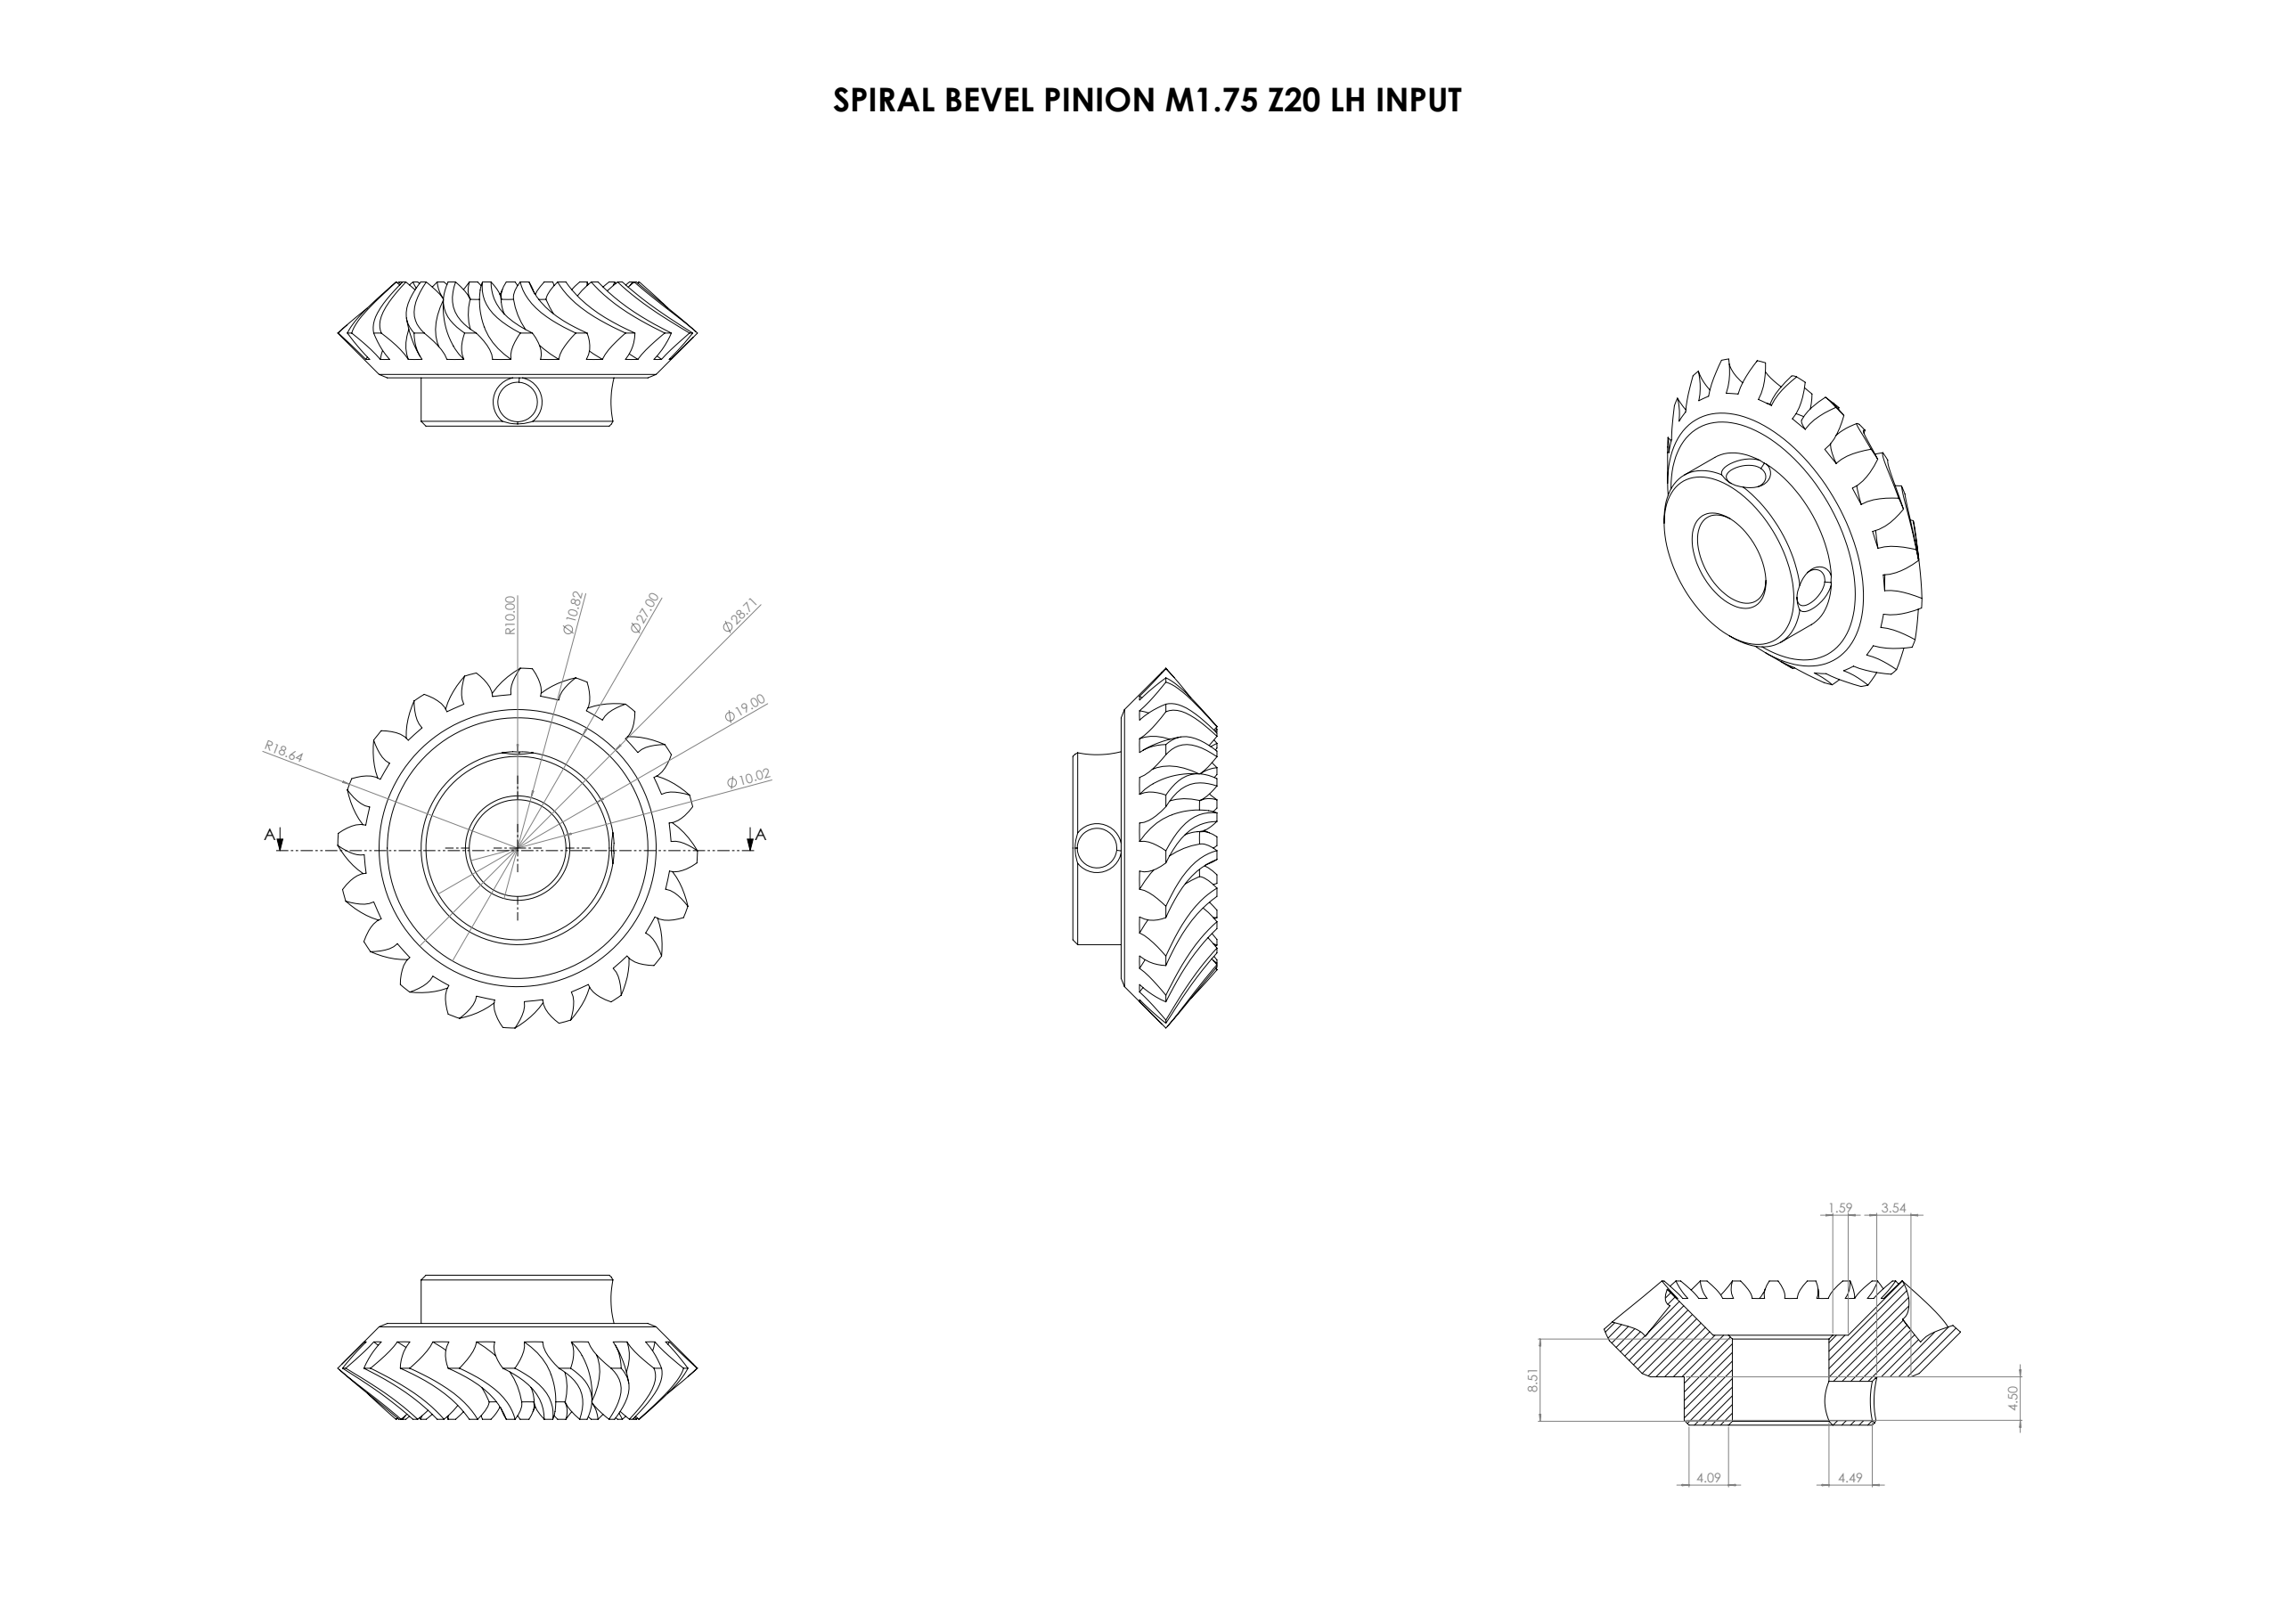
ISO-10303-21;
HEADER;
/* Generated by software containing ST-Developer
 * from STEP Tools, Inc. (www.steptools.com) 
 */

FILE_DESCRIPTION(
/* description */ (''),
/* implementation_level */ '2;1');

FILE_NAME(
/* name */ 
'03_Spiral_Bevel_Pinion_m1.75_z20_LH_Input.step',
/* time_stamp */ '2026-10-22T00:21:42-07:00',
/* author */ (''),
/* organization */ (''),
/* preprocessor_version */ 'ST-DEVELOPER v20.2',
/* originating_system */ 'Autodesk Translation Framework v15.15.0.0',
/* authorisation */ '');

FILE_SCHEMA (('AUTOMOTIVE_DESIGN { 1 0 10303 214 3 1 1 }'));
ENDSEC;

DATA;
#10=MECHANICAL_DESIGN_GEOMETRIC_PRESENTATION_REPRESENTATION('',(#206),#31638);
#184=SHAPE_REPRESENTATION_RELATIONSHIP('SRR','None',#31706,#195);
#195=ADVANCED_BREP_SHAPE_REPRESENTATION('',(#217),#31628);
#206=STYLED_ITEM('',(#31823),#217);
#217=MANIFOLD_SOLID_BREP('Spiral bevel gear',#12481);
#263=CYLINDRICAL_SURFACE('',#12805,1.);
#264=CYLINDRICAL_SURFACE('',#12808,1.);
#265=CYLINDRICAL_SURFACE('',#12810,0.205);
#266=CYLINDRICAL_SURFACE('',#12811,0.205);
#267=CYLINDRICAL_SURFACE('',#12860,0.501);
#376=CONICAL_SURFACE('',#12777,1.39267766952966,1.17809724509617);
#377=CONICAL_SURFACE('',#12781,1.63192209588552,0.785398163397448);
#378=CONICAL_SURFACE('',#12812,0.975,0.785398163397446);
#379=CONICAL_SURFACE('',#12814,1.56260147929642,0.850360450324169);
#380=CONICAL_SURFACE('',#12816,1.56260147929642,0.850360450324169);
#381=CONICAL_SURFACE('',#12818,1.56260147929642,0.850360450324169);
#382=CONICAL_SURFACE('',#12820,1.56260147929642,0.850360450324169);
#383=CONICAL_SURFACE('',#12822,1.56260147929642,0.850360450324169);
#384=CONICAL_SURFACE('',#12824,1.56260147929642,0.850360450324169);
#385=CONICAL_SURFACE('',#12826,1.56260147929642,0.850360450324169);
#386=CONICAL_SURFACE('',#12828,1.56260147929642,0.850360450324169);
#387=CONICAL_SURFACE('',#12830,1.56260147929642,0.850360450324169);
#388=CONICAL_SURFACE('',#12832,1.56260147929642,0.850360450324169);
#389=CONICAL_SURFACE('',#12834,1.56260147929642,0.850360450324169);
#390=CONICAL_SURFACE('',#12836,1.56260147929642,0.850360450324169);
#391=CONICAL_SURFACE('',#12838,1.56260147929642,0.850360450324169);
#392=CONICAL_SURFACE('',#12840,1.56260147929642,0.850360450324169);
#393=CONICAL_SURFACE('',#12842,1.56260147929642,0.850360450324169);
#394=CONICAL_SURFACE('',#12844,1.56260147929642,0.850360450324169);
#395=CONICAL_SURFACE('',#12846,1.56260147929642,0.850360450324169);
#396=CONICAL_SURFACE('',#12848,1.56260147929642,0.850360450324169);
#397=CONICAL_SURFACE('',#12850,1.56260147929642,0.850360450324169);
#398=CONICAL_SURFACE('',#12852,0.980679383410898,0.785398163397448);
#399=CONICAL_SURFACE('',#12855,1.56260147929642,0.850360450324169);
#400=CONICAL_SURFACE('',#12858,0.521,0.785398163397448);
#401=CONICAL_SURFACE('',#12862,0.521,0.785398163397451);
#501=B_SPLINE_CURVE_WITH_KNOTS('',3,(#17566,#17567,#17568,#17569,#17570,
#17571,#17572,#17573),.UNSPECIFIED.,.F.,.F.,(4,2,2,4),(0.149692773523897,
0.272438948836772,0.38754999579811,0.470116529869204),.UNSPECIFIED.);
#502=B_SPLINE_CURVE_WITH_KNOTS('',3,(#17575,#17576,#17577,#17578,#17579,
#17580,#17581),.UNSPECIFIED.,.F.,.F.,(4,3,4),(0.,0.0936389480740432,0.191756090575866),
 .UNSPECIFIED.);
#503=B_SPLINE_CURVE_WITH_KNOTS('',3,(#17583,#17584,#17585,#17586,#17587,
#17588),.UNSPECIFIED.,.F.,.F.,(4,2,4),(0.,0.200149552465016,0.391670798584888),
 .UNSPECIFIED.);
#504=B_SPLINE_CURVE_WITH_KNOTS('',3,(#17592,#17593,#17594,#17595,#17596,
#17597,#17598,#17599),.UNSPECIFIED.,.F.,.F.,(4,2,2,4),(0.0766926694683487,
0.272438948824957,0.387549995788498,0.470116529871579),.UNSPECIFIED.);
#505=B_SPLINE_CURVE_WITH_KNOTS('',3,(#17601,#17602,#17603,#17604,#17605,
#17606,#17607),.UNSPECIFIED.,.F.,.F.,(4,3,4),(0.,0.0936389480740869,0.191756090576058),
 .UNSPECIFIED.);
#506=B_SPLINE_CURVE_WITH_KNOTS('',3,(#17609,#17610,#17611,#17612,#17613,
#17614),.UNSPECIFIED.,.F.,.F.,(4,2,4),(0.,0.200149552461942,0.391670798543005),
 .UNSPECIFIED.);
#507=B_SPLINE_CURVE_WITH_KNOTS('',3,(#17618,#17619,#17620,#17621,#17622,
#17623,#17624,#17625),.UNSPECIFIED.,.F.,.F.,(4,2,2,4),(0.07669266946791,
0.272438948814009,0.387549995787584,0.470116529878316),.UNSPECIFIED.);
#508=B_SPLINE_CURVE_WITH_KNOTS('',3,(#17627,#17628,#17629,#17630,#17631,
#17632,#17633),.UNSPECIFIED.,.F.,.F.,(4,3,4),(0.,0.093638948074052,0.191756090575907),
 .UNSPECIFIED.);
#509=B_SPLINE_CURVE_WITH_KNOTS('',3,(#17635,#17636,#17637,#17638,#17639,
#17640),.UNSPECIFIED.,.F.,.F.,(4,2,4),(0.,0.200149552452443,0.391670798540186),
 .UNSPECIFIED.);
#510=B_SPLINE_CURVE_WITH_KNOTS('',3,(#17644,#17645,#17646,#17647,#17648,
#17649,#17650,#17651),.UNSPECIFIED.,.F.,.F.,(4,2,2,4),(0.0766926694699025,
0.27243894883796,0.387549995810096,0.470116529899442),.UNSPECIFIED.);
#511=B_SPLINE_CURVE_WITH_KNOTS('',3,(#17653,#17654,#17655,#17656,#17657,
#17658,#17659),.UNSPECIFIED.,.F.,.F.,(4,3,4),(0.,0.0936389480740974,0.191756090576102),
 .UNSPECIFIED.);
#512=B_SPLINE_CURVE_WITH_KNOTS('',3,(#17661,#17662,#17663,#17664,#17665,
#17666),.UNSPECIFIED.,.F.,.F.,(4,2,4),(0.,0.200149552471508,0.391670798610117),
 .UNSPECIFIED.);
#513=B_SPLINE_CURVE_WITH_KNOTS('',3,(#17670,#17671,#17672,#17673,#17674,
#17675,#17676,#17677),.UNSPECIFIED.,.F.,.F.,(4,2,2,4),(0.0766926694689824,
0.272438948828123,0.387549995794212,0.47011652987127),.UNSPECIFIED.);
#514=B_SPLINE_CURVE_WITH_KNOTS('',3,(#17679,#17680,#17681,#17682,#17683,
#17684,#17685),.UNSPECIFIED.,.F.,.F.,(4,3,4),(0.,0.0936389480740665,0.191756090575991),
 .UNSPECIFIED.);
#515=B_SPLINE_CURVE_WITH_KNOTS('',3,(#17687,#17688,#17689,#17690,#17691,
#17692),.UNSPECIFIED.,.F.,.F.,(4,2,4),(0.,0.200149552469487,0.327652992715533),
 .UNSPECIFIED.);
#516=B_SPLINE_CURVE_WITH_KNOTS('',3,(#17696,#17697,#17698,#17699,#17700,
#17701,#17702,#17703),.UNSPECIFIED.,.F.,.F.,(4,2,2,4),(0.0766926694695153,
0.272438948836664,0.387549995798075,0.47011652986564),.UNSPECIFIED.);
#517=B_SPLINE_CURVE_WITH_KNOTS('',3,(#17705,#17706,#17707,#17708,#17709,
#17710,#17711),.UNSPECIFIED.,.F.,.F.,(4,3,4),(0.,0.0936389480740678,0.191756090575965),
 .UNSPECIFIED.);
#518=B_SPLINE_CURVE_WITH_KNOTS('',3,(#17713,#17714,#17715,#17716,#17717,
#17718),.UNSPECIFIED.,.F.,.F.,(4,2,4),(0.,0.200149552470465,0.391670798620175),
 .UNSPECIFIED.);
#519=B_SPLINE_CURVE_WITH_KNOTS('',3,(#17722,#17723,#17724,#17725,#17726,
#17727,#17728,#17729),.UNSPECIFIED.,.F.,.F.,(4,2,2,4),(0.0766926694689144,
0.272438948826603,0.387549995797168,0.47011652988698),.UNSPECIFIED.);
#520=B_SPLINE_CURVE_WITH_KNOTS('',3,(#17731,#17732,#17733,#17734,#17735,
#17736,#17737),.UNSPECIFIED.,.F.,.F.,(4,3,4),(0.,0.0936389480740579,0.191756090575915),
 .UNSPECIFIED.);
#521=B_SPLINE_CURVE_WITH_KNOTS('',3,(#17739,#17740,#17741,#17742,#17743,
#17744),.UNSPECIFIED.,.F.,.F.,(4,2,4),(0.,0.200149552468106,0.391670798588367),
 .UNSPECIFIED.);
#522=B_SPLINE_CURVE_WITH_KNOTS('',3,(#17748,#17749,#17750,#17751,#17752,
#17753,#17754,#17755),.UNSPECIFIED.,.F.,.F.,(4,2,2,4),(0.0766926694722585,
0.272438948867033,0.387549995827054,0.470116529890559),.UNSPECIFIED.);
#523=B_SPLINE_CURVE_WITH_KNOTS('',3,(#17757,#17758,#17759,#17760,#17761,
#17762,#17763),.UNSPECIFIED.,.F.,.F.,(4,3,4),(0.,0.0936389480740453,0.191756090575874),
 .UNSPECIFIED.);
#524=B_SPLINE_CURVE_WITH_KNOTS('',3,(#17765,#17766,#17767,#17768,#17769,
#17770),.UNSPECIFIED.,.F.,.F.,(4,2,4),(0.,0.200149552459509,0.391670798578034),
 .UNSPECIFIED.);
#525=B_SPLINE_CURVE_WITH_KNOTS('',3,(#17774,#17775,#17776,#17777,#17778,
#17779,#17780,#17781),.UNSPECIFIED.,.F.,.F.,(4,2,2,4),(0.0766926694700454,
0.272438948841727,0.387549995804977,0.470116529879896),.UNSPECIFIED.);
#526=B_SPLINE_CURVE_WITH_KNOTS('',3,(#17783,#17784,#17785,#17786,#17787,
#17788,#17789),.UNSPECIFIED.,.F.,.F.,(4,3,4),(0.,0.0936389480740846,0.191756090576072),
 .UNSPECIFIED.);
#527=B_SPLINE_CURVE_WITH_KNOTS('',3,(#17791,#17792,#17793,#17794,#17795,
#17796),.UNSPECIFIED.,.F.,.F.,(4,2,4),(0.,0.200149552458071,0.391670798531918),
 .UNSPECIFIED.);
#528=B_SPLINE_CURVE_WITH_KNOTS('',3,(#17800,#17801,#17802,#17803,#17804,
#17805,#17806,#17807),.UNSPECIFIED.,.F.,.F.,(4,2,2,4),(0.0766926694689764,
0.272438948828007,0.387549995794164,0.470116529870617),.UNSPECIFIED.);
#529=B_SPLINE_CURVE_WITH_KNOTS('',3,(#17809,#17810,#17811,#17812,#17813,
#17814,#17815),.UNSPECIFIED.,.F.,.F.,(4,3,4),(0.,0.0936389480741051,0.191756090576146),
 .UNSPECIFIED.);
#530=B_SPLINE_CURVE_WITH_KNOTS('',3,(#17817,#17818,#17819,#17820,#17821,
#17822),.UNSPECIFIED.,.F.,.F.,(4,2,4),(0.,0.200149552457873,0.327652992693914),
 .UNSPECIFIED.);
#531=B_SPLINE_CURVE_WITH_KNOTS('',3,(#17826,#17827,#17828,#17829,#17830,
#17831,#17832,#17833),.UNSPECIFIED.,.F.,.F.,(4,2,2,4),(0.0766926694699692,
0.272438948839556,0.387549995809595,0.470116529895468),.UNSPECIFIED.);
#532=B_SPLINE_CURVE_WITH_KNOTS('',3,(#17835,#17836,#17837,#17838,#17839,
#17840,#17841),.UNSPECIFIED.,.F.,.F.,(4,3,4),(0.,0.0936389480740616,0.191756090575948),
 .UNSPECIFIED.);
#533=B_SPLINE_CURVE_WITH_KNOTS('',3,(#17843,#17844,#17845,#17846,#17847,
#17848),.UNSPECIFIED.,.F.,.F.,(4,2,4),(0.,0.200149552455358,0.391670798525636),
 .UNSPECIFIED.);
#534=B_SPLINE_CURVE_WITH_KNOTS('',3,(#17852,#17853,#17854,#17855,#17856,
#17857,#17858,#17859),.UNSPECIFIED.,.F.,.F.,(4,2,2,4),(0.0766926694698568,
0.272438948838172,0.387549995805395,0.470116529884337),.UNSPECIFIED.);
#535=B_SPLINE_CURVE_WITH_KNOTS('',3,(#17861,#17862,#17863,#17864,#17865,
#17866,#17867),.UNSPECIFIED.,.F.,.F.,(4,3,4),(0.,0.0936389480740228,0.191756090575811),
 .UNSPECIFIED.);
#536=B_SPLINE_CURVE_WITH_KNOTS('',3,(#17869,#17870,#17871,#17872,#17873,
#17874),.UNSPECIFIED.,.F.,.F.,(4,2,4),(0.,0.200149552470612,0.391670798618823),
 .UNSPECIFIED.);
#537=B_SPLINE_CURVE_WITH_KNOTS('',3,(#17878,#17879,#17880,#17881,#17882,
#17883,#17884,#17885),.UNSPECIFIED.,.F.,.F.,(4,2,2,4),(0.0766926694692372,
0.272438948831663,0.387549995799224,0.470116529873121),.UNSPECIFIED.);
#538=B_SPLINE_CURVE_WITH_KNOTS('',3,(#17887,#17888,#17889,#17890,#17891,
#17892,#17893),.UNSPECIFIED.,.F.,.F.,(4,3,4),(0.,0.0936389480740782,0.19175609057602),
 .UNSPECIFIED.);
#539=B_SPLINE_CURVE_WITH_KNOTS('',3,(#17895,#17896,#17897,#17898,#17899,
#17900),.UNSPECIFIED.,.F.,.F.,(4,2,4),(0.,0.200149552459575,0.391670798562508),
 .UNSPECIFIED.);
#540=B_SPLINE_CURVE_WITH_KNOTS('',3,(#17904,#17905,#17906,#17907,#17908,
#17909,#17910,#17911),.UNSPECIFIED.,.F.,.F.,(4,2,2,4),(0.0766926694691861,
0.272438948833637,0.387549995804666,0.470116529896578),.UNSPECIFIED.);
#541=B_SPLINE_CURVE_WITH_KNOTS('',3,(#17913,#17914,#17915,#17916,#17917,
#17918,#17919),.UNSPECIFIED.,.F.,.F.,(4,3,4),(0.,0.093638948074071,0.191756090576001),
 .UNSPECIFIED.);
#542=B_SPLINE_CURVE_WITH_KNOTS('',3,(#17921,#17922,#17923,#17924,#17925,
#17926),.UNSPECIFIED.,.F.,.F.,(4,2,4),(0.,0.20014955246592,0.39167079859368),
 .UNSPECIFIED.);
#543=B_SPLINE_CURVE_WITH_KNOTS('',3,(#17930,#17931,#17932,#17933,#17934,
#17935,#17936,#17937),.UNSPECIFIED.,.F.,.F.,(4,2,2,4),(0.0766926694700761,
0.27243894884306,0.387549995806336,0.470116529880931),.UNSPECIFIED.);
#544=B_SPLINE_CURVE_WITH_KNOTS('',3,(#17939,#17940,#17941,#17942,#17943,
#17944,#17945),.UNSPECIFIED.,.F.,.F.,(4,3,4),(0.,0.0936389480740579,0.191756090575929),
 .UNSPECIFIED.);
#545=B_SPLINE_CURVE_WITH_KNOTS('',3,(#17947,#17948,#17949,#17950,#17951,
#17952),.UNSPECIFIED.,.F.,.F.,(4,2,4),(0.,0.200149552465185,0.327652992740583),
 .UNSPECIFIED.);
#546=B_SPLINE_CURVE_WITH_KNOTS('',3,(#17956,#17957,#17958,#17959,#17960,
#17961,#17962,#17963),.UNSPECIFIED.,.F.,.F.,(4,2,2,4),(0.0766926694694027,
0.272438948835416,0.38754999579658,0.470116529865663),.UNSPECIFIED.);
#547=B_SPLINE_CURVE_WITH_KNOTS('',3,(#17965,#17966,#17967,#17968,#17969,
#17970,#17971),.UNSPECIFIED.,.F.,.F.,(4,3,4),(0.,0.0936389480740775,0.191756090576017),
 .UNSPECIFIED.);
#548=B_SPLINE_CURVE_WITH_KNOTS('',3,(#17973,#17974,#17975,#17976,#17977,
#17978),.UNSPECIFIED.,.F.,.F.,(4,2,4),(0.,0.200149552466382,0.391670798591391),
 .UNSPECIFIED.);
#549=B_SPLINE_CURVE_WITH_KNOTS('',3,(#17982,#17983,#17984,#17985,#17986,
#17987,#17988,#17989),.UNSPECIFIED.,.F.,.F.,(4,2,2,4),(0.0766926694683472,
0.272438948824933,0.387549995788448,0.470116529871442),.UNSPECIFIED.);
#550=B_SPLINE_CURVE_WITH_KNOTS('',3,(#17991,#17992,#17993,#17994,#17995,
#17996,#17997),.UNSPECIFIED.,.F.,.F.,(4,3,4),(0.,0.0936389480740692,0.19175609057597),
 .UNSPECIFIED.);
#551=B_SPLINE_CURVE_WITH_KNOTS('',3,(#17999,#18000,#18001,#18002,#18003,
#18004),.UNSPECIFIED.,.F.,.F.,(4,2,4),(0.,0.200149552469509,0.391670798593535),
 .UNSPECIFIED.);
#552=B_SPLINE_CURVE_WITH_KNOTS('',3,(#18008,#18009,#18010,#18011,#18012,
#18013,#18014,#18015),.UNSPECIFIED.,.F.,.F.,(4,2,2,4),(0.0766926694679092,
0.272438948814003,0.387549995787569,0.470116529878258),.UNSPECIFIED.);
#553=B_SPLINE_CURVE_WITH_KNOTS('',3,(#18017,#18018,#18019,#18020,#18021,
#18022,#18023),.UNSPECIFIED.,.F.,.F.,(4,3,4),(0.,0.093638948074058,0.191756090575958),
 .UNSPECIFIED.);
#554=B_SPLINE_CURVE_WITH_KNOTS('',3,(#18025,#18026,#18027,#18028,#18029,
#18030),.UNSPECIFIED.,.F.,.F.,(4,2,4),(0.,0.200149552458024,0.391670798575916),
 .UNSPECIFIED.);
#555=B_SPLINE_CURVE_WITH_KNOTS('',3,(#18034,#18035,#18036,#18037,#18038,
#18039,#18040,#18041),.UNSPECIFIED.,.F.,.F.,(4,2,2,4),(0.076692669469278,
0.272438948829378,0.387549995792969,0.47011652986107),.UNSPECIFIED.);
#556=B_SPLINE_CURVE_WITH_KNOTS('',3,(#18043,#18044,#18045,#18046,#18047,
#18048,#18049),.UNSPECIFIED.,.F.,.F.,(4,3,4),(0.,0.093638948074072,0.191756090575973),
 .UNSPECIFIED.);
#557=B_SPLINE_CURVE_WITH_KNOTS('',3,(#18051,#18052,#18053,#18054,#18055,
#18056),.UNSPECIFIED.,.F.,.F.,(4,2,4),(0.,0.200149552458622,0.391670798526984),
 .UNSPECIFIED.);
#558=B_SPLINE_CURVE_WITH_KNOTS('',3,(#18060,#18061,#18062,#18063,#18064,
#18065,#18066,#18067),.UNSPECIFIED.,.F.,.F.,(4,2,2,4),(0.0766926694689178,
0.272438948827195,0.387549995791794,0.470116529864375),.UNSPECIFIED.);
#559=B_SPLINE_CURVE_WITH_KNOTS('',3,(#18069,#18070,#18071,#18072,#18073,
#18074,#18075),.UNSPECIFIED.,.F.,.F.,(4,3,4),(0.,0.0936389480740925,0.191756090576061),
 .UNSPECIFIED.);
#560=B_SPLINE_CURVE_WITH_KNOTS('',3,(#18077,#18078,#18079,#18080,#18081,
#18082),.UNSPECIFIED.,.F.,.F.,(4,2,4),(0.,0.200149552462937,0.327652992716261),
 .UNSPECIFIED.);
#561=B_SPLINE_CURVE_WITH_KNOTS('',3,(#18085,#18086,#18087,#18088),
 .UNSPECIFIED.,.F.,.F.,(4,4),(0.076692669469509,0.149692773523897),
 .UNSPECIFIED.);
#562=B_SPLINE_CURVE_WITH_KNOTS('',3,(#18094,#18095,#18096,#18097,#18098,
#18099,#18100,#18101,#18102,#18103,#18104,#18105,#18106,#18107,#18108,#18109,
#18110,#18111,#18112,#18113,#18114,#18115,#18116,#18117,#18118,#18119,#18120,
#18121,#18122,#18123,#18124,#18125,#18126,#18127,#18128,#18129,#18130),
 .UNSPECIFIED.,.F.,.F.,(4,3,3,3,3,3,3,3,3,3,3,3,4),(0.,0.0140126898858465,
0.0198365927950119,0.0393688637311589,0.0455583406050571,0.0493231568139791,
0.0527005792494364,0.0569161964938546,0.0651768568751002,0.0683276956644967,
0.0828398890011837,0.0964479725722503,0.100882854087323),.UNSPECIFIED.);
#563=B_SPLINE_CURVE_WITH_KNOTS('',3,(#18133,#18134,#18135,#18136,#18137,
#18138,#18139,#18140,#18141,#18142,#18143,#18144,#18145,#18146,#18147,#18148,
#18149,#18150,#18151,#18152,#18153,#18154,#18155,#18156,#18157,#18158,#18159,
#18160,#18161,#18162,#18163,#18164,#18165,#18166),.UNSPECIFIED.,.F.,.F.,
(4,3,3,3,3,3,3,3,3,3,3,4),(0.,0.0110116267986798,0.0198365927950272,0.0393688637311641,
0.0455583406049715,0.0493231568143408,0.0527005792502689,0.056916196494854,
0.0651768568763584,0.0788461297337949,0.0828398890027903,0.100882854089343),
 .UNSPECIFIED.);
#564=B_SPLINE_CURVE_WITH_KNOTS('',3,(#18284,#18285,#18286,#18287,#18288,
#18289,#18290,#18291,#18292,#18293,#18294,#18295,#18296,#18297),
 .UNSPECIFIED.,.F.,.F.,(4,1,1,1,1,1,1,1,1,2,4),(-0.889886066635509,-0.843971490026765,
-0.78979558357151,-0.749163653730069,-0.681443770661001,-0.654355817433373,
-0.627267864205746,-0.600179910978118,-0.573091957750491,-0.464740144839981,
-0.44137654239973),.UNSPECIFIED.);
#565=B_SPLINE_CURVE_WITH_KNOTS('',3,(#18299,#18300,#18301,#18302,#18303,
#18304,#18305,#18306,#18307,#18308,#18309,#18310),.UNSPECIFIED.,.F.,.F.,
(4,2,2,2,2,4),(0.,0.0358257028990328,0.131952299625094,0.148884451735932,
0.157379698574708,0.16223106694039),.UNSPECIFIED.);
#566=B_SPLINE_CURVE_WITH_KNOTS('',3,(#18312,#18313,#18314,#18315),
 .UNSPECIFIED.,.F.,.F.,(4,4),(0.549999999941368,1.),.UNSPECIFIED.);
#567=B_SPLINE_CURVE_WITH_KNOTS('',3,(#18317,#18318,#18319,#18320,#18321,
#18322,#18323,#18324,#18325,#18326,#18327,#18328,#18329,#18330,#18331,#18332),
 .UNSPECIFIED.,.F.,.F.,(4,1,2,1,1,1,1,1,1,1,1,1,4),(0.310721506882948,0.387730825861464,
0.464740144839981,0.573091957750491,0.600179910978118,0.627267864205746,
0.654355817433373,0.681443770661001,0.749163653730069,0.78979558357151,
0.843971490026765,0.89814739648202,0.929489890414014),.UNSPECIFIED.);
#568=B_SPLINE_CURVE_WITH_KNOTS('',3,(#18333,#18334,#18335,#18336,#18337,
#18338,#18339,#18340,#18341,#18342,#18343,#18344,#18345,#18346,#18347,#18348,
#18349),.UNSPECIFIED.,.F.,.F.,(4,1,1,1,1,1,1,1,1,1,1,1,1,1,4),(0.929489890414014,
0.952323302937276,1.00649920939253,1.06067511584779,1.11485102230304,1.1690269287583,
1.22320283521355,1.26383476505499,1.33155464812406,1.35864260135169,1.38573055457932,
1.41281850780694,1.43990646103457,1.49408236748983,1.54825827394508),
 .UNSPECIFIED.);
#569=B_SPLINE_CURVE_WITH_KNOTS('',3,(#18351,#18352,#18353,#18354,#18355,
#18356,#18357,#18358,#18359,#18360,#18361,#18362,#18363,#18364),
 .UNSPECIFIED.,.F.,.F.,(4,2,2,2,2,2,4),(0.16223106694039,0.163967550885131,
0.171180716857468,0.182777598096348,0.205784524866042,0.262730804446443,
0.324280670363194),.UNSPECIFIED.);
#570=B_SPLINE_CURVE_WITH_KNOTS('',3,(#18365,#18366,#18367,#18368,#18369,
#18370,#18371,#18372,#18373,#18374,#18375,#18376,#18377,#18378),
 .UNSPECIFIED.,.F.,.F.,(4,1,1,1,1,1,1,1,1,1,1,4),(-1.4176032384283,-1.41281850780694,
-1.38573055457932,-1.35864260135169,-1.33155464812406,-1.26383476505499,
-1.22320283521355,-1.1690269287583,-1.11485102230304,-1.06067511584779,
-1.00649920939253,-0.969093714192518),.UNSPECIFIED.);
#571=B_SPLINE_CURVE_WITH_KNOTS('',3,(#18384,#18385,#18386,#18387,#18388,
#18389,#18390,#18391,#18392,#18393,#18394,#18395),.UNSPECIFIED.,.F.,.F.,
(4,1,1,1,1,1,1,2,4),(-1.50954599357819,-1.43295998077967,-1.38938999215504,
-1.34582000353042,-1.25868002628116,-1.21511003765654,-1.17154004903191,
-1.08440007178266,-1.06103646934241),.UNSPECIFIED.);
#572=B_SPLINE_CURVE_WITH_KNOTS('',3,(#18398,#18399,#18400,#18401,#18402,
#18403,#18404,#18405,#18406,#18407,#18408,#18409,#18410,#18411),
 .UNSPECIFIED.,.F.,.F.,(4,1,1,1,2,2,1,1,1,4),(-2.03726316537097,-2.03275764211163,
-2.01344899085789,-1.93621438584296,-1.85897978082803,-1.78151988977668,
-1.71616490683974,-1.69437991252743,-1.60723993527817,-1.58875364113519),
 .UNSPECIFIED.);
#573=B_SPLINE_CURVE_WITH_KNOTS('',3,(#18417,#18418,#18419,#18420,#18421,
#18422,#18423,#18424,#18425,#18426),.UNSPECIFIED.,.F.,.F.,(4,2,2,2,4),(0.,
0.0782721603764034,0.156544320752807,0.234729089704077,0.312913858655347),
 .UNSPECIFIED.);
#574=B_SPLINE_CURVE_WITH_KNOTS('',3,(#18427,#18428,#18429,#18430,#18431,
#18432,#18433,#18434,#18435,#18436,#18437,#18438,#18439,#18440,#18441,#18442,
#18443,#18444,#18445,#18446,#18447,#18448,#18449,#18450,#18451,#18452),
 .UNSPECIFIED.,.F.,.F.,(4,2,2,2,2,2,2,2,2,2,2,2,4),(0.312913858655347,0.391098627606618,
0.469283396557888,0.547555556934292,0.625827717310695,0.704099877687098,
0.782372038063502,0.860556807014772,0.938741575966043,1.01692634491731,
1.09511111386858,1.17338327424499,1.25165543462139),.UNSPECIFIED.);
#575=B_SPLINE_CURVE_WITH_KNOTS('',3,(#18566,#18567,#18568,#18569,#18570,
#18571,#18572,#18573,#18574,#18575,#18576,#18577),.UNSPECIFIED.,.F.,.F.,
(4,2,2,2,2,4),(0.,0.0358257028990433,0.131952299625135,0.148884451735976,
0.157379698574799,0.162231066940522),.UNSPECIFIED.);
#576=B_SPLINE_CURVE_WITH_KNOTS('',3,(#18579,#18580,#18581,#18582),
 .UNSPECIFIED.,.F.,.F.,(4,4),(0.549999999941368,1.),.UNSPECIFIED.);
#577=B_SPLINE_CURVE_WITH_KNOTS('',3,(#18584,#18585,#18586,#18587,#18588,
#18589,#18590,#18591,#18592,#18593,#18594,#18595,#18596,#18597),
 .UNSPECIFIED.,.F.,.F.,(4,1,2,1,1,1,1,1,1,1,4),(0.930381433825624,1.00739075280414,
1.08440007178266,1.17154004903191,1.21511003765654,1.25868002628116,1.34582000353042,
1.38938999215504,1.43295998077967,1.52009995802892,1.54914981735669),
 .UNSPECIFIED.);
#578=B_SPLINE_CURVE_WITH_KNOTS('',3,(#18598,#18599,#18600,#18601,#18602,
#18603,#18604,#18605,#18606,#18607,#18608,#18609,#18610,#18611,#18612,#18613,
#18614,#18615),.UNSPECIFIED.,.F.,.F.,(4,1,1,1,1,1,2,2,1,1,1,1,1,4),(1.54914981735669,
1.56366994665355,1.58545494096586,1.60723993527817,1.69437991252743,1.71616490683974,
1.78151988977668,1.85897978082803,1.93621438584296,2.01344899085789,2.03275764211163,
2.05206629336536,2.09068359587282,2.16791820088776),.UNSPECIFIED.);
#579=B_SPLINE_CURVE_WITH_KNOTS('',3,(#18616,#18617,#18618,#18619,#18620,
#18621,#18622,#18623,#18624,#18625,#18626,#18627,#18628,#18629),
 .UNSPECIFIED.,.F.,.F.,(4,2,2,2,2,2,4),(0.162231066940522,0.163967550885278,
0.171180716857662,0.182777598096494,0.205784524865831,0.262730804445425,
0.324280670361326),.UNSPECIFIED.);
#580=B_SPLINE_CURVE_WITH_KNOTS('',3,(#18633,#18634,#18635,#18636,#18637,
#18638,#18639,#18640,#18641,#18642,#18643,#18644,#18645,#18646,#18647,#18648,
#18649,#18650,#18651,#18652,#18653,#18654,#18655,#18656,#18657,#18658),
 .UNSPECIFIED.,.F.,.F.,(4,2,2,2,2,2,2,2,2,2,2,2,4),(0.,0.0782721603764034,
0.156544320752807,0.234729089704077,0.312913858655348,0.391098627606618,
0.469283396557888,0.547555556934292,0.625827717310695,0.704099877687099,
0.782372038063502,0.860556807014772,0.938741575966043),.UNSPECIFIED.);
#581=B_SPLINE_CURVE_WITH_KNOTS('',3,(#18659,#18660,#18661,#18662,#18663,
#18664,#18665,#18666,#18667,#18668),.UNSPECIFIED.,.F.,.F.,(4,2,2,2,4),(0.938741575966043,
1.01692634491731,1.09511111386858,1.17338327424499,1.25165543462139),
 .UNSPECIFIED.);
#582=B_SPLINE_CURVE_WITH_KNOTS('',3,(#18700,#18701,#18702,#18703,#18704,
#18705),.UNSPECIFIED.,.F.,.F.,(4,2,4),(0.,0.138460176945389,0.254919406868435),
 .UNSPECIFIED.);
#583=B_SPLINE_CURVE_WITH_KNOTS('',3,(#18706,#18707,#18708,#18709,#18710,
#18711),.UNSPECIFIED.,.F.,.F.,(4,2,4),(0.0638119305867456,0.434740434623819,
0.895232561311265),.UNSPECIFIED.);
#584=B_SPLINE_CURVE_WITH_KNOTS('',3,(#18712,#18713,#18714,#18715,#18716,
#18717,#18718,#18719),.UNSPECIFIED.,.F.,.F.,(4,2,2,4),(0.0746811865707125,
0.397508022614213,0.744535688298142,1.03619555646955),.UNSPECIFIED.);
#585=B_SPLINE_CURVE_WITH_KNOTS('',3,(#18746,#18747,#18748,#18749,#18750,
#18751,#18752,#18753),.UNSPECIFIED.,.F.,.F.,(4,2,2,4),(0.0544345524991837,
0.140376841744982,0.193303927754724,0.23329596220082),.UNSPECIFIED.);
#586=B_SPLINE_CURVE_WITH_KNOTS('',3,(#18754,#18755,#18756,#18757,#18758,
#18759,#18760,#18761),.UNSPECIFIED.,.F.,.F.,(4,2,2,4),(0.15440517711793,
0.43827181462838,0.790258491635714,1.12994605591353),.UNSPECIFIED.);
#587=B_SPLINE_CURVE_WITH_KNOTS('',3,(#18762,#18763,#18764,#18765,#18766,
#18767),.UNSPECIFIED.,.F.,.F.,(4,2,4),(0.0638119305867456,0.434740434623819,
0.895232561311264),.UNSPECIFIED.);
#588=B_SPLINE_CURVE_WITH_KNOTS('',3,(#18784,#18785,#18786,#18787,#18788,
#18789,#18790),.UNSPECIFIED.,.F.,.F.,(4,3,4),(0.,0.0653793053833038,0.130355487793338),
 .UNSPECIFIED.);
#589=B_SPLINE_CURVE_WITH_KNOTS('',3,(#18794,#18795,#18796,#18797,#18798,
#18799,#18800,#18801),.UNSPECIFIED.,.F.,.F.,(4,2,2,4),(0.0746811865707133,
0.397508022614224,0.744535688298146,1.0361955564692),.UNSPECIFIED.);
#590=B_SPLINE_CURVE_WITH_KNOTS('',3,(#18804,#18805,#18806,#18807,#18808,
#18809,#18810,#18811),.UNSPECIFIED.,.F.,.F.,(4,2,2,4),(0.15440517711793,
0.438271814628377,0.790258491635718,1.12994605591353),.UNSPECIFIED.);
#591=B_SPLINE_CURVE_WITH_KNOTS('',3,(#18839,#18840,#18841,#18842,#18843,
#18844),.UNSPECIFIED.,.F.,.F.,(4,2,4),(0.,0.138460176942891,0.254919406877601),
 .UNSPECIFIED.);
#592=B_SPLINE_CURVE_WITH_KNOTS('',3,(#18845,#18846,#18847,#18848,#18849,
#18850),.UNSPECIFIED.,.F.,.F.,(4,2,4),(0.0638119305867455,0.434740434623819,
0.895232561311264),.UNSPECIFIED.);
#593=B_SPLINE_CURVE_WITH_KNOTS('',3,(#18851,#18852,#18853,#18854,#18855,
#18856,#18857,#18858),.UNSPECIFIED.,.F.,.F.,(4,2,2,4),(0.0746811865707128,
0.397508022614225,0.744535688298148,1.03619555646854),.UNSPECIFIED.);
#594=B_SPLINE_CURVE_WITH_KNOTS('',3,(#18884,#18885,#18886,#18887,#18888,
#18889,#18890,#18891),.UNSPECIFIED.,.F.,.F.,(4,2,2,4),(0.0544345524999985,
0.140376841748909,0.193303927764524,0.233295962216222),.UNSPECIFIED.);
#595=B_SPLINE_CURVE_WITH_KNOTS('',3,(#18892,#18893,#18894,#18895,#18896,
#18897),.UNSPECIFIED.,.F.,.F.,(4,2,4),(0.0638119305867455,0.434740434623819,
0.895232561311264),.UNSPECIFIED.);
#596=B_SPLINE_CURVE_WITH_KNOTS('',3,(#18914,#18915,#18916,#18917,#18918,
#18919,#18920),.UNSPECIFIED.,.F.,.F.,(4,3,4),(0.,0.0653793053833002,0.130355487793372),
 .UNSPECIFIED.);
#597=B_SPLINE_CURVE_WITH_KNOTS('',3,(#18923,#18924,#18925,#18926,#18927,
#18928,#18929,#18930),.UNSPECIFIED.,.F.,.F.,(4,2,2,4),(0.154405177117932,
0.438271814628394,0.790258491635738,1.12994605591355),.UNSPECIFIED.);
#598=B_SPLINE_CURVE_WITH_KNOTS('',3,(#18958,#18959,#18960,#18961,#18962,
#18963),.UNSPECIFIED.,.F.,.F.,(4,2,4),(0.,0.138460176943918,0.254919406860805),
 .UNSPECIFIED.);
#599=B_SPLINE_CURVE_WITH_KNOTS('',3,(#18964,#18965,#18966,#18967,#18968,
#18969),.UNSPECIFIED.,.F.,.F.,(4,2,4),(0.0638119305867456,0.434740434623819,
0.895232561311265),.UNSPECIFIED.);
#600=B_SPLINE_CURVE_WITH_KNOTS('',3,(#18970,#18971,#18972,#18973,#18974,
#18975,#18976,#18977),.UNSPECIFIED.,.F.,.F.,(4,2,2,4),(0.0746811865707128,
0.397508022614222,0.744535688298131,1.03619555646937),.UNSPECIFIED.);
#601=B_SPLINE_CURVE_WITH_KNOTS('',3,(#19003,#19004,#19005,#19006,#19007,
#19008,#19009,#19010),.UNSPECIFIED.,.F.,.F.,(4,2,2,4),(0.0544345524991458,
0.140376841744735,0.193303927754458,0.233295962201587),.UNSPECIFIED.);
#602=B_SPLINE_CURVE_WITH_KNOTS('',3,(#19011,#19012,#19013,#19014,#19015,
#19016),.UNSPECIFIED.,.F.,.F.,(4,2,4),(0.0638119305867456,0.434740434623819,
0.895232561311265),.UNSPECIFIED.);
#603=B_SPLINE_CURVE_WITH_KNOTS('',3,(#19033,#19034,#19035,#19036,#19037,
#19038,#19039),.UNSPECIFIED.,.F.,.F.,(4,3,4),(0.,0.0653793053832705,0.130355487793285),
 .UNSPECIFIED.);
#604=B_SPLINE_CURVE_WITH_KNOTS('',3,(#19042,#19043,#19044,#19045,#19046,
#19047,#19048,#19049),.UNSPECIFIED.,.F.,.F.,(4,2,2,4),(0.15440517711793,
0.438271814628378,0.790258491635719,1.12994605591353),.UNSPECIFIED.);
#605=B_SPLINE_CURVE_WITH_KNOTS('',3,(#19077,#19078,#19079,#19080,#19081,
#19082),.UNSPECIFIED.,.F.,.F.,(4,2,4),(0.,0.138460176945285,0.254919406866285),
 .UNSPECIFIED.);
#606=B_SPLINE_CURVE_WITH_KNOTS('',3,(#19083,#19084,#19085,#19086,#19087,
#19088),.UNSPECIFIED.,.F.,.F.,(4,2,4),(0.0638119305867456,0.434740434623819,
0.895232561311265),.UNSPECIFIED.);
#607=B_SPLINE_CURVE_WITH_KNOTS('',3,(#19089,#19090,#19091,#19092,#19093,
#19094,#19095,#19096),.UNSPECIFIED.,.F.,.F.,(4,2,2,4),(0.0746811865707126,
0.397508022614211,0.744535688298121,1.05488349691751),.UNSPECIFIED.);
#608=B_SPLINE_CURVE_WITH_KNOTS('',3,(#19122,#19123,#19124,#19125,#19126,
#19127,#19128,#19129),.UNSPECIFIED.,.F.,.F.,(4,2,2,4),(0.0544345524985586,
0.140376841742248,0.193303927756487,0.233295962206935),.UNSPECIFIED.);
#609=B_SPLINE_CURVE_WITH_KNOTS('',3,(#19130,#19131,#19132,#19133,#19134,
#19135),.UNSPECIFIED.,.F.,.F.,(4,2,4),(0.0638119305867456,0.434740434623819,
0.895232561311265),.UNSPECIFIED.);
#610=B_SPLINE_CURVE_WITH_KNOTS('',3,(#19152,#19153,#19154,#19155,#19156,
#19157,#19158),.UNSPECIFIED.,.F.,.F.,(4,3,4),(0.,0.0653793053832869,0.130355487793285),
 .UNSPECIFIED.);
#611=B_SPLINE_CURVE_WITH_KNOTS('',3,(#19161,#19162,#19163,#19164,#19165,
#19166,#19167,#19168),.UNSPECIFIED.,.F.,.F.,(4,2,2,4),(0.0774162478443013,
0.414979417786432,0.760655521250469,1.05194916247838),.UNSPECIFIED.);
#612=B_SPLINE_CURVE_WITH_KNOTS('',3,(#19196,#19197,#19198,#19199,#19200,
#19201),.UNSPECIFIED.,.F.,.F.,(4,2,4),(0.,0.138460176945226,0.254919406867686),
 .UNSPECIFIED.);
#613=B_SPLINE_CURVE_WITH_KNOTS('',3,(#19202,#19203,#19204,#19205,#19206,
#19207),.UNSPECIFIED.,.F.,.F.,(4,2,4),(0.0638119305867456,0.434740434623819,
0.895232561311265),.UNSPECIFIED.);
#614=B_SPLINE_CURVE_WITH_KNOTS('',3,(#19208,#19209,#19210,#19211,#19212,
#19213,#19214,#19215),.UNSPECIFIED.,.F.,.F.,(4,2,2,4),(0.0746811865707126,
0.397508022614209,0.744535688298118,1.03619555646857),.UNSPECIFIED.);
#615=B_SPLINE_CURVE_WITH_KNOTS('',3,(#19241,#19242,#19243,#19244,#19245,
#19246,#19247,#19248),.UNSPECIFIED.,.F.,.F.,(4,2,2,4),(0.0544345524990915,
0.140376841744593,0.193303927757736,0.233295962205675),.UNSPECIFIED.);
#616=B_SPLINE_CURVE_WITH_KNOTS('',3,(#19249,#19250,#19251,#19252,#19253,
#19254),.UNSPECIFIED.,.F.,.F.,(4,2,4),(0.0638119305867457,0.434740434623819,
0.895232561311264),.UNSPECIFIED.);
#617=B_SPLINE_CURVE_WITH_KNOTS('',3,(#19271,#19272,#19273,#19274,#19275,
#19276,#19277),.UNSPECIFIED.,.F.,.F.,(4,3,4),(0.,0.0653793053833536,0.130355487793441),
 .UNSPECIFIED.);
#618=B_SPLINE_CURVE_WITH_KNOTS('',3,(#19280,#19281,#19282,#19283,#19284,
#19285,#19286,#19287),.UNSPECIFIED.,.F.,.F.,(4,2,2,4),(0.154405177117923,
0.438271814628353,0.790258491635649,1.1299460559134),.UNSPECIFIED.);
#619=B_SPLINE_CURVE_WITH_KNOTS('',3,(#19315,#19316,#19317,#19318,#19319,
#19320),.UNSPECIFIED.,.F.,.F.,(4,2,4),(0.,0.138460176945371,0.254919406866122),
 .UNSPECIFIED.);
#620=B_SPLINE_CURVE_WITH_KNOTS('',3,(#19321,#19322,#19323,#19324,#19325,
#19326),.UNSPECIFIED.,.F.,.F.,(4,2,4),(0.0638119305867456,0.434740434623819,
0.895232561311265),.UNSPECIFIED.);
#621=B_SPLINE_CURVE_WITH_KNOTS('',3,(#19327,#19328,#19329,#19330,#19331,
#19332,#19333,#19334),.UNSPECIFIED.,.F.,.F.,(4,2,2,4),(0.0746811865707114,
0.397508022614213,0.744535688298102,1.03619555646808),.UNSPECIFIED.);
#622=B_SPLINE_CURVE_WITH_KNOTS('',3,(#19360,#19361,#19362,#19363,#19364,
#19365,#19366,#19367),.UNSPECIFIED.,.F.,.F.,(4,2,2,4),(0.0544345524988946,
0.140376841743774,0.193303927754125,0.233295962200619),.UNSPECIFIED.);
#623=B_SPLINE_CURVE_WITH_KNOTS('',3,(#19368,#19369,#19370,#19371,#19372,
#19373),.UNSPECIFIED.,.F.,.F.,(4,2,4),(0.0638119305867456,0.434740434623819,
0.895232561311264),.UNSPECIFIED.);
#624=B_SPLINE_CURVE_WITH_KNOTS('',3,(#19390,#19391,#19392,#19393,#19394,
#19395,#19396),.UNSPECIFIED.,.F.,.F.,(4,3,4),(0.,0.0653793053832619,0.130355487793235),
 .UNSPECIFIED.);
#625=B_SPLINE_CURVE_WITH_KNOTS('',3,(#19399,#19400,#19401,#19402,#19403,
#19404,#19405,#19406),.UNSPECIFIED.,.F.,.F.,(4,2,2,4),(0.154405177117934,
0.4382718146284,0.790258491635752,1.12994605591358),.UNSPECIFIED.);
#626=B_SPLINE_CURVE_WITH_KNOTS('',3,(#19434,#19435,#19436,#19437,#19438,
#19439),.UNSPECIFIED.,.F.,.F.,(4,2,4),(0.,0.138460176943452,0.25491940687479),
 .UNSPECIFIED.);
#627=B_SPLINE_CURVE_WITH_KNOTS('',3,(#19440,#19441,#19442,#19443,#19444,
#19445),.UNSPECIFIED.,.F.,.F.,(4,2,4),(0.0638119305867456,0.434740434623819,
0.895232561311265),.UNSPECIFIED.);
#628=B_SPLINE_CURVE_WITH_KNOTS('',3,(#19446,#19447,#19448,#19449,#19450,
#19451,#19452,#19453),.UNSPECIFIED.,.F.,.F.,(4,2,2,4),(0.0746811865707127,
0.397508022614219,0.744535688298134,1.0361955564692),.UNSPECIFIED.);
#629=B_SPLINE_CURVE_WITH_KNOTS('',3,(#19479,#19480,#19481,#19482,#19483,
#19484,#19485,#19486),.UNSPECIFIED.,.F.,.F.,(4,2,2,4),(0.0544345524985935,
0.140376841742227,0.193303927751676,0.233295962196035),.UNSPECIFIED.);
#630=B_SPLINE_CURVE_WITH_KNOTS('',3,(#19487,#19488,#19489,#19490,#19491,
#19492),.UNSPECIFIED.,.F.,.F.,(4,2,4),(0.0638119305867456,0.434740434623819,
0.895232561311264),.UNSPECIFIED.);
#631=B_SPLINE_CURVE_WITH_KNOTS('',3,(#19509,#19510,#19511,#19512,#19513,
#19514,#19515),.UNSPECIFIED.,.F.,.F.,(4,3,4),(0.,0.0653793053833638,0.130355487793505),
 .UNSPECIFIED.);
#632=B_SPLINE_CURVE_WITH_KNOTS('',3,(#19518,#19519,#19520,#19521,#19522,
#19523,#19524,#19525),.UNSPECIFIED.,.F.,.F.,(4,2,2,4),(0.154405177117939,
0.438271814628415,0.790258491635773,1.12994605591359),.UNSPECIFIED.);
#633=B_SPLINE_CURVE_WITH_KNOTS('',3,(#19553,#19554,#19555,#19556,#19557,
#19558),.UNSPECIFIED.,.F.,.F.,(4,2,4),(0.,0.138460176943768,0.254919406861752),
 .UNSPECIFIED.);
#634=B_SPLINE_CURVE_WITH_KNOTS('',3,(#19559,#19560,#19561,#19562,#19563,
#19564),.UNSPECIFIED.,.F.,.F.,(4,2,4),(0.0638119305867455,0.434740434623819,
0.895232561311264),.UNSPECIFIED.);
#635=B_SPLINE_CURVE_WITH_KNOTS('',3,(#19565,#19566,#19567,#19568,#19569,
#19570,#19571,#19572),.UNSPECIFIED.,.F.,.F.,(4,2,2,4),(0.074681186570713,
0.397508022614234,0.744535688298142,1.03619555646862),.UNSPECIFIED.);
#636=B_SPLINE_CURVE_WITH_KNOTS('',3,(#19598,#19599,#19600,#19601,#19602,
#19603,#19604,#19605),.UNSPECIFIED.,.F.,.F.,(4,2,2,4),(0.0544345524996551,
0.140376841747112,0.193303927760047,0.233295962211347),.UNSPECIFIED.);
#637=B_SPLINE_CURVE_WITH_KNOTS('',3,(#19606,#19607,#19608,#19609,#19610,
#19611),.UNSPECIFIED.,.F.,.F.,(4,2,4),(0.0638119305867455,0.434740434623819,
0.895232561311264),.UNSPECIFIED.);
#638=B_SPLINE_CURVE_WITH_KNOTS('',3,(#19628,#19629,#19630,#19631,#19632,
#19633,#19634),.UNSPECIFIED.,.F.,.F.,(4,3,4),(0.,0.065379305383271,0.130355487793261),
 .UNSPECIFIED.);
#639=B_SPLINE_CURVE_WITH_KNOTS('',3,(#19637,#19638,#19639,#19640,#19641,
#19642,#19643,#19644),.UNSPECIFIED.,.F.,.F.,(4,2,2,4),(0.154405177117931,
0.43827181462838,0.790258491635724,1.12994605591354),.UNSPECIFIED.);
#640=B_SPLINE_CURVE_WITH_KNOTS('',3,(#19672,#19673,#19674,#19675,#19676,
#19677),.UNSPECIFIED.,.F.,.F.,(4,2,4),(0.,0.13846017694485,0.254919406873115),
 .UNSPECIFIED.);
#641=B_SPLINE_CURVE_WITH_KNOTS('',3,(#19678,#19679,#19680,#19681,#19682,
#19683),.UNSPECIFIED.,.F.,.F.,(4,2,4),(0.0638119305867456,0.434740434623819,
0.895232561311265),.UNSPECIFIED.);
#642=B_SPLINE_CURVE_WITH_KNOTS('',3,(#19684,#19685,#19686,#19687,#19688,
#19689,#19690,#19691),.UNSPECIFIED.,.F.,.F.,(4,2,2,4),(0.0746811865707127,
0.397508022614212,0.74453568829812,1.05488349691753),.UNSPECIFIED.);
#643=B_SPLINE_CURVE_WITH_KNOTS('',3,(#19717,#19718,#19719,#19720,#19721,
#19722,#19723,#19724),.UNSPECIFIED.,.F.,.F.,(4,2,2,4),(0.0544345524992758,
0.140376841745509,0.193303927759893,0.233295962209951),.UNSPECIFIED.);
#644=B_SPLINE_CURVE_WITH_KNOTS('',3,(#19725,#19726,#19727,#19728,#19729,
#19730),.UNSPECIFIED.,.F.,.F.,(4,2,4),(0.0638119305867456,0.434740434623819,
0.895232561311265),.UNSPECIFIED.);
#645=B_SPLINE_CURVE_WITH_KNOTS('',3,(#19747,#19748,#19749,#19750,#19751,
#19752,#19753),.UNSPECIFIED.,.F.,.F.,(4,3,4),(0.,0.0653793053833319,0.130355487793411),
 .UNSPECIFIED.);
#646=B_SPLINE_CURVE_WITH_KNOTS('',3,(#19756,#19757,#19758,#19759,#19760,
#19761,#19762,#19763),.UNSPECIFIED.,.F.,.F.,(4,2,2,4),(0.0774162478442982,
0.414979417786394,0.760655521250395,1.05194916247827),.UNSPECIFIED.);
#647=B_SPLINE_CURVE_WITH_KNOTS('',3,(#19791,#19792,#19793,#19794,#19795,
#19796),.UNSPECIFIED.,.F.,.F.,(4,2,4),(0.,0.13846017694524,0.209756131428923),
 .UNSPECIFIED.);
#648=B_SPLINE_CURVE_WITH_KNOTS('',3,(#19797,#19798,#19799,#19800,#19801,
#19802),.UNSPECIFIED.,.F.,.F.,(4,2,4),(0.0638119305867456,0.434740434623819,
0.895232561311265),.UNSPECIFIED.);
#649=B_SPLINE_CURVE_WITH_KNOTS('',3,(#19804,#19805,#19806,#19807,#19808,
#19809,#19810,#19811),.UNSPECIFIED.,.F.,.F.,(4,2,2,4),(0.0746811865707122,
0.397508022614215,0.744535688298118,1.03619555646847),.UNSPECIFIED.);
#650=B_SPLINE_CURVE_WITH_KNOTS('',3,(#19812,#19813,#19814,#19815),
 .UNSPECIFIED.,.F.,.F.,(4,4),(0.209756131428923,0.254919406867736),
 .UNSPECIFIED.);
#651=B_SPLINE_CURVE_WITH_KNOTS('',3,(#19841,#19842,#19843,#19844,#19845,
#19846,#19847,#19848),.UNSPECIFIED.,.F.,.F.,(4,2,2,4),(0.0544345524990686,
0.140376841744483,0.193303927757129,0.233295962204701),.UNSPECIFIED.);
#652=B_SPLINE_CURVE_WITH_KNOTS('',3,(#19849,#19850,#19851,#19852,#19853,
#19854),.UNSPECIFIED.,.F.,.F.,(4,2,4),(0.0638119305867457,0.434740434623819,
0.895232561311264),.UNSPECIFIED.);
#653=B_SPLINE_CURVE_WITH_KNOTS('',3,(#19871,#19872,#19873,#19874,#19875,
#19876,#19877),.UNSPECIFIED.,.F.,.F.,(4,3,4),(0.,0.0653793053833073,0.130355487793357),
 .UNSPECIFIED.);
#654=B_SPLINE_CURVE_WITH_KNOTS('',3,(#19880,#19881,#19882,#19883,#19884,
#19885,#19886,#19887),.UNSPECIFIED.,.F.,.F.,(4,2,2,4),(0.154405177117928,
0.438271814628368,0.790258491635699,1.12994605591349),.UNSPECIFIED.);
#655=B_SPLINE_CURVE_WITH_KNOTS('',3,(#19915,#19916,#19917,#19918,#19919,
#19920),.UNSPECIFIED.,.F.,.F.,(4,2,4),(0.,0.138460176945471,0.254919406864932),
 .UNSPECIFIED.);
#656=B_SPLINE_CURVE_WITH_KNOTS('',3,(#19921,#19922,#19923,#19924,#19925,
#19926),.UNSPECIFIED.,.F.,.F.,(4,2,4),(0.0638119305867457,0.434740434623819,
0.895232561311265),.UNSPECIFIED.);
#657=B_SPLINE_CURVE_WITH_KNOTS('',3,(#19927,#19928,#19929,#19930,#19931,
#19932,#19933,#19934),.UNSPECIFIED.,.F.,.F.,(4,2,2,4),(0.0746811865707118,
0.39750802261421,0.744535688298092,1.03619555646858),.UNSPECIFIED.);
#658=B_SPLINE_CURVE_WITH_KNOTS('',3,(#19960,#19961,#19962,#19963,#19964,
#19965,#19966,#19967),.UNSPECIFIED.,.F.,.F.,(4,2,2,4),(0.0544345524998506,
0.140376841748323,0.193303927766303,0.233295962218452),.UNSPECIFIED.);
#659=B_SPLINE_CURVE_WITH_KNOTS('',3,(#19968,#19969,#19970,#19971,#19972,
#19973),.UNSPECIFIED.,.F.,.F.,(4,2,4),(0.0638119305867456,0.434740434623819,
0.895232561311265),.UNSPECIFIED.);
#660=B_SPLINE_CURVE_WITH_KNOTS('',3,(#19990,#19991,#19992,#19993,#19994,
#19995,#19996),.UNSPECIFIED.,.F.,.F.,(4,3,4),(0.,0.0653793053833078,0.130355487793348),
 .UNSPECIFIED.);
#661=B_SPLINE_CURVE_WITH_KNOTS('',3,(#19999,#20000,#20001,#20002,#20003,
#20004,#20005,#20006),.UNSPECIFIED.,.F.,.F.,(4,2,2,4),(0.154405177117931,
0.438271814628383,0.790258491635722,1.12994605591352),.UNSPECIFIED.);
#662=B_SPLINE_CURVE_WITH_KNOTS('',3,(#20034,#20035,#20036,#20037,#20038,
#20039),.UNSPECIFIED.,.F.,.F.,(4,2,4),(0.,0.138460176943519,0.254919406873928),
 .UNSPECIFIED.);
#663=B_SPLINE_CURVE_WITH_KNOTS('',3,(#20040,#20041,#20042,#20043,#20044,
#20045),.UNSPECIFIED.,.F.,.F.,(4,2,4),(0.0638119305867456,0.434740434623819,
0.895232561311265),.UNSPECIFIED.);
#664=B_SPLINE_CURVE_WITH_KNOTS('',3,(#20046,#20047,#20048,#20049,#20050,
#20051,#20052,#20053),.UNSPECIFIED.,.F.,.F.,(4,2,2,4),(0.0746811865707111,
0.397508022614208,0.744535688298079,1.036195556468),.UNSPECIFIED.);
#665=B_SPLINE_CURVE_WITH_KNOTS('',3,(#20079,#20080,#20081,#20082,#20083,
#20084,#20085,#20086),.UNSPECIFIED.,.F.,.F.,(4,2,2,4),(0.0544345524985954,
0.140376841742234,0.193303927751678,0.233295962196024),.UNSPECIFIED.);
#666=B_SPLINE_CURVE_WITH_KNOTS('',3,(#20087,#20088,#20089,#20090,#20091,
#20092),.UNSPECIFIED.,.F.,.F.,(4,2,4),(0.0638119305867456,0.434740434623819,
0.895232561311264),.UNSPECIFIED.);
#667=B_SPLINE_CURVE_WITH_KNOTS('',3,(#20109,#20110,#20111,#20112,#20113,
#20114,#20115),.UNSPECIFIED.,.F.,.F.,(4,3,4),(0.,0.0653793053833565,0.130355487793492),
 .UNSPECIFIED.);
#668=B_SPLINE_CURVE_WITH_KNOTS('',3,(#20118,#20119,#20120,#20121,#20122,
#20123,#20124,#20125),.UNSPECIFIED.,.F.,.F.,(4,2,2,4),(0.15440517711794,
0.438271814628416,0.790258491635786,1.12994605591364),.UNSPECIFIED.);
#669=B_SPLINE_CURVE_WITH_KNOTS('',3,(#20153,#20154,#20155,#20156,#20157,
#20158),.UNSPECIFIED.,.F.,.F.,(4,2,4),(0.,0.138460176943852,0.254919406858792),
 .UNSPECIFIED.);
#670=B_SPLINE_CURVE_WITH_KNOTS('',3,(#20159,#20160,#20161,#20162,#20163,
#20164),.UNSPECIFIED.,.F.,.F.,(4,2,4),(0.0638119305867455,0.434740434623819,
0.895232561311264),.UNSPECIFIED.);
#671=B_SPLINE_CURVE_WITH_KNOTS('',3,(#20165,#20166,#20167,#20168,#20169,
#20170,#20171,#20172),.UNSPECIFIED.,.F.,.F.,(4,2,2,4),(0.074681186570714,
0.397508022614236,0.744535688298161,1.03619555646797),.UNSPECIFIED.);
#672=B_SPLINE_CURVE_WITH_KNOTS('',3,(#20198,#20199,#20200,#20201,#20202,
#20203,#20204,#20205),.UNSPECIFIED.,.F.,.F.,(4,2,2,4),(0.054434552499654,
0.140376841747107,0.193303927760024,0.233295962211313),.UNSPECIFIED.);
#673=B_SPLINE_CURVE_WITH_KNOTS('',3,(#20206,#20207,#20208,#20209,#20210,
#20211),.UNSPECIFIED.,.F.,.F.,(4,2,4),(0.0638119305867455,0.434740434623819,
0.895232561311264),.UNSPECIFIED.);
#674=B_SPLINE_CURVE_WITH_KNOTS('',3,(#20228,#20229,#20230,#20231,#20232,
#20233,#20234),.UNSPECIFIED.,.F.,.F.,(4,3,4),(0.,0.0653793053832257,0.130355487793195),
 .UNSPECIFIED.);
#675=B_SPLINE_CURVE_WITH_KNOTS('',3,(#20237,#20238,#20239,#20240,#20241,
#20242,#20243,#20244),.UNSPECIFIED.,.F.,.F.,(4,2,2,4),(0.154405177117938,
0.438271814628411,0.790258491635778,1.12994605591362),.UNSPECIFIED.);
#676=B_SPLINE_CURVE_WITH_KNOTS('',3,(#20272,#20273,#20274,#20275,#20276,
#20277),.UNSPECIFIED.,.F.,.F.,(4,2,4),(0.,0.138460176944659,0.254919406872703),
 .UNSPECIFIED.);
#677=B_SPLINE_CURVE_WITH_KNOTS('',3,(#20278,#20279,#20280,#20281,#20282,
#20283),.UNSPECIFIED.,.F.,.F.,(4,2,4),(0.0638119305867456,0.434740434623819,
0.895232561311265),.UNSPECIFIED.);
#678=B_SPLINE_CURVE_WITH_KNOTS('',3,(#20284,#20285,#20286,#20287,#20288,
#20289,#20290,#20291),.UNSPECIFIED.,.F.,.F.,(4,2,2,4),(0.0746811865707118,
0.397508022614199,0.7445356882981,1.05488349691747),.UNSPECIFIED.);
#679=B_SPLINE_CURVE_WITH_KNOTS('',3,(#20317,#20318,#20319,#20320,#20321,
#20322,#20323,#20324),.UNSPECIFIED.,.F.,.F.,(4,2,2,4),(0.0544345524994541,
0.140376841746265,0.193303927760631,0.2332959622117),.UNSPECIFIED.);
#680=B_SPLINE_CURVE_WITH_KNOTS('',3,(#20325,#20326,#20327,#20328,#20329,
#20330),.UNSPECIFIED.,.F.,.F.,(4,2,4),(0.0638119305867456,0.434740434623819,
0.895232561311265),.UNSPECIFIED.);
#681=B_SPLINE_CURVE_WITH_KNOTS('',3,(#20347,#20348,#20349,#20350,#20351,
#20352,#20353),.UNSPECIFIED.,.F.,.F.,(4,3,4),(0.,0.0653793053833301,0.130355487793397),
 .UNSPECIFIED.);
#682=B_SPLINE_CURVE_WITH_KNOTS('',3,(#20356,#20357,#20358,#20359,#20360,
#20361,#20362,#20363),.UNSPECIFIED.,.F.,.F.,(4,2,2,4),(0.0774162478442986,
0.414979417786383,0.760655521250363,1.05194916247819),.UNSPECIFIED.);
#683=B_SPLINE_CURVE_WITH_KNOTS('',3,(#20391,#20392,#20393,#20394,#20395,
#20396),.UNSPECIFIED.,.F.,.F.,(4,2,4),(0.,0.138460176945229,0.254919406868124),
 .UNSPECIFIED.);
#684=B_SPLINE_CURVE_WITH_KNOTS('',3,(#20397,#20398,#20399,#20400,#20401,
#20402),.UNSPECIFIED.,.F.,.F.,(4,2,4),(0.0638119305867456,0.434740434623819,
0.895232561311265),.UNSPECIFIED.);
#685=B_SPLINE_CURVE_WITH_KNOTS('',3,(#20403,#20404,#20405,#20406,#20407,
#20408,#20409,#20410),.UNSPECIFIED.,.F.,.F.,(4,2,2,4),(0.0746811865707123,
0.397508022614217,0.744535688298116,1.03619555646925),.UNSPECIFIED.);
#686=B_SPLINE_CURVE_WITH_KNOTS('',3,(#20436,#20437,#20438,#20439,#20440,
#20441,#20442,#20443),.UNSPECIFIED.,.F.,.F.,(4,2,2,4),(0.0544345524990402,
0.140376841744349,0.193303927756099,0.233295962203159),.UNSPECIFIED.);
#687=B_SPLINE_CURVE_WITH_KNOTS('',3,(#20444,#20445,#20446,#20447,#20448,
#20449),.UNSPECIFIED.,.F.,.F.,(4,2,4),(0.0638119305867457,0.434740434623819,
0.895232561311264),.UNSPECIFIED.);
#688=B_SPLINE_CURVE_WITH_KNOTS('',3,(#20466,#20467,#20468,#20469,#20470,
#20471,#20472),.UNSPECIFIED.,.F.,.F.,(4,3,4),(0.,0.0653793053833115,0.130355487793403),
 .UNSPECIFIED.);
#689=B_SPLINE_CURVE_WITH_KNOTS('',3,(#20475,#20476,#20477,#20478,#20479,
#20480,#20481,#20482),.UNSPECIFIED.,.F.,.F.,(4,2,2,4),(0.154405177117932,
0.438271814628382,0.79025849163572,1.12994605591353),.UNSPECIFIED.);
#690=B_SPLINE_CURVE_WITH_KNOTS('',3,(#20510,#20511,#20512,#20513,#20514,
#20515),.UNSPECIFIED.,.F.,.F.,(4,2,4),(0.,0.138460176945405,0.254919406862959),
 .UNSPECIFIED.);
#691=B_SPLINE_CURVE_WITH_KNOTS('',3,(#20516,#20517,#20518,#20519,#20520,
#20521),.UNSPECIFIED.,.F.,.F.,(4,2,4),(0.0638119305867455,0.434740434623819,
0.895232561311264),.UNSPECIFIED.);
#692=B_SPLINE_CURVE_WITH_KNOTS('',3,(#20522,#20523,#20524,#20525,#20526,
#20527,#20528,#20529),.UNSPECIFIED.,.F.,.F.,(4,2,2,4),(0.0746811865707101,
0.397508022614198,0.744535688298082,1.0361955564677),.UNSPECIFIED.);
#693=B_SPLINE_CURVE_WITH_KNOTS('',3,(#20555,#20556,#20557,#20558,#20559,
#20560,#20561,#20562),.UNSPECIFIED.,.F.,.F.,(4,2,2,4),(0.0544345524991343,
0.140376841744944,0.193303927755901,0.233295962204409),.UNSPECIFIED.);
#694=B_SPLINE_CURVE_WITH_KNOTS('',3,(#20563,#20564,#20565,#20566,#20567,
#20568),.UNSPECIFIED.,.F.,.F.,(4,2,4),(0.0638119305867454,0.434740434623819,
0.895232561311264),.UNSPECIFIED.);
#695=B_SPLINE_CURVE_WITH_KNOTS('',3,(#20585,#20586,#20587,#20588,#20589,
#20590,#20591),.UNSPECIFIED.,.F.,.F.,(4,3,4),(0.,0.065379305383312,0.130355487793393),
 .UNSPECIFIED.);
#696=B_SPLINE_CURVE_WITH_KNOTS('',3,(#20594,#20595,#20596,#20597,#20598,
#20599,#20600,#20601),.UNSPECIFIED.,.F.,.F.,(4,2,2,4),(0.15440517711793,
0.438271814628381,0.790258491635719,1.12994605591353),.UNSPECIFIED.);
#697=B_SPLINE_CURVE_WITH_KNOTS('',3,(#20629,#20630,#20631,#20632,#20633,
#20634),.UNSPECIFIED.,.F.,.F.,(4,2,4),(0.,0.138460176943226,0.254919406847183),
 .UNSPECIFIED.);
#698=B_SPLINE_CURVE_WITH_KNOTS('',3,(#20635,#20636,#20637,#20638,#20639,
#20640),.UNSPECIFIED.,.F.,.F.,(4,2,4),(0.0638119305867456,0.434740434623819,
0.895232561311265),.UNSPECIFIED.);
#699=B_SPLINE_CURVE_WITH_KNOTS('',3,(#20641,#20642,#20643,#20644,#20645,
#20646,#20647,#20648),.UNSPECIFIED.,.F.,.F.,(4,2,2,4),(0.0746811865707119,
0.397508022614209,0.744535688298112,1.03619555646863),.UNSPECIFIED.);
#700=B_SPLINE_CURVE_WITH_KNOTS('',3,(#20674,#20675,#20676,#20677,#20678,
#20679,#20680,#20681),.UNSPECIFIED.,.F.,.F.,(4,2,2,4),(0.0544345524993946,
0.140376841745933,0.193303927757098,0.233295962203211),.UNSPECIFIED.);
#701=B_SPLINE_CURVE_WITH_KNOTS('',3,(#20682,#20683,#20684,#20685,#20686,
#20687),.UNSPECIFIED.,.F.,.F.,(4,2,4),(0.0638119305867456,0.434740434623819,
0.895232561311264),.UNSPECIFIED.);
#702=B_SPLINE_CURVE_WITH_KNOTS('',3,(#20704,#20705,#20706,#20707,#20708,
#20709,#20710),.UNSPECIFIED.,.F.,.F.,(4,3,4),(0.,0.0653793053833217,0.130355487793375),
 .UNSPECIFIED.);
#703=B_SPLINE_CURVE_WITH_KNOTS('',3,(#20713,#20714,#20715,#20716,#20717,
#20718,#20719,#20720),.UNSPECIFIED.,.F.,.F.,(4,2,2,4),(0.154405177117935,
0.4382718146284,0.790258491635752,1.12994605591357),.UNSPECIFIED.);
#704=B_SPLINE_CURVE_WITH_KNOTS('',3,(#20748,#20749,#20750,#20751,#20752,
#20753),.UNSPECIFIED.,.F.,.F.,(4,2,4),(0.,0.138460176944331,0.254919406857816),
 .UNSPECIFIED.);
#705=B_SPLINE_CURVE_WITH_KNOTS('',3,(#20754,#20755,#20756,#20757,#20758,
#20759),.UNSPECIFIED.,.F.,.F.,(4,2,4),(0.0638119305867456,0.434740434623819,
0.895232561311265),.UNSPECIFIED.);
#706=B_SPLINE_CURVE_WITH_KNOTS('',3,(#20760,#20761,#20762,#20763,#20764,
#20765,#20766,#20767),.UNSPECIFIED.,.F.,.F.,(4,2,2,4),(0.0746811865707107,
0.397508022614195,0.744535688298062,1.03619555646822),.UNSPECIFIED.);
#707=B_SPLINE_CURVE_WITH_KNOTS('',3,(#20793,#20794,#20795,#20796,#20797,
#20798,#20799,#20800),.UNSPECIFIED.,.F.,.F.,(4,2,2,4),(0.0544345524991419,
0.140376841744898,0.193303927757274,0.233295962207447),.UNSPECIFIED.);
#708=B_SPLINE_CURVE_WITH_KNOTS('',3,(#20801,#20802,#20803,#20804,#20805,
#20806),.UNSPECIFIED.,.F.,.F.,(4,2,4),(0.0638119305867456,0.434740434623819,
0.895232561311265),.UNSPECIFIED.);
#709=B_SPLINE_CURVE_WITH_KNOTS('',3,(#20823,#20824,#20825,#20826,#20827,
#20828,#20829),.UNSPECIFIED.,.F.,.F.,(4,3,4),(0.,0.065379305383224,0.13035548779319),
 .UNSPECIFIED.);
#710=B_SPLINE_CURVE_WITH_KNOTS('',3,(#20832,#20833,#20834,#20835,#20836,
#20837,#20838,#20839),.UNSPECIFIED.,.F.,.F.,(4,2,2,4),(0.154405177117924,
0.43827181462835,0.79025849163566,1.12994605591344),.UNSPECIFIED.);
#711=B_SPLINE_CURVE_WITH_KNOTS('',3,(#20866,#20867,#20868,#20869,#20870,
#20871),.UNSPECIFIED.,.F.,.F.,(4,2,4),(0.0638119305867455,0.434740434623819,
0.895232561311264),.UNSPECIFIED.);
#712=B_SPLINE_CURVE_WITH_KNOTS('',3,(#20872,#20873,#20874,#20875,#20876,
#20877,#20878,#20879),.UNSPECIFIED.,.F.,.F.,(4,2,2,4),(0.054434552499212,
0.140376841745297,0.193303927759282,0.233295962210278),.UNSPECIFIED.);
#713=B_SPLINE_CURVE_WITH_KNOTS('',3,(#20897,#20898,#20899,#20900,#20901,
#20902),.UNSPECIFIED.,.F.,.F.,(4,2,4),(0.0638119305867455,0.434740434623819,
0.895232561311264),.UNSPECIFIED.);
#714=B_SPLINE_CURVE_WITH_KNOTS('',3,(#20903,#20904,#20905,#20906,#20907,
#20908,#20909),.UNSPECIFIED.,.F.,.F.,(4,3,4),(0.,0.0653793053832804,0.130355487793316),
 .UNSPECIFIED.);
#715=B_SPLINE_CURVE_WITH_KNOTS('',3,(#20935,#20936,#20937,#20938,#20939,
#20940,#20941,#20942),.UNSPECIFIED.,.F.,.F.,(4,2,2,4),(0.0746811865707135,
0.397508022614223,0.744535688298131,1.05488349691753),.UNSPECIFIED.);
#716=B_SPLINE_CURVE_WITH_KNOTS('',3,(#20943,#20944,#20945,#20946,#20947,
#20948),.UNSPECIFIED.,.F.,.F.,(4,2,4),(0.,0.138460176944853,0.254919406867187),
 .UNSPECIFIED.);
#717=B_SPLINE_CURVE_WITH_KNOTS('',3,(#20974,#20975,#20976,#20977,#20978,
#20979),.UNSPECIFIED.,.F.,.F.,(4,2,4),(0.0638119305867456,0.434740434623819,
0.895232561311265),.UNSPECIFIED.);
#718=B_SPLINE_CURVE_WITH_KNOTS('',3,(#20981,#20982,#20983,#20984,#20985,
#20986,#20987,#20988),.UNSPECIFIED.,.F.,.F.,(4,2,2,4),(0.0544345524992891,
0.140376841745541,0.193303927759119,0.23329596220775),.UNSPECIFIED.);
#719=B_SPLINE_CURVE_WITH_KNOTS('',3,(#20989,#20990,#20991,#20992,#20993,
#20994,#20995,#20996),.UNSPECIFIED.,.F.,.F.,(4,2,2,4),(0.0774162478442987,
0.414979417786396,0.760655521250396,1.05194916247824),.UNSPECIFIED.);
#720=B_SPLINE_CURVE_WITH_KNOTS('',3,(#21014,#21015,#21016,#21017,#21018,
#21019),.UNSPECIFIED.,.F.,.F.,(4,2,4),(0.0638119305867456,0.434740434623819,
0.895232561311265),.UNSPECIFIED.);
#721=B_SPLINE_CURVE_WITH_KNOTS('',3,(#21020,#21021,#21022,#21023,#21024,
#21025,#21026),.UNSPECIFIED.,.F.,.F.,(4,3,4),(0.,0.0653793053833094,0.13035548779333),
 .UNSPECIFIED.);
#722=B_SPLINE_CURVE_WITH_KNOTS('',3,(#21051,#21052,#21053,#21054,#21055,
#21056),.UNSPECIFIED.,.F.,.F.,(4,2,4),(0.,0.13846017694525,0.254919406867388),
 .UNSPECIFIED.);
#1206=B_SPLINE_SURFACE_WITH_KNOTS('',3,3,((#18167,#18168,#18169,#18170,
#18171,#18172,#18173,#18174,#18175,#18176,#18177,#18178,#18179,#18180,#18181,
#18182,#18183,#18184,#18185,#18186,#18187,#18188,#18189,#18190,#18191,#18192,
#18193,#18194,#18195),(#18196,#18197,#18198,#18199,#18200,#18201,#18202,
#18203,#18204,#18205,#18206,#18207,#18208,#18209,#18210,#18211,#18212,#18213,
#18214,#18215,#18216,#18217,#18218,#18219,#18220,#18221,#18222,#18223,#18224),
(#18225,#18226,#18227,#18228,#18229,#18230,#18231,#18232,#18233,#18234,
#18235,#18236,#18237,#18238,#18239,#18240,#18241,#18242,#18243,#18244,#18245,
#18246,#18247,#18248,#18249,#18250,#18251,#18252,#18253),(#18254,#18255,
#18256,#18257,#18258,#18259,#18260,#18261,#18262,#18263,#18264,#18265,#18266,
#18267,#18268,#18269,#18270,#18271,#18272,#18273,#18274,#18275,#18276,#18277,
#18278,#18279,#18280,#18281,#18282)),.UNSPECIFIED.,.F.,.T.,.F.,(4,4),(4,
1,2,1,1,1,1,1,1,1,1,1,1,1,1,1,1,1,1,1,1,1,1,1,1,4),(0.,1.),(0.310721506882948,
0.387730825861464,0.464740144839981,0.573091957750491,0.600179910978118,
0.627267864205746,0.654355817433373,0.681443770661001,0.749163653730069,
0.78979558357151,0.843971490026765,0.89814739648202,0.952323302937276,1.00649920939253,
1.06067511584779,1.11485102230304,1.1690269287583,1.22320283521355,1.26383476505499,
1.33155464812406,1.35864260135169,1.38573055457932,1.41281850780694,1.43990646103457,
1.49408236748983,1.54825827394508),.UNSPECIFIED.);
#1207=B_SPLINE_SURFACE_WITH_KNOTS('',3,3,((#18453,#18454,#18455,#18456,
#18457,#18458,#18459,#18460,#18461,#18462,#18463,#18464,#18465,#18466,#18467,
#18468,#18469,#18470,#18471,#18472,#18473,#18474,#18475,#18476,#18477,#18478,
#18479,#18480),(#18481,#18482,#18483,#18484,#18485,#18486,#18487,#18488,
#18489,#18490,#18491,#18492,#18493,#18494,#18495,#18496,#18497,#18498,#18499,
#18500,#18501,#18502,#18503,#18504,#18505,#18506,#18507,#18508),(#18509,
#18510,#18511,#18512,#18513,#18514,#18515,#18516,#18517,#18518,#18519,#18520,
#18521,#18522,#18523,#18524,#18525,#18526,#18527,#18528,#18529,#18530,#18531,
#18532,#18533,#18534,#18535,#18536),(#18537,#18538,#18539,#18540,#18541,
#18542,#18543,#18544,#18545,#18546,#18547,#18548,#18549,#18550,#18551,#18552,
#18553,#18554,#18555,#18556,#18557,#18558,#18559,#18560,#18561,#18562,#18563,
#18564)),.UNSPECIFIED.,.F.,.T.,.F.,(4,4),(4,1,2,1,1,1,1,1,1,1,1,1,1,1,1,
2,2,1,1,1,1,1,4),(0.,1.),(0.930381433825624,1.00739075280414,1.08440007178266,
1.17154004903191,1.21511003765654,1.25868002628116,1.34582000353042,1.38938999215504,
1.43295998077967,1.52009995802892,1.56366994665355,1.58545494096586,1.60723993527817,
1.69437991252743,1.71616490683974,1.78151988977668,1.85897978082803,1.93621438584296,
2.01344899085789,2.03275764211163,2.05206629336536,2.09068359587282,2.16791820088776),
 .UNSPECIFIED.);
#1208=B_SPLINE_SURFACE_WITH_KNOTS('',3,3,((#18674,#18675,#18676,#18677),
(#18678,#18679,#18680,#18681),(#18682,#18683,#18684,#18685),(#18686,#18687,
#18688,#18689),(#18690,#18691,#18692,#18693),(#18694,#18695,#18696,#18697)),
 .UNSPECIFIED.,.F.,.F.,.F.,(4,1,1,4),(4,4),(0.,0.183007073635842,0.366014147271685,
0.854033010300598),(0.0593282328972054,0.895517622296388),.UNSPECIFIED.);
#1209=B_SPLINE_SURFACE_WITH_KNOTS('',3,3,((#18720,#18721,#18722,#18723),
(#18724,#18725,#18726,#18727),(#18728,#18729,#18730,#18731),(#18732,#18733,
#18734,#18735),(#18736,#18737,#18738,#18739),(#18740,#18741,#18742,#18743)),
 .UNSPECIFIED.,.F.,.F.,.F.,(4,1,1,4),(4,4),(0.147257440457363,0.512718537404208,
0.756359268702104,1.),(0.0593287707275125,0.895619345916655),
 .UNSPECIFIED.);
#1210=B_SPLINE_SURFACE_WITH_KNOTS('',3,3,((#18768,#18769,#18770,#18771),
(#18772,#18773,#18774,#18775),(#18776,#18777,#18778,#18779),(#18780,#18781,
#18782,#18783)),.UNSPECIFIED.,.F.,.F.,.F.,(4,4),(4,4),(0.,1.),(0.0638119305867456,
0.897818181014928),.UNSPECIFIED.);
#1211=B_SPLINE_SURFACE_WITH_KNOTS('',3,3,((#18813,#18814,#18815,#18816),
(#18817,#18818,#18819,#18820),(#18821,#18822,#18823,#18824),(#18825,#18826,
#18827,#18828),(#18829,#18830,#18831,#18832),(#18833,#18834,#18835,#18836)),
 .UNSPECIFIED.,.F.,.F.,.F.,(4,1,1,4),(4,4),(0.,0.183007073635851,0.366014147271702,
0.854033010300638),(0.0593282328972055,0.895517622296396),.UNSPECIFIED.);
#1212=B_SPLINE_SURFACE_WITH_KNOTS('',3,3,((#18859,#18860,#18861,#18862),
(#18863,#18864,#18865,#18866),(#18867,#18868,#18869,#18870),(#18871,#18872,
#18873,#18874),(#18875,#18876,#18877,#18878),(#18879,#18880,#18881,#18882)),
 .UNSPECIFIED.,.F.,.F.,.F.,(4,1,1,4),(4,4),(0.147257440457364,0.512718537404208,
0.756359268702104,1.),(0.0593287707275126,0.895619345916652),
 .UNSPECIFIED.);
#1213=B_SPLINE_SURFACE_WITH_KNOTS('',3,3,((#18898,#18899,#18900,#18901),
(#18902,#18903,#18904,#18905),(#18906,#18907,#18908,#18909),(#18910,#18911,
#18912,#18913)),.UNSPECIFIED.,.F.,.F.,.F.,(4,4),(4,4),(0.,1.),(0.0638119305867453,
0.897818181014928),.UNSPECIFIED.);
#1214=B_SPLINE_SURFACE_WITH_KNOTS('',3,3,((#18932,#18933,#18934,#18935),
(#18936,#18937,#18938,#18939),(#18940,#18941,#18942,#18943),(#18944,#18945,
#18946,#18947),(#18948,#18949,#18950,#18951),(#18952,#18953,#18954,#18955)),
 .UNSPECIFIED.,.F.,.F.,.F.,(4,1,1,4),(4,4),(0.,0.183007073635844,0.366014147271687,
0.854033010300603),(0.0593282328972056,0.895517622296375),.UNSPECIFIED.);
#1215=B_SPLINE_SURFACE_WITH_KNOTS('',3,3,((#18978,#18979,#18980,#18981),
(#18982,#18983,#18984,#18985),(#18986,#18987,#18988,#18989),(#18990,#18991,
#18992,#18993),(#18994,#18995,#18996,#18997),(#18998,#18999,#19000,#19001)),
 .UNSPECIFIED.,.F.,.F.,.F.,(4,1,1,4),(4,4),(0.147257440457365,0.634538903053156,
0.817269451526578,1.),(0.0593287707275126,0.895619345916675),
 .UNSPECIFIED.);
#1216=B_SPLINE_SURFACE_WITH_KNOTS('',3,3,((#19017,#19018,#19019,#19020),
(#19021,#19022,#19023,#19024),(#19025,#19026,#19027,#19028),(#19029,#19030,
#19031,#19032)),.UNSPECIFIED.,.F.,.F.,.F.,(4,4),(4,4),(0.,1.),(0.0638119305867456,
0.897818181014929),.UNSPECIFIED.);
#1217=B_SPLINE_SURFACE_WITH_KNOTS('',3,3,((#19051,#19052,#19053,#19054),
(#19055,#19056,#19057,#19058),(#19059,#19060,#19061,#19062),(#19063,#19064,
#19065,#19066),(#19067,#19068,#19069,#19070),(#19071,#19072,#19073,#19074)),
 .UNSPECIFIED.,.F.,.F.,.F.,(4,1,1,4),(4,4),(0.,0.182864493320986,0.365728986641973,
0.853367635497937),(0.0593282328972057,0.895517622296394),.UNSPECIFIED.);
#1218=B_SPLINE_SURFACE_WITH_KNOTS('',3,3,((#19097,#19098,#19099,#19100),
(#19101,#19102,#19103,#19104),(#19105,#19106,#19107,#19108),(#19109,#19110,
#19111,#19112),(#19113,#19114,#19115,#19116),(#19117,#19118,#19119,#19120)),
 .UNSPECIFIED.,.F.,.F.,.F.,(4,1,1,4),(4,4),(0.147257440457363,0.512718537404207,
0.756359268702104,1.),(0.0593287707275127,0.895619345916678),
 .UNSPECIFIED.);
#1219=B_SPLINE_SURFACE_WITH_KNOTS('',3,3,((#19136,#19137,#19138,#19139),
(#19140,#19141,#19142,#19143),(#19144,#19145,#19146,#19147),(#19148,#19149,
#19150,#19151)),.UNSPECIFIED.,.F.,.F.,.F.,(4,4),(4,4),(0.,1.),(0.0638119305867454,
0.897818181014929),.UNSPECIFIED.);
#1220=B_SPLINE_SURFACE_WITH_KNOTS('',3,3,((#19170,#19171,#19172,#19173),
(#19174,#19175,#19176,#19177),(#19178,#19179,#19180,#19181),(#19182,#19183,
#19184,#19185),(#19186,#19187,#19188,#19189),(#19190,#19191,#19192,#19193)),
 .UNSPECIFIED.,.F.,.F.,.F.,(4,1,1,4),(4,4),(0.,0.18300707363585,0.366014147271701,
0.854033010300635),(0.0593282328972055,0.895517622296389),.UNSPECIFIED.);
#1221=B_SPLINE_SURFACE_WITH_KNOTS('',3,3,((#19216,#19217,#19218,#19219),
(#19220,#19221,#19222,#19223),(#19224,#19225,#19226,#19227),(#19228,#19229,
#19230,#19231),(#19232,#19233,#19234,#19235),(#19236,#19237,#19238,#19239)),
 .UNSPECIFIED.,.F.,.F.,.F.,(4,1,1,4),(4,4),(0.146295352012394,0.512168772578511,
0.756084386289255,1.),(0.0593287707275128,0.895619345916675),
 .UNSPECIFIED.);
#1222=B_SPLINE_SURFACE_WITH_KNOTS('',3,3,((#19255,#19256,#19257,#19258),
(#19259,#19260,#19261,#19262),(#19263,#19264,#19265,#19266),(#19267,#19268,
#19269,#19270)),.UNSPECIFIED.,.F.,.F.,.F.,(4,4),(4,4),(0.,1.),(0.0638119305867453,
0.897818181014928),.UNSPECIFIED.);
#1223=B_SPLINE_SURFACE_WITH_KNOTS('',3,3,((#19289,#19290,#19291,#19292),
(#19293,#19294,#19295,#19296),(#19297,#19298,#19299,#19300),(#19301,#19302,
#19303,#19304),(#19305,#19306,#19307,#19308),(#19309,#19310,#19311,#19312)),
 .UNSPECIFIED.,.F.,.F.,.F.,(4,1,1,4),(4,4),(0.,0.183007073635854,0.366014147271708,
0.854033010300653),(0.0593282328972056,0.895517622296374),.UNSPECIFIED.);
#1224=B_SPLINE_SURFACE_WITH_KNOTS('',3,3,((#19335,#19336,#19337,#19338),
(#19339,#19340,#19341,#19342),(#19343,#19344,#19345,#19346),(#19347,#19348,
#19349,#19350),(#19351,#19352,#19353,#19354),(#19355,#19356,#19357,#19358)),
 .UNSPECIFIED.,.F.,.F.,.F.,(4,1,1,4),(4,4),(0.147257440457363,0.512718537404207,
0.756359268702104,1.),(0.0593287707275127,0.895619345916681),
 .UNSPECIFIED.);
#1225=B_SPLINE_SURFACE_WITH_KNOTS('',3,3,((#19374,#19375,#19376,#19377),
(#19378,#19379,#19380,#19381),(#19382,#19383,#19384,#19385),(#19386,#19387,
#19388,#19389)),.UNSPECIFIED.,.F.,.F.,.F.,(4,4),(4,4),(0.,1.),(0.0638119305867453,
0.897818181014928),.UNSPECIFIED.);
#1226=B_SPLINE_SURFACE_WITH_KNOTS('',3,3,((#19408,#19409,#19410,#19411),
(#19412,#19413,#19414,#19415),(#19416,#19417,#19418,#19419),(#19420,#19421,
#19422,#19423),(#19424,#19425,#19426,#19427),(#19428,#19429,#19430,#19431)),
 .UNSPECIFIED.,.F.,.F.,.F.,(4,1,1,4),(4,4),(0.,0.183007073635845,0.36601414727169,
0.854033010300609),(0.0593282328972055,0.895517622296379),.UNSPECIFIED.);
#1227=B_SPLINE_SURFACE_WITH_KNOTS('',3,3,((#19454,#19455,#19456,#19457),
(#19458,#19459,#19460,#19461),(#19462,#19463,#19464,#19465),(#19466,#19467,
#19468,#19469),(#19470,#19471,#19472,#19473),(#19474,#19475,#19476,#19477)),
 .UNSPECIFIED.,.F.,.F.,.F.,(4,1,1,4),(4,4),(0.147257440457364,0.512718537404208,
0.756359268702104,1.),(0.0593287707275128,0.895619345916639),
 .UNSPECIFIED.);
#1228=B_SPLINE_SURFACE_WITH_KNOTS('',3,3,((#19493,#19494,#19495,#19496),
(#19497,#19498,#19499,#19500),(#19501,#19502,#19503,#19504),(#19505,#19506,
#19507,#19508)),.UNSPECIFIED.,.F.,.F.,.F.,(4,4),(4,4),(0.,1.),(0.0638119305867455,
0.897818181014928),.UNSPECIFIED.);
#1229=B_SPLINE_SURFACE_WITH_KNOTS('',3,3,((#19527,#19528,#19529,#19530),
(#19531,#19532,#19533,#19534),(#19535,#19536,#19537,#19538),(#19539,#19540,
#19541,#19542),(#19543,#19544,#19545,#19546),(#19547,#19548,#19549,#19550)),
 .UNSPECIFIED.,.F.,.F.,.F.,(4,1,1,4),(4,4),(0.,0.18300707363585,0.3660141472717,
0.854033010300634),(0.0593282328972057,0.895517622296377),.UNSPECIFIED.);
#1230=B_SPLINE_SURFACE_WITH_KNOTS('',3,3,((#19573,#19574,#19575,#19576),
(#19577,#19578,#19579,#19580),(#19581,#19582,#19583,#19584),(#19585,#19586,
#19587,#19588),(#19589,#19590,#19591,#19592),(#19593,#19594,#19595,#19596)),
 .UNSPECIFIED.,.F.,.F.,.F.,(4,1,1,4),(4,4),(0.147257440457363,0.634538903053156,
0.817269451526578,1.),(0.0593287707275124,0.895619345916661),
 .UNSPECIFIED.);
#1231=B_SPLINE_SURFACE_WITH_KNOTS('',3,3,((#19612,#19613,#19614,#19615),
(#19616,#19617,#19618,#19619),(#19620,#19621,#19622,#19623),(#19624,#19625,
#19626,#19627)),.UNSPECIFIED.,.F.,.F.,.F.,(4,4),(4,4),(0.,1.),(0.0638119305867453,
0.897818181014928),.UNSPECIFIED.);
#1232=B_SPLINE_SURFACE_WITH_KNOTS('',3,3,((#19646,#19647,#19648,#19649),
(#19650,#19651,#19652,#19653),(#19654,#19655,#19656,#19657),(#19658,#19659,
#19660,#19661),(#19662,#19663,#19664,#19665),(#19666,#19667,#19668,#19669)),
 .UNSPECIFIED.,.F.,.F.,.F.,(4,1,1,4),(4,4),(0.,0.182864493320987,0.365728986641974,
0.853367635497938),(0.0593282328972058,0.895517622296391),.UNSPECIFIED.);
#1233=B_SPLINE_SURFACE_WITH_KNOTS('',3,3,((#19692,#19693,#19694,#19695),
(#19696,#19697,#19698,#19699),(#19700,#19701,#19702,#19703),(#19704,#19705,
#19706,#19707),(#19708,#19709,#19710,#19711),(#19712,#19713,#19714,#19715)),
 .UNSPECIFIED.,.F.,.F.,.F.,(4,1,1,4),(4,4),(0.147257440457363,0.634538903053156,
0.817269451526578,1.),(0.059328770727513,0.895619345916667),
 .UNSPECIFIED.);
#1234=B_SPLINE_SURFACE_WITH_KNOTS('',3,3,((#19731,#19732,#19733,#19734),
(#19735,#19736,#19737,#19738),(#19739,#19740,#19741,#19742),(#19743,#19744,
#19745,#19746)),.UNSPECIFIED.,.F.,.F.,.F.,(4,4),(4,4),(0.,1.),(0.0638119305867456,
0.897818181014928),.UNSPECIFIED.);
#1235=B_SPLINE_SURFACE_WITH_KNOTS('',3,3,((#19765,#19766,#19767,#19768),
(#19769,#19770,#19771,#19772),(#19773,#19774,#19775,#19776),(#19777,#19778,
#19779,#19780),(#19781,#19782,#19783,#19784),(#19785,#19786,#19787,#19788)),
 .UNSPECIFIED.,.F.,.F.,.F.,(4,1,1,4),(4,4),(0.,0.183007073635851,0.366014147271702,
0.854033010300638),(0.0593282328972056,0.895517622296395),.UNSPECIFIED.);
#1236=B_SPLINE_SURFACE_WITH_KNOTS('',3,3,((#19816,#19817,#19818,#19819),
(#19820,#19821,#19822,#19823),(#19824,#19825,#19826,#19827),(#19828,#19829,
#19830,#19831),(#19832,#19833,#19834,#19835),(#19836,#19837,#19838,#19839)),
 .UNSPECIFIED.,.F.,.F.,.F.,(4,1,1,4),(4,4),(0.146295352012395,0.512168772578511,
0.756084386289256,1.),(0.0593287707275127,0.895619345916662),
 .UNSPECIFIED.);
#1237=B_SPLINE_SURFACE_WITH_KNOTS('',3,3,((#19855,#19856,#19857,#19858),
(#19859,#19860,#19861,#19862),(#19863,#19864,#19865,#19866),(#19867,#19868,
#19869,#19870)),.UNSPECIFIED.,.F.,.F.,.F.,(4,4),(4,4),(0.,1.),(0.0638119305867453,
0.897818181014928),.UNSPECIFIED.);
#1238=B_SPLINE_SURFACE_WITH_KNOTS('',3,3,((#19889,#19890,#19891,#19892),
(#19893,#19894,#19895,#19896),(#19897,#19898,#19899,#19900),(#19901,#19902,
#19903,#19904),(#19905,#19906,#19907,#19908),(#19909,#19910,#19911,#19912)),
 .UNSPECIFIED.,.F.,.F.,.F.,(4,1,1,4),(4,4),(0.,0.18300707363585,0.3660141472717,
0.854033010300633),(0.0593282328972056,0.895517622296402),.UNSPECIFIED.);
#1239=B_SPLINE_SURFACE_WITH_KNOTS('',3,3,((#19935,#19936,#19937,#19938),
(#19939,#19940,#19941,#19942),(#19943,#19944,#19945,#19946),(#19947,#19948,
#19949,#19950),(#19951,#19952,#19953,#19954),(#19955,#19956,#19957,#19958)),
 .UNSPECIFIED.,.F.,.F.,.F.,(4,1,1,4),(4,4),(0.147257440457363,0.512718537404207,
0.756359268702104,1.),(0.0593287707275125,0.895619345916659),
 .UNSPECIFIED.);
#1240=B_SPLINE_SURFACE_WITH_KNOTS('',3,3,((#19974,#19975,#19976,#19977),
(#19978,#19979,#19980,#19981),(#19982,#19983,#19984,#19985),(#19986,#19987,
#19988,#19989)),.UNSPECIFIED.,.F.,.F.,.F.,(4,4),(4,4),(0.,1.),(0.0638119305867455,
0.897818181014928),.UNSPECIFIED.);
#1241=B_SPLINE_SURFACE_WITH_KNOTS('',3,3,((#20008,#20009,#20010,#20011),
(#20012,#20013,#20014,#20015),(#20016,#20017,#20018,#20019),(#20020,#20021,
#20022,#20023),(#20024,#20025,#20026,#20027),(#20028,#20029,#20030,#20031)),
 .UNSPECIFIED.,.F.,.F.,.F.,(4,1,1,4),(4,4),(0.,0.183007073635855,0.366014147271709,
0.854033010300655),(0.0593282328972057,0.895517622296379),.UNSPECIFIED.);
#1242=B_SPLINE_SURFACE_WITH_KNOTS('',3,3,((#20054,#20055,#20056,#20057),
(#20058,#20059,#20060,#20061),(#20062,#20063,#20064,#20065),(#20066,#20067,
#20068,#20069),(#20070,#20071,#20072,#20073),(#20074,#20075,#20076,#20077)),
 .UNSPECIFIED.,.F.,.F.,.F.,(4,1,1,4),(4,4),(0.147257440457364,0.512718537404208,
0.756359268702104,1.),(0.0593287707275129,0.895619345916649),
 .UNSPECIFIED.);
#1243=B_SPLINE_SURFACE_WITH_KNOTS('',3,3,((#20093,#20094,#20095,#20096),
(#20097,#20098,#20099,#20100),(#20101,#20102,#20103,#20104),(#20105,#20106,
#20107,#20108)),.UNSPECIFIED.,.F.,.F.,.F.,(4,4),(4,4),(0.,1.),(0.0638119305867455,
0.897818181014929),.UNSPECIFIED.);
#1244=B_SPLINE_SURFACE_WITH_KNOTS('',3,3,((#20127,#20128,#20129,#20130),
(#20131,#20132,#20133,#20134),(#20135,#20136,#20137,#20138),(#20139,#20140,
#20141,#20142),(#20143,#20144,#20145,#20146),(#20147,#20148,#20149,#20150)),
 .UNSPECIFIED.,.F.,.F.,.F.,(4,1,1,4),(4,4),(0.,0.183007073635856,0.366014147271713,
0.854033010300663),(0.0593282328972055,0.895517622296378),.UNSPECIFIED.);
#1245=B_SPLINE_SURFACE_WITH_KNOTS('',3,3,((#20173,#20174,#20175,#20176),
(#20177,#20178,#20179,#20180),(#20181,#20182,#20183,#20184),(#20185,#20186,
#20187,#20188),(#20189,#20190,#20191,#20192),(#20193,#20194,#20195,#20196)),
 .UNSPECIFIED.,.F.,.F.,.F.,(4,1,1,4),(4,4),(0.147257440457363,0.512718537404207,
0.756359268702104,1.),(0.0593287707275125,0.895619345916676),
 .UNSPECIFIED.);
#1246=B_SPLINE_SURFACE_WITH_KNOTS('',3,3,((#20212,#20213,#20214,#20215),
(#20216,#20217,#20218,#20219),(#20220,#20221,#20222,#20223),(#20224,#20225,
#20226,#20227)),.UNSPECIFIED.,.F.,.F.,.F.,(4,4),(4,4),(0.,1.),(0.0638119305867453,
0.897818181014928),.UNSPECIFIED.);
#1247=B_SPLINE_SURFACE_WITH_KNOTS('',3,3,((#20246,#20247,#20248,#20249),
(#20250,#20251,#20252,#20253),(#20254,#20255,#20256,#20257),(#20258,#20259,
#20260,#20261),(#20262,#20263,#20264,#20265),(#20266,#20267,#20268,#20269)),
 .UNSPECIFIED.,.F.,.F.,.F.,(4,1,1,4),(4,4),(0.,0.243819324427982,0.487638648855963,
0.853367635497936),(0.0593282328972057,0.895517622296394),.UNSPECIFIED.);
#1248=B_SPLINE_SURFACE_WITH_KNOTS('',3,3,((#20292,#20293,#20294,#20295),
(#20296,#20297,#20298,#20299),(#20300,#20301,#20302,#20303),(#20304,#20305,
#20306,#20307),(#20308,#20309,#20310,#20311),(#20312,#20313,#20314,#20315)),
 .UNSPECIFIED.,.F.,.F.,.F.,(4,1,1,4),(4,4),(0.147257440457363,0.512718537404207,
0.756359268702104,1.),(0.0593287707275129,0.895619345916666),
 .UNSPECIFIED.);
#1249=B_SPLINE_SURFACE_WITH_KNOTS('',3,3,((#20331,#20332,#20333,#20334),
(#20335,#20336,#20337,#20338),(#20339,#20340,#20341,#20342),(#20343,#20344,
#20345,#20346)),.UNSPECIFIED.,.F.,.F.,.F.,(4,4),(4,4),(0.,1.),(0.0638119305867456,
0.897818181014929),.UNSPECIFIED.);
#1250=B_SPLINE_SURFACE_WITH_KNOTS('',3,3,((#20365,#20366,#20367,#20368),
(#20369,#20370,#20371,#20372),(#20373,#20374,#20375,#20376),(#20377,#20378,
#20379,#20380),(#20381,#20382,#20383,#20384),(#20385,#20386,#20387,#20388)),
 .UNSPECIFIED.,.F.,.F.,.F.,(4,1,1,4),(4,4),(0.,0.183007073635844,0.366014147271688,
0.854033010300606),(0.0593282328972055,0.895517622296384),.UNSPECIFIED.);
#1251=B_SPLINE_SURFACE_WITH_KNOTS('',3,3,((#20411,#20412,#20413,#20414),
(#20415,#20416,#20417,#20418),(#20419,#20420,#20421,#20422),(#20423,#20424,
#20425,#20426),(#20427,#20428,#20429,#20430),(#20431,#20432,#20433,#20434)),
 .UNSPECIFIED.,.F.,.F.,.F.,(4,1,1,4),(4,4),(0.146295352012395,0.634126579433884,
0.817063289716942,1.),(0.0593287707275129,0.895619345916667),
 .UNSPECIFIED.);
#1252=B_SPLINE_SURFACE_WITH_KNOTS('',3,3,((#20450,#20451,#20452,#20453),
(#20454,#20455,#20456,#20457),(#20458,#20459,#20460,#20461),(#20462,#20463,
#20464,#20465)),.UNSPECIFIED.,.F.,.F.,.F.,(4,4),(4,4),(0.,1.),(0.0638119305867452,
0.897818181014929),.UNSPECIFIED.);
#1253=B_SPLINE_SURFACE_WITH_KNOTS('',3,3,((#20484,#20485,#20486,#20487),
(#20488,#20489,#20490,#20491),(#20492,#20493,#20494,#20495),(#20496,#20497,
#20498,#20499),(#20500,#20501,#20502,#20503),(#20504,#20505,#20506,#20507)),
 .UNSPECIFIED.,.F.,.F.,.F.,(4,1,1,4),(4,4),(0.,0.183007073635857,0.366014147271714,
0.854033010300667),(0.0593282328972057,0.895517622296367),.UNSPECIFIED.);
#1254=B_SPLINE_SURFACE_WITH_KNOTS('',3,3,((#20530,#20531,#20532,#20533),
(#20534,#20535,#20536,#20537),(#20538,#20539,#20540,#20541),(#20542,#20543,
#20544,#20545),(#20546,#20547,#20548,#20549),(#20550,#20551,#20552,#20553)),
 .UNSPECIFIED.,.F.,.F.,.F.,(4,1,1,4),(4,4),(0.147257440457363,0.512718537404208,
0.756359268702104,1.),(0.0593287707275124,0.89561934591667),
 .UNSPECIFIED.);
#1255=B_SPLINE_SURFACE_WITH_KNOTS('',3,3,((#20569,#20570,#20571,#20572),
(#20573,#20574,#20575,#20576),(#20577,#20578,#20579,#20580),(#20581,#20582,
#20583,#20584)),.UNSPECIFIED.,.F.,.F.,.F.,(4,4),(4,4),(0.,1.),(0.063811930586745,
0.897818181014928),.UNSPECIFIED.);
#1256=B_SPLINE_SURFACE_WITH_KNOTS('',3,3,((#20603,#20604,#20605,#20606),
(#20607,#20608,#20609,#20610),(#20611,#20612,#20613,#20614),(#20615,#20616,
#20617,#20618),(#20619,#20620,#20621,#20622),(#20623,#20624,#20625,#20626)),
 .UNSPECIFIED.,.F.,.F.,.F.,(4,1,1,4),(4,4),(0.,0.18300707363585,0.3660141472717,
0.854033010300632),(0.0593282328972055,0.895517622296395),.UNSPECIFIED.);
#1257=B_SPLINE_SURFACE_WITH_KNOTS('',3,3,((#20649,#20650,#20651,#20652),
(#20653,#20654,#20655,#20656),(#20657,#20658,#20659,#20660),(#20661,#20662,
#20663,#20664),(#20665,#20666,#20667,#20668),(#20669,#20670,#20671,#20672)),
 .UNSPECIFIED.,.F.,.F.,.F.,(4,1,1,4),(4,4),(0.147257440457364,0.634538903053156,
0.817269451526578,1.),(0.0593287707275127,0.895619345916657),
 .UNSPECIFIED.);
#1258=B_SPLINE_SURFACE_WITH_KNOTS('',3,3,((#20688,#20689,#20690,#20691),
(#20692,#20693,#20694,#20695),(#20696,#20697,#20698,#20699),(#20700,#20701,
#20702,#20703)),.UNSPECIFIED.,.F.,.F.,.F.,(4,4),(4,4),(0.,1.),(0.0638119305867455,
0.897818181014928),.UNSPECIFIED.);
#1259=B_SPLINE_SURFACE_WITH_KNOTS('',3,3,((#20722,#20723,#20724,#20725),
(#20726,#20727,#20728,#20729),(#20730,#20731,#20732,#20733),(#20734,#20735,
#20736,#20737),(#20738,#20739,#20740,#20741),(#20742,#20743,#20744,#20745)),
 .UNSPECIFIED.,.F.,.F.,.F.,(4,1,1,4),(4,4),(0.,0.183007073635853,0.366014147271705,
0.854033010300645),(0.0593282328972057,0.895517622296384),.UNSPECIFIED.);
#1260=B_SPLINE_SURFACE_WITH_KNOTS('',3,3,((#20768,#20769,#20770,#20771),
(#20772,#20773,#20774,#20775),(#20776,#20777,#20778,#20779),(#20780,#20781,
#20782,#20783),(#20784,#20785,#20786,#20787),(#20788,#20789,#20790,#20791)),
 .UNSPECIFIED.,.F.,.F.,.F.,(4,1,1,4),(4,4),(0.147257440457364,0.512718537404208,
0.756359268702104,1.),(0.0593287707275128,0.895619345916678),
 .UNSPECIFIED.);
#1261=B_SPLINE_SURFACE_WITH_KNOTS('',3,3,((#20807,#20808,#20809,#20810),
(#20811,#20812,#20813,#20814),(#20815,#20816,#20817,#20818),(#20819,#20820,
#20821,#20822)),.UNSPECIFIED.,.F.,.F.,.F.,(4,4),(4,4),(0.,1.),(0.0638119305867456,
0.897818181014929),.UNSPECIFIED.);
#1262=B_SPLINE_SURFACE_WITH_KNOTS('',3,3,((#20841,#20842,#20843,#20844),
(#20845,#20846,#20847,#20848),(#20849,#20850,#20851,#20852),(#20853,#20854,
#20855,#20856),(#20857,#20858,#20859,#20860),(#20861,#20862,#20863,#20864)),
 .UNSPECIFIED.,.F.,.F.,.F.,(4,1,1,4),(4,4),(0.147257440457363,0.634538903053156,
0.817269451526578,1.),(0.0593287707275126,0.895619345916645),
 .UNSPECIFIED.);
#1263=B_SPLINE_SURFACE_WITH_KNOTS('',3,3,((#20880,#20881,#20882,#20883),
(#20884,#20885,#20886,#20887),(#20888,#20889,#20890,#20891),(#20892,#20893,
#20894,#20895)),.UNSPECIFIED.,.F.,.F.,.F.,(4,4),(4,4),(0.,1.),(0.0638119305867452,
0.897818181014928),.UNSPECIFIED.);
#1264=B_SPLINE_SURFACE_WITH_KNOTS('',3,3,((#20910,#20911,#20912,#20913),
(#20914,#20915,#20916,#20917),(#20918,#20919,#20920,#20921),(#20922,#20923,
#20924,#20925),(#20926,#20927,#20928,#20929),(#20930,#20931,#20932,#20933)),
 .UNSPECIFIED.,.F.,.F.,.F.,(4,1,1,4),(4,4),(0.,0.243819324427982,0.487638648855964,
0.853367635497937),(0.0593282328972056,0.895517622296376),.UNSPECIFIED.);
#1265=B_SPLINE_SURFACE_WITH_KNOTS('',3,3,((#20949,#20950,#20951,#20952),
(#20953,#20954,#20955,#20956),(#20957,#20958,#20959,#20960),(#20961,#20962,
#20963,#20964),(#20965,#20966,#20967,#20968),(#20969,#20970,#20971,#20972)),
 .UNSPECIFIED.,.F.,.F.,.F.,(4,1,1,4),(4,4),(0.146295352012396,0.634126579433884,
0.817063289716942,1.),(0.059328770727513,0.895619345916653),
 .UNSPECIFIED.);
#1266=B_SPLINE_SURFACE_WITH_KNOTS('',3,3,((#20997,#20998,#20999,#21000),
(#21001,#21002,#21003,#21004),(#21005,#21006,#21007,#21008),(#21009,#21010,
#21011,#21012)),.UNSPECIFIED.,.F.,.F.,.F.,(4,4),(4,4),(0.,1.),(0.0638119305867454,
0.897818181014928),.UNSPECIFIED.);
#1267=B_SPLINE_SURFACE_WITH_KNOTS('',3,3,((#21027,#21028,#21029,#21030),
(#21031,#21032,#21033,#21034),(#21035,#21036,#21037,#21038),(#21039,#21040,
#21041,#21042),(#21043,#21044,#21045,#21046),(#21047,#21048,#21049,#21050)),
 .UNSPECIFIED.,.F.,.F.,.F.,(4,1,1,4),(4,4),(0.,0.183007073635845,0.366014147271691,
0.854033010300612),(0.0593282328972056,0.89551762229639),.UNSPECIFIED.);
#1360=FACE_BOUND('',#2665,.T.);
#1361=FACE_BOUND('',#2755,.T.);
#1362=FACE_BOUND('',#2758,.T.);
#1363=FACE_BOUND('',#2759,.T.);
#1364=FACE_BOUND('',#2762,.T.);
#1457=CIRCLE('',#12778,1.35);
#1458=CIRCLE('',#12779,1.43535533905933);
#1459=CIRCLE('',#12780,1.43535533905933);
#1460=CIRCLE('',#12782,1.86384419177103);
#1461=CIRCLE('',#12783,1.86384419177103);
#1462=CIRCLE('',#12784,1.86384419177103);
#1463=CIRCLE('',#12785,1.86384419177103);
#1464=CIRCLE('',#12786,1.86384419177103);
#1465=CIRCLE('',#12787,1.86384419177103);
#1466=CIRCLE('',#12788,1.86384419177103);
#1467=CIRCLE('',#12789,1.86384419177103);
#1468=CIRCLE('',#12790,1.86384419177103);
#1469=CIRCLE('',#12791,1.86384419177103);
#1470=CIRCLE('',#12792,1.86384419177103);
#1471=CIRCLE('',#12793,1.86384419177103);
#1472=CIRCLE('',#12794,1.86384419177103);
#1473=CIRCLE('',#12795,1.86384419177103);
#1474=CIRCLE('',#12796,1.86384419177103);
#1475=CIRCLE('',#12797,1.86384419177103);
#1476=CIRCLE('',#12798,1.86384419177103);
#1477=CIRCLE('',#12799,1.86384419177103);
#1478=CIRCLE('',#12800,1.86384419177103);
#1479=CIRCLE('',#12801,1.86384419177103);
#1480=CIRCLE('',#12803,1.);
#1481=CIRCLE('',#12804,1.);
#1482=CIRCLE('',#12806,1.);
#1483=CIRCLE('',#12807,1.);
#1484=CIRCLE('',#12809,1.);
#1485=CIRCLE('',#12813,0.95);
#1486=CIRCLE('',#12815,1.2613587668218);
#1487=CIRCLE('',#12817,1.2613587668218);
#1488=CIRCLE('',#12819,1.2613587668218);
#1489=CIRCLE('',#12821,1.2613587668218);
#1490=CIRCLE('',#12823,1.2613587668218);
#1491=CIRCLE('',#12825,1.2613587668218);
#1492=CIRCLE('',#12827,1.2613587668218);
#1493=CIRCLE('',#12829,1.2613587668218);
#1494=CIRCLE('',#12831,1.2613587668218);
#1495=CIRCLE('',#12833,1.2613587668218);
#1496=CIRCLE('',#12835,1.2613587668218);
#1497=CIRCLE('',#12837,1.2613587668218);
#1498=CIRCLE('',#12839,1.2613587668218);
#1499=CIRCLE('',#12841,1.2613587668218);
#1500=CIRCLE('',#12843,1.2613587668218);
#1501=CIRCLE('',#12845,1.2613587668218);
#1502=CIRCLE('',#12847,1.2613587668218);
#1503=CIRCLE('',#12849,1.2613587668218);
#1504=CIRCLE('',#12851,1.2613587668218);
#1505=CIRCLE('',#12853,0.7);
#1506=CIRCLE('',#12854,1.2613587668218);
#1507=CIRCLE('',#12857,0.541);
#1508=CIRCLE('',#12859,0.501);
#1509=CIRCLE('',#12861,0.501);
#1510=CIRCLE('',#12863,0.541);
#1948=FACE_OUTER_BOUND('',#2662,.T.);
#1949=FACE_OUTER_BOUND('',#2663,.T.);
#1950=FACE_OUTER_BOUND('',#2664,.T.);
#1951=FACE_OUTER_BOUND('',#2666,.T.);
#1952=FACE_OUTER_BOUND('',#2667,.T.);
#1953=FACE_OUTER_BOUND('',#2668,.T.);
#1954=FACE_OUTER_BOUND('',#2669,.T.);
#1955=FACE_OUTER_BOUND('',#2670,.T.);
#1956=FACE_OUTER_BOUND('',#2671,.T.);
#1957=FACE_OUTER_BOUND('',#2672,.T.);
#1958=FACE_OUTER_BOUND('',#2673,.T.);
#1959=FACE_OUTER_BOUND('',#2674,.T.);
#1960=FACE_OUTER_BOUND('',#2675,.T.);
#1961=FACE_OUTER_BOUND('',#2676,.T.);
#1962=FACE_OUTER_BOUND('',#2677,.T.);
#1963=FACE_OUTER_BOUND('',#2678,.T.);
#1964=FACE_OUTER_BOUND('',#2679,.T.);
#1965=FACE_OUTER_BOUND('',#2680,.T.);
#1966=FACE_OUTER_BOUND('',#2681,.T.);
#1967=FACE_OUTER_BOUND('',#2682,.T.);
#1968=FACE_OUTER_BOUND('',#2683,.T.);
#1969=FACE_OUTER_BOUND('',#2684,.T.);
#1970=FACE_OUTER_BOUND('',#2685,.T.);
#1971=FACE_OUTER_BOUND('',#2686,.T.);
#1972=FACE_OUTER_BOUND('',#2687,.T.);
#1973=FACE_OUTER_BOUND('',#2688,.T.);
#1974=FACE_OUTER_BOUND('',#2689,.T.);
#1975=FACE_OUTER_BOUND('',#2690,.T.);
#1976=FACE_OUTER_BOUND('',#2691,.T.);
#1977=FACE_OUTER_BOUND('',#2692,.T.);
#1978=FACE_OUTER_BOUND('',#2693,.T.);
#1979=FACE_OUTER_BOUND('',#2694,.T.);
#1980=FACE_OUTER_BOUND('',#2695,.T.);
#1981=FACE_OUTER_BOUND('',#2696,.T.);
#1982=FACE_OUTER_BOUND('',#2697,.T.);
#1983=FACE_OUTER_BOUND('',#2698,.T.);
#1984=FACE_OUTER_BOUND('',#2699,.T.);
#1985=FACE_OUTER_BOUND('',#2700,.T.);
#1986=FACE_OUTER_BOUND('',#2701,.T.);
#1987=FACE_OUTER_BOUND('',#2702,.T.);
#1988=FACE_OUTER_BOUND('',#2703,.T.);
#1989=FACE_OUTER_BOUND('',#2704,.T.);
#1990=FACE_OUTER_BOUND('',#2705,.T.);
#1991=FACE_OUTER_BOUND('',#2706,.T.);
#1992=FACE_OUTER_BOUND('',#2707,.T.);
#1993=FACE_OUTER_BOUND('',#2708,.T.);
#1994=FACE_OUTER_BOUND('',#2709,.T.);
#1995=FACE_OUTER_BOUND('',#2710,.T.);
#1996=FACE_OUTER_BOUND('',#2711,.T.);
#1997=FACE_OUTER_BOUND('',#2712,.T.);
#1998=FACE_OUTER_BOUND('',#2713,.T.);
#1999=FACE_OUTER_BOUND('',#2714,.T.);
#2000=FACE_OUTER_BOUND('',#2715,.T.);
#2001=FACE_OUTER_BOUND('',#2716,.T.);
#2002=FACE_OUTER_BOUND('',#2717,.T.);
#2003=FACE_OUTER_BOUND('',#2718,.T.);
#2004=FACE_OUTER_BOUND('',#2719,.T.);
#2005=FACE_OUTER_BOUND('',#2720,.T.);
#2006=FACE_OUTER_BOUND('',#2721,.T.);
#2007=FACE_OUTER_BOUND('',#2722,.T.);
#2008=FACE_OUTER_BOUND('',#2723,.T.);
#2009=FACE_OUTER_BOUND('',#2724,.T.);
#2010=FACE_OUTER_BOUND('',#2725,.T.);
#2011=FACE_OUTER_BOUND('',#2726,.T.);
#2012=FACE_OUTER_BOUND('',#2727,.T.);
#2013=FACE_OUTER_BOUND('',#2728,.T.);
#2014=FACE_OUTER_BOUND('',#2729,.T.);
#2015=FACE_OUTER_BOUND('',#2730,.T.);
#2016=FACE_OUTER_BOUND('',#2731,.T.);
#2017=FACE_OUTER_BOUND('',#2732,.T.);
#2018=FACE_OUTER_BOUND('',#2733,.T.);
#2019=FACE_OUTER_BOUND('',#2734,.T.);
#2020=FACE_OUTER_BOUND('',#2735,.T.);
#2021=FACE_OUTER_BOUND('',#2736,.T.);
#2022=FACE_OUTER_BOUND('',#2737,.T.);
#2023=FACE_OUTER_BOUND('',#2738,.T.);
#2024=FACE_OUTER_BOUND('',#2739,.T.);
#2025=FACE_OUTER_BOUND('',#2740,.T.);
#2026=FACE_OUTER_BOUND('',#2741,.T.);
#2027=FACE_OUTER_BOUND('',#2742,.T.);
#2028=FACE_OUTER_BOUND('',#2743,.T.);
#2029=FACE_OUTER_BOUND('',#2744,.T.);
#2030=FACE_OUTER_BOUND('',#2745,.T.);
#2031=FACE_OUTER_BOUND('',#2746,.T.);
#2032=FACE_OUTER_BOUND('',#2747,.T.);
#2033=FACE_OUTER_BOUND('',#2748,.T.);
#2034=FACE_OUTER_BOUND('',#2749,.T.);
#2035=FACE_OUTER_BOUND('',#2750,.T.);
#2036=FACE_OUTER_BOUND('',#2751,.T.);
#2037=FACE_OUTER_BOUND('',#2752,.T.);
#2038=FACE_OUTER_BOUND('',#2753,.T.);
#2039=FACE_OUTER_BOUND('',#2754,.T.);
#2040=FACE_OUTER_BOUND('',#2756,.T.);
#2041=FACE_OUTER_BOUND('',#2757,.T.);
#2042=FACE_OUTER_BOUND('',#2760,.T.);
#2043=FACE_OUTER_BOUND('',#2761,.T.);
#2662=EDGE_LOOP('',(#8411,#8412,#8413,#8414,#8415));
#2663=EDGE_LOOP('',(#8416,#8417,#8418,#8419,#8420,#8421,#8422,#8423,#8424,
#8425,#8426,#8427,#8428,#8429,#8430,#8431,#8432,#8433,#8434,#8435,#8436,
#8437,#8438,#8439,#8440,#8441,#8442,#8443,#8444,#8445,#8446,#8447,#8448,
#8449,#8450,#8451,#8452,#8453,#8454,#8455,#8456,#8457,#8458,#8459,#8460,
#8461,#8462,#8463,#8464,#8465,#8466,#8467,#8468,#8469,#8470,#8471,#8472,
#8473,#8474,#8475,#8476,#8477,#8478,#8479,#8480,#8481,#8482,#8483,#8484,
#8485,#8486,#8487,#8488,#8489,#8490,#8491,#8492,#8493,#8494,#8495,#8496,
#8497,#8498,#8499,#8500));
#2664=EDGE_LOOP('',(#8501));
#2665=EDGE_LOOP('',(#8502,#8503,#8504,#8505));
#2666=EDGE_LOOP('',(#8506,#8507,#8508,#8509,#8510,#8511,#8512,#8513,#8514));
#2667=EDGE_LOOP('',(#8515,#8516,#8517,#8518,#8519));
#2668=EDGE_LOOP('',(#8520,#8521,#8522,#8523));
#2669=EDGE_LOOP('',(#8524,#8525,#8526,#8527,#8528,#8529));
#2670=EDGE_LOOP('',(#8530,#8531,#8532,#8533,#8534,#8535,#8536,#8537,#8538));
#2671=EDGE_LOOP('',(#8539,#8540,#8541,#8542,#8543,#8544));
#2672=EDGE_LOOP('',(#8545,#8546,#8547,#8548,#8549,#8550,#8551,#8552,#8553,
#8554));
#2673=EDGE_LOOP('',(#8555,#8556,#8557,#8558));
#2674=EDGE_LOOP('',(#8559,#8560,#8561,#8562));
#2675=EDGE_LOOP('',(#8563,#8564,#8565,#8566));
#2676=EDGE_LOOP('',(#8567,#8568,#8569,#8570));
#2677=EDGE_LOOP('',(#8571,#8572,#8573,#8574));
#2678=EDGE_LOOP('',(#8575,#8576,#8577,#8578));
#2679=EDGE_LOOP('',(#8579,#8580,#8581,#8582));
#2680=EDGE_LOOP('',(#8583,#8584,#8585,#8586));
#2681=EDGE_LOOP('',(#8587,#8588,#8589,#8590));
#2682=EDGE_LOOP('',(#8591,#8592,#8593,#8594));
#2683=EDGE_LOOP('',(#8595,#8596,#8597,#8598));
#2684=EDGE_LOOP('',(#8599,#8600,#8601,#8602));
#2685=EDGE_LOOP('',(#8603,#8604,#8605,#8606));
#2686=EDGE_LOOP('',(#8607,#8608,#8609,#8610));
#2687=EDGE_LOOP('',(#8611,#8612,#8613,#8614));
#2688=EDGE_LOOP('',(#8615,#8616,#8617,#8618));
#2689=EDGE_LOOP('',(#8619,#8620,#8621,#8622));
#2690=EDGE_LOOP('',(#8623,#8624,#8625,#8626));
#2691=EDGE_LOOP('',(#8627,#8628,#8629,#8630));
#2692=EDGE_LOOP('',(#8631,#8632,#8633,#8634));
#2693=EDGE_LOOP('',(#8635,#8636,#8637,#8638));
#2694=EDGE_LOOP('',(#8639,#8640,#8641,#8642));
#2695=EDGE_LOOP('',(#8643,#8644,#8645,#8646));
#2696=EDGE_LOOP('',(#8647,#8648,#8649,#8650));
#2697=EDGE_LOOP('',(#8651,#8652,#8653,#8654));
#2698=EDGE_LOOP('',(#8655,#8656,#8657,#8658));
#2699=EDGE_LOOP('',(#8659,#8660,#8661,#8662));
#2700=EDGE_LOOP('',(#8663,#8664,#8665,#8666));
#2701=EDGE_LOOP('',(#8667,#8668,#8669,#8670));
#2702=EDGE_LOOP('',(#8671,#8672,#8673,#8674));
#2703=EDGE_LOOP('',(#8675,#8676,#8677,#8678));
#2704=EDGE_LOOP('',(#8679,#8680,#8681,#8682));
#2705=EDGE_LOOP('',(#8683,#8684,#8685,#8686));
#2706=EDGE_LOOP('',(#8687,#8688,#8689,#8690,#8691));
#2707=EDGE_LOOP('',(#8692,#8693,#8694,#8695));
#2708=EDGE_LOOP('',(#8696,#8697,#8698,#8699));
#2709=EDGE_LOOP('',(#8700,#8701,#8702,#8703));
#2710=EDGE_LOOP('',(#8704,#8705,#8706,#8707,#8708));
#2711=EDGE_LOOP('',(#8709,#8710,#8711,#8712));
#2712=EDGE_LOOP('',(#8713,#8714,#8715,#8716));
#2713=EDGE_LOOP('',(#8717,#8718,#8719,#8720));
#2714=EDGE_LOOP('',(#8721,#8722,#8723,#8724));
#2715=EDGE_LOOP('',(#8725,#8726,#8727,#8728));
#2716=EDGE_LOOP('',(#8729,#8730,#8731,#8732));
#2717=EDGE_LOOP('',(#8733,#8734,#8735,#8736));
#2718=EDGE_LOOP('',(#8737,#8738,#8739,#8740));
#2719=EDGE_LOOP('',(#8741,#8742,#8743,#8744));
#2720=EDGE_LOOP('',(#8745,#8746,#8747,#8748));
#2721=EDGE_LOOP('',(#8749,#8750,#8751,#8752));
#2722=EDGE_LOOP('',(#8753,#8754,#8755,#8756));
#2723=EDGE_LOOP('',(#8757,#8758,#8759,#8760));
#2724=EDGE_LOOP('',(#8761,#8762,#8763,#8764));
#2725=EDGE_LOOP('',(#8765,#8766,#8767,#8768));
#2726=EDGE_LOOP('',(#8769,#8770,#8771,#8772));
#2727=EDGE_LOOP('',(#8773,#8774,#8775,#8776));
#2728=EDGE_LOOP('',(#8777,#8778,#8779,#8780));
#2729=EDGE_LOOP('',(#8781,#8782,#8783,#8784));
#2730=EDGE_LOOP('',(#8785,#8786,#8787,#8788));
#2731=EDGE_LOOP('',(#8789,#8790,#8791,#8792));
#2732=EDGE_LOOP('',(#8793,#8794,#8795,#8796));
#2733=EDGE_LOOP('',(#8797,#8798,#8799,#8800));
#2734=EDGE_LOOP('',(#8801,#8802,#8803,#8804));
#2735=EDGE_LOOP('',(#8805,#8806,#8807,#8808));
#2736=EDGE_LOOP('',(#8809,#8810,#8811,#8812));
#2737=EDGE_LOOP('',(#8813,#8814,#8815,#8816));
#2738=EDGE_LOOP('',(#8817,#8818,#8819,#8820));
#2739=EDGE_LOOP('',(#8821,#8822,#8823,#8824));
#2740=EDGE_LOOP('',(#8825,#8826,#8827,#8828));
#2741=EDGE_LOOP('',(#8829,#8830,#8831,#8832));
#2742=EDGE_LOOP('',(#8833,#8834,#8835,#8836));
#2743=EDGE_LOOP('',(#8837,#8838,#8839,#8840));
#2744=EDGE_LOOP('',(#8841,#8842,#8843,#8844));
#2745=EDGE_LOOP('',(#8845,#8846,#8847,#8848));
#2746=EDGE_LOOP('',(#8849,#8850,#8851,#8852));
#2747=EDGE_LOOP('',(#8853,#8854,#8855,#8856));
#2748=EDGE_LOOP('',(#8857,#8858,#8859,#8860));
#2749=EDGE_LOOP('',(#8861,#8862,#8863,#8864));
#2750=EDGE_LOOP('',(#8865,#8866,#8867,#8868));
#2751=EDGE_LOOP('',(#8869,#8870,#8871,#8872));
#2752=EDGE_LOOP('',(#8873,#8874,#8875,#8876,#8877,#8878,#8879,#8880,#8881,
#8882,#8883,#8884,#8885,#8886,#8887,#8888,#8889,#8890,#8891,#8892,#8893,
#8894,#8895,#8896,#8897,#8898,#8899,#8900,#8901,#8902,#8903,#8904,#8905,
#8906,#8907,#8908,#8909,#8910,#8911,#8912,#8913,#8914,#8915,#8916,#8917,
#8918,#8919,#8920,#8921,#8922,#8923,#8924,#8925,#8926,#8927,#8928,#8929,
#8930,#8931,#8932,#8933,#8934,#8935,#8936,#8937,#8938,#8939,#8940,#8941,
#8942,#8943,#8944,#8945,#8946,#8947,#8948,#8949,#8950,#8951,#8952,#8953,
#8954,#8955,#8956));
#2753=EDGE_LOOP('',(#8957,#8958,#8959,#8960));
#2754=EDGE_LOOP('',(#8961));
#2755=EDGE_LOOP('',(#8962));
#2756=EDGE_LOOP('',(#8963,#8964,#8965,#8966));
#2757=EDGE_LOOP('',(#8967,#8968,#8969,#8970));
#2758=EDGE_LOOP('',(#8971,#8972));
#2759=EDGE_LOOP('',(#8973,#8974));
#2760=EDGE_LOOP('',(#8975,#8976,#8977,#8978));
#2761=EDGE_LOOP('',(#8979));
#2762=EDGE_LOOP('',(#8980));
#3505=LINE('',#17558,#4210);
#3506=LINE('',#17564,#4211);
#3507=LINE('',#18415,#4212);
#3508=LINE('',#18669,#4213);
#3509=LINE('',#18673,#4214);
#3510=LINE('',#21060,#4215);
#3511=LINE('',#21068,#4216);
#3512=LINE('',#21072,#4217);
#3513=LINE('',#21076,#4218);
#4210=VECTOR('',#14185,1.39267766952966);
#4211=VECTOR('',#14192,1.63192209588552);
#4212=VECTOR('',#14251,0.205);
#4213=VECTOR('',#14254,0.205);
#4214=VECTOR('',#14259,0.975);
#4215=VECTOR('',#14340,0.980679383410898);
#4216=VECTOR('',#14351,0.521);
#4217=VECTOR('',#14356,0.501);
#4218=VECTOR('',#14361,0.521);
#4890=VERTEX_POINT('',#17555);
#4891=VERTEX_POINT('',#17557);
#4892=VERTEX_POINT('',#17559);
#4893=VERTEX_POINT('',#17563);
#4894=VERTEX_POINT('',#17565);
#4895=VERTEX_POINT('',#17574);
#4896=VERTEX_POINT('',#17582);
#4897=VERTEX_POINT('',#17589);
#4898=VERTEX_POINT('',#17591);
#4899=VERTEX_POINT('',#17600);
#4900=VERTEX_POINT('',#17608);
#4901=VERTEX_POINT('',#17615);
#4902=VERTEX_POINT('',#17617);
#4903=VERTEX_POINT('',#17626);
#4904=VERTEX_POINT('',#17634);
#4905=VERTEX_POINT('',#17641);
#4906=VERTEX_POINT('',#17643);
#4907=VERTEX_POINT('',#17652);
#4908=VERTEX_POINT('',#17660);
#4909=VERTEX_POINT('',#17667);
#4910=VERTEX_POINT('',#17669);
#4911=VERTEX_POINT('',#17678);
#4912=VERTEX_POINT('',#17686);
#4913=VERTEX_POINT('',#17693);
#4914=VERTEX_POINT('',#17695);
#4915=VERTEX_POINT('',#17704);
#4916=VERTEX_POINT('',#17712);
#4917=VERTEX_POINT('',#17719);
#4918=VERTEX_POINT('',#17721);
#4919=VERTEX_POINT('',#17730);
#4920=VERTEX_POINT('',#17738);
#4921=VERTEX_POINT('',#17745);
#4922=VERTEX_POINT('',#17747);
#4923=VERTEX_POINT('',#17756);
#4924=VERTEX_POINT('',#17764);
#4925=VERTEX_POINT('',#17771);
#4926=VERTEX_POINT('',#17773);
#4927=VERTEX_POINT('',#17782);
#4928=VERTEX_POINT('',#17790);
#4929=VERTEX_POINT('',#17797);
#4930=VERTEX_POINT('',#17799);
#4931=VERTEX_POINT('',#17808);
#4932=VERTEX_POINT('',#17816);
#4933=VERTEX_POINT('',#17823);
#4934=VERTEX_POINT('',#17825);
#4935=VERTEX_POINT('',#17834);
#4936=VERTEX_POINT('',#17842);
#4937=VERTEX_POINT('',#17849);
#4938=VERTEX_POINT('',#17851);
#4939=VERTEX_POINT('',#17860);
#4940=VERTEX_POINT('',#17868);
#4941=VERTEX_POINT('',#17875);
#4942=VERTEX_POINT('',#17877);
#4943=VERTEX_POINT('',#17886);
#4944=VERTEX_POINT('',#17894);
#4945=VERTEX_POINT('',#17901);
#4946=VERTEX_POINT('',#17903);
#4947=VERTEX_POINT('',#17912);
#4948=VERTEX_POINT('',#17920);
#4949=VERTEX_POINT('',#17927);
#4950=VERTEX_POINT('',#17929);
#4951=VERTEX_POINT('',#17938);
#4952=VERTEX_POINT('',#17946);
#4953=VERTEX_POINT('',#17953);
#4954=VERTEX_POINT('',#17955);
#4955=VERTEX_POINT('',#17964);
#4956=VERTEX_POINT('',#17972);
#4957=VERTEX_POINT('',#17979);
#4958=VERTEX_POINT('',#17981);
#4959=VERTEX_POINT('',#17990);
#4960=VERTEX_POINT('',#17998);
#4961=VERTEX_POINT('',#18005);
#4962=VERTEX_POINT('',#18007);
#4963=VERTEX_POINT('',#18016);
#4964=VERTEX_POINT('',#18024);
#4965=VERTEX_POINT('',#18031);
#4966=VERTEX_POINT('',#18033);
#4967=VERTEX_POINT('',#18042);
#4968=VERTEX_POINT('',#18050);
#4969=VERTEX_POINT('',#18057);
#4970=VERTEX_POINT('',#18059);
#4971=VERTEX_POINT('',#18068);
#4972=VERTEX_POINT('',#18076);
#4973=VERTEX_POINT('',#18083);
#4974=VERTEX_POINT('',#18090);
#4975=VERTEX_POINT('',#18091);
#4976=VERTEX_POINT('',#18093);
#4977=VERTEX_POINT('',#18131);
#4978=VERTEX_POINT('',#18283);
#4979=VERTEX_POINT('',#18298);
#4980=VERTEX_POINT('',#18311);
#4981=VERTEX_POINT('',#18316);
#4982=VERTEX_POINT('',#18350);
#4983=VERTEX_POINT('',#18380);
#4984=VERTEX_POINT('',#18382);
#4985=VERTEX_POINT('',#18397);
#4986=VERTEX_POINT('',#18414);
#4987=VERTEX_POINT('',#18416);
#4988=VERTEX_POINT('',#18565);
#4989=VERTEX_POINT('',#18578);
#4990=VERTEX_POINT('',#18583);
#4991=VERTEX_POINT('',#18631);
#4992=VERTEX_POINT('',#18632);
#4993=VERTEX_POINT('',#18671);
#4994=VERTEX_POINT('',#18698);
#4995=VERTEX_POINT('',#18699);
#4996=VERTEX_POINT('',#18744);
#4997=VERTEX_POINT('',#18745);
#4998=VERTEX_POINT('',#18792);
#4999=VERTEX_POINT('',#18803);
#5000=VERTEX_POINT('',#18837);
#5001=VERTEX_POINT('',#18838);
#5002=VERTEX_POINT('',#18883);
#5003=VERTEX_POINT('',#18922);
#5004=VERTEX_POINT('',#18956);
#5005=VERTEX_POINT('',#18957);
#5006=VERTEX_POINT('',#19002);
#5007=VERTEX_POINT('',#19041);
#5008=VERTEX_POINT('',#19075);
#5009=VERTEX_POINT('',#19076);
#5010=VERTEX_POINT('',#19121);
#5011=VERTEX_POINT('',#19160);
#5012=VERTEX_POINT('',#19194);
#5013=VERTEX_POINT('',#19195);
#5014=VERTEX_POINT('',#19240);
#5015=VERTEX_POINT('',#19279);
#5016=VERTEX_POINT('',#19313);
#5017=VERTEX_POINT('',#19314);
#5018=VERTEX_POINT('',#19359);
#5019=VERTEX_POINT('',#19398);
#5020=VERTEX_POINT('',#19432);
#5021=VERTEX_POINT('',#19433);
#5022=VERTEX_POINT('',#19478);
#5023=VERTEX_POINT('',#19517);
#5024=VERTEX_POINT('',#19551);
#5025=VERTEX_POINT('',#19552);
#5026=VERTEX_POINT('',#19597);
#5027=VERTEX_POINT('',#19636);
#5028=VERTEX_POINT('',#19670);
#5029=VERTEX_POINT('',#19671);
#5030=VERTEX_POINT('',#19716);
#5031=VERTEX_POINT('',#19755);
#5032=VERTEX_POINT('',#19789);
#5033=VERTEX_POINT('',#19790);
#5034=VERTEX_POINT('',#19803);
#5035=VERTEX_POINT('',#19840);
#5036=VERTEX_POINT('',#19879);
#5037=VERTEX_POINT('',#19913);
#5038=VERTEX_POINT('',#19914);
#5039=VERTEX_POINT('',#19959);
#5040=VERTEX_POINT('',#19998);
#5041=VERTEX_POINT('',#20032);
#5042=VERTEX_POINT('',#20033);
#5043=VERTEX_POINT('',#20078);
#5044=VERTEX_POINT('',#20117);
#5045=VERTEX_POINT('',#20151);
#5046=VERTEX_POINT('',#20152);
#5047=VERTEX_POINT('',#20197);
#5048=VERTEX_POINT('',#20236);
#5049=VERTEX_POINT('',#20270);
#5050=VERTEX_POINT('',#20271);
#5051=VERTEX_POINT('',#20316);
#5052=VERTEX_POINT('',#20355);
#5053=VERTEX_POINT('',#20389);
#5054=VERTEX_POINT('',#20390);
#5055=VERTEX_POINT('',#20435);
#5056=VERTEX_POINT('',#20474);
#5057=VERTEX_POINT('',#20508);
#5058=VERTEX_POINT('',#20509);
#5059=VERTEX_POINT('',#20554);
#5060=VERTEX_POINT('',#20593);
#5061=VERTEX_POINT('',#20627);
#5062=VERTEX_POINT('',#20628);
#5063=VERTEX_POINT('',#20673);
#5064=VERTEX_POINT('',#20712);
#5065=VERTEX_POINT('',#20746);
#5066=VERTEX_POINT('',#20747);
#5067=VERTEX_POINT('',#20792);
#5068=VERTEX_POINT('',#20831);
#5069=VERTEX_POINT('',#20865);
#5070=VERTEX_POINT('',#20896);
#5071=VERTEX_POINT('',#20934);
#5072=VERTEX_POINT('',#20973);
#5073=VERTEX_POINT('',#20980);
#5074=VERTEX_POINT('',#21013);
#5075=VERTEX_POINT('',#21058);
#5076=VERTEX_POINT('',#21064);
#5077=VERTEX_POINT('',#21067);
#5078=VERTEX_POINT('',#21071);
#5079=VERTEX_POINT('',#21075);
#6217=EDGE_CURVE('',#4890,#4890,#1457,.T.);
#6218=EDGE_CURVE('',#4890,#4891,#3505,.T.);
#6219=EDGE_CURVE('',#4891,#4892,#1458,.T.);
#6220=EDGE_CURVE('',#4892,#4891,#1459,.T.);
#6221=EDGE_CURVE('',#4892,#4893,#3506,.T.);
#6222=EDGE_CURVE('',#4893,#4894,#501,.T.);
#6223=EDGE_CURVE('',#4894,#4895,#502,.T.);
#6224=EDGE_CURVE('',#4895,#4896,#503,.T.);
#6225=EDGE_CURVE('',#4896,#4897,#1460,.T.);
#6226=EDGE_CURVE('',#4897,#4898,#504,.T.);
#6227=EDGE_CURVE('',#4898,#4899,#505,.T.);
#6228=EDGE_CURVE('',#4899,#4900,#506,.T.);
#6229=EDGE_CURVE('',#4900,#4901,#1461,.T.);
#6230=EDGE_CURVE('',#4901,#4902,#507,.T.);
#6231=EDGE_CURVE('',#4902,#4903,#508,.T.);
#6232=EDGE_CURVE('',#4903,#4904,#509,.T.);
#6233=EDGE_CURVE('',#4904,#4905,#1462,.T.);
#6234=EDGE_CURVE('',#4905,#4906,#510,.T.);
#6235=EDGE_CURVE('',#4906,#4907,#511,.T.);
#6236=EDGE_CURVE('',#4907,#4908,#512,.T.);
#6237=EDGE_CURVE('',#4908,#4909,#1463,.T.);
#6238=EDGE_CURVE('',#4909,#4910,#513,.T.);
#6239=EDGE_CURVE('',#4910,#4911,#514,.T.);
#6240=EDGE_CURVE('',#4911,#4912,#515,.T.);
#6241=EDGE_CURVE('',#4912,#4913,#1464,.T.);
#6242=EDGE_CURVE('',#4913,#4914,#516,.T.);
#6243=EDGE_CURVE('',#4914,#4915,#517,.T.);
#6244=EDGE_CURVE('',#4915,#4916,#518,.T.);
#6245=EDGE_CURVE('',#4916,#4917,#1465,.T.);
#6246=EDGE_CURVE('',#4917,#4918,#519,.T.);
#6247=EDGE_CURVE('',#4918,#4919,#520,.T.);
#6248=EDGE_CURVE('',#4919,#4920,#521,.T.);
#6249=EDGE_CURVE('',#4920,#4921,#1466,.T.);
#6250=EDGE_CURVE('',#4921,#4922,#522,.T.);
#6251=EDGE_CURVE('',#4922,#4923,#523,.T.);
#6252=EDGE_CURVE('',#4923,#4924,#524,.T.);
#6253=EDGE_CURVE('',#4924,#4925,#1467,.T.);
#6254=EDGE_CURVE('',#4925,#4926,#525,.T.);
#6255=EDGE_CURVE('',#4926,#4927,#526,.T.);
#6256=EDGE_CURVE('',#4927,#4928,#527,.T.);
#6257=EDGE_CURVE('',#4928,#4929,#1468,.T.);
#6258=EDGE_CURVE('',#4929,#4930,#528,.T.);
#6259=EDGE_CURVE('',#4930,#4931,#529,.T.);
#6260=EDGE_CURVE('',#4931,#4932,#530,.T.);
#6261=EDGE_CURVE('',#4932,#4933,#1469,.T.);
#6262=EDGE_CURVE('',#4933,#4934,#531,.T.);
#6263=EDGE_CURVE('',#4934,#4935,#532,.T.);
#6264=EDGE_CURVE('',#4935,#4936,#533,.T.);
#6265=EDGE_CURVE('',#4936,#4937,#1470,.T.);
#6266=EDGE_CURVE('',#4937,#4938,#534,.T.);
#6267=EDGE_CURVE('',#4938,#4939,#535,.T.);
#6268=EDGE_CURVE('',#4939,#4940,#536,.T.);
#6269=EDGE_CURVE('',#4940,#4941,#1471,.T.);
#6270=EDGE_CURVE('',#4941,#4942,#537,.T.);
#6271=EDGE_CURVE('',#4942,#4943,#538,.T.);
#6272=EDGE_CURVE('',#4943,#4944,#539,.T.);
#6273=EDGE_CURVE('',#4944,#4945,#1472,.T.);
#6274=EDGE_CURVE('',#4945,#4946,#540,.T.);
#6275=EDGE_CURVE('',#4946,#4947,#541,.T.);
#6276=EDGE_CURVE('',#4947,#4948,#542,.T.);
#6277=EDGE_CURVE('',#4948,#4949,#1473,.T.);
#6278=EDGE_CURVE('',#4949,#4950,#543,.T.);
#6279=EDGE_CURVE('',#4950,#4951,#544,.T.);
#6280=EDGE_CURVE('',#4951,#4952,#545,.T.);
#6281=EDGE_CURVE('',#4952,#4953,#1474,.T.);
#6282=EDGE_CURVE('',#4953,#4954,#546,.T.);
#6283=EDGE_CURVE('',#4954,#4955,#547,.T.);
#6284=EDGE_CURVE('',#4955,#4956,#548,.T.);
#6285=EDGE_CURVE('',#4956,#4957,#1475,.T.);
#6286=EDGE_CURVE('',#4957,#4958,#549,.T.);
#6287=EDGE_CURVE('',#4958,#4959,#550,.T.);
#6288=EDGE_CURVE('',#4959,#4960,#551,.T.);
#6289=EDGE_CURVE('',#4960,#4961,#1476,.T.);
#6290=EDGE_CURVE('',#4961,#4962,#552,.T.);
#6291=EDGE_CURVE('',#4962,#4963,#553,.T.);
#6292=EDGE_CURVE('',#4963,#4964,#554,.T.);
#6293=EDGE_CURVE('',#4964,#4965,#1477,.T.);
#6294=EDGE_CURVE('',#4965,#4966,#555,.T.);
#6295=EDGE_CURVE('',#4966,#4967,#556,.T.);
#6296=EDGE_CURVE('',#4967,#4968,#557,.T.);
#6297=EDGE_CURVE('',#4968,#4969,#1478,.T.);
#6298=EDGE_CURVE('',#4969,#4970,#558,.T.);
#6299=EDGE_CURVE('',#4970,#4971,#559,.T.);
#6300=EDGE_CURVE('',#4971,#4972,#560,.T.);
#6301=EDGE_CURVE('',#4972,#4973,#1479,.T.);
#6302=EDGE_CURVE('',#4973,#4893,#561,.T.);
#6303=EDGE_CURVE('',#4974,#4975,#1480,.T.);
#6304=EDGE_CURVE('',#4974,#4976,#562,.T.);
#6305=EDGE_CURVE('',#4977,#4976,#1481,.T.);
#6306=EDGE_CURVE('',#4977,#4975,#563,.T.);
#6307=EDGE_CURVE('',#4977,#4978,#564,.T.);
#6308=EDGE_CURVE('',#4978,#4979,#565,.T.);
#6309=EDGE_CURVE('',#4979,#4980,#566,.T.);
#6310=EDGE_CURVE('',#4980,#4981,#567,.T.);
#6311=EDGE_CURVE('',#4981,#4980,#568,.T.);
#6312=EDGE_CURVE('',#4979,#4982,#569,.T.);
#6313=EDGE_CURVE('',#4982,#4975,#570,.T.);
#6314=EDGE_CURVE('',#4983,#4982,#1482,.T.);
#6315=EDGE_CURVE('',#4984,#4983,#1483,.T.);
#6316=EDGE_CURVE('',#4974,#4984,#571,.T.);
#6317=EDGE_CURVE('',#4985,#4976,#572,.T.);
#6318=EDGE_CURVE('',#4978,#4985,#1484,.T.);
#6319=EDGE_CURVE('',#4981,#4986,#3507,.T.);
#6320=EDGE_CURVE('',#4987,#4986,#573,.T.);
#6321=EDGE_CURVE('',#4986,#4987,#574,.T.);
#6322=EDGE_CURVE('',#4984,#4988,#575,.T.);
#6323=EDGE_CURVE('',#4988,#4989,#576,.T.);
#6324=EDGE_CURVE('',#4989,#4990,#577,.T.);
#6325=EDGE_CURVE('',#4990,#4989,#578,.T.);
#6326=EDGE_CURVE('',#4988,#4985,#579,.T.);
#6327=EDGE_CURVE('',#4991,#4992,#580,.T.);
#6328=EDGE_CURVE('',#4992,#4991,#581,.T.);
#6329=EDGE_CURVE('',#4992,#4990,#3508,.T.);
#6330=EDGE_CURVE('',#4993,#4993,#1485,.T.);
#6331=EDGE_CURVE('',#4993,#4983,#3509,.T.);
#6332=EDGE_CURVE('',#4994,#4995,#582,.T.);
#6333=EDGE_CURVE('',#4994,#4926,#583,.T.);
#6334=EDGE_CURVE('',#4995,#4925,#584,.T.);
#6335=EDGE_CURVE('',#4996,#4997,#585,.T.);
#6336=EDGE_CURVE('',#4928,#4996,#586,.T.);
#6337=EDGE_CURVE('',#4997,#4927,#587,.T.);
#6338=EDGE_CURVE('',#4997,#4994,#588,.T.);
#6339=EDGE_CURVE('',#4996,#4998,#1486,.T.);
#6340=EDGE_CURVE('',#4998,#4929,#589,.T.);
#6341=EDGE_CURVE('',#4924,#4999,#590,.T.);
#6342=EDGE_CURVE('',#4999,#4995,#1487,.T.);
#6343=EDGE_CURVE('',#5000,#5001,#591,.T.);
#6344=EDGE_CURVE('',#5000,#4922,#592,.T.);
#6345=EDGE_CURVE('',#5001,#4921,#593,.T.);
#6346=EDGE_CURVE('',#4999,#5002,#594,.T.);
#6347=EDGE_CURVE('',#5002,#4923,#595,.T.);
#6348=EDGE_CURVE('',#5002,#5000,#596,.T.);
#6349=EDGE_CURVE('',#4920,#5003,#597,.T.);
#6350=EDGE_CURVE('',#5003,#5001,#1488,.T.);
#6351=EDGE_CURVE('',#5004,#5005,#598,.T.);
#6352=EDGE_CURVE('',#5004,#4918,#599,.T.);
#6353=EDGE_CURVE('',#5005,#4917,#600,.T.);
#6354=EDGE_CURVE('',#5003,#5006,#601,.T.);
#6355=EDGE_CURVE('',#5006,#4919,#602,.T.);
#6356=EDGE_CURVE('',#5006,#5004,#603,.T.);
#6357=EDGE_CURVE('',#4916,#5007,#604,.T.);
#6358=EDGE_CURVE('',#5007,#5005,#1489,.T.);
#6359=EDGE_CURVE('',#5008,#5009,#605,.T.);
#6360=EDGE_CURVE('',#5008,#4914,#606,.T.);
#6361=EDGE_CURVE('',#5009,#4913,#607,.T.);
#6362=EDGE_CURVE('',#5007,#5010,#608,.T.);
#6363=EDGE_CURVE('',#5010,#4915,#609,.T.);
#6364=EDGE_CURVE('',#5010,#5008,#610,.T.);
#6365=EDGE_CURVE('',#4912,#5011,#611,.T.);
#6366=EDGE_CURVE('',#5011,#5009,#1490,.T.);
#6367=EDGE_CURVE('',#5012,#5013,#612,.T.);
#6368=EDGE_CURVE('',#5012,#4910,#613,.T.);
#6369=EDGE_CURVE('',#5013,#4909,#614,.T.);
#6370=EDGE_CURVE('',#5011,#5014,#615,.T.);
#6371=EDGE_CURVE('',#5014,#4911,#616,.T.);
#6372=EDGE_CURVE('',#5014,#5012,#617,.T.);
#6373=EDGE_CURVE('',#4908,#5015,#618,.T.);
#6374=EDGE_CURVE('',#5015,#5013,#1491,.T.);
#6375=EDGE_CURVE('',#5016,#5017,#619,.T.);
#6376=EDGE_CURVE('',#5016,#4906,#620,.T.);
#6377=EDGE_CURVE('',#5017,#4905,#621,.T.);
#6378=EDGE_CURVE('',#5015,#5018,#622,.T.);
#6379=EDGE_CURVE('',#5018,#4907,#623,.T.);
#6380=EDGE_CURVE('',#5018,#5016,#624,.T.);
#6381=EDGE_CURVE('',#4904,#5019,#625,.T.);
#6382=EDGE_CURVE('',#5019,#5017,#1492,.T.);
#6383=EDGE_CURVE('',#5020,#5021,#626,.T.);
#6384=EDGE_CURVE('',#5020,#4902,#627,.T.);
#6385=EDGE_CURVE('',#5021,#4901,#628,.T.);
#6386=EDGE_CURVE('',#5019,#5022,#629,.T.);
#6387=EDGE_CURVE('',#5022,#4903,#630,.T.);
#6388=EDGE_CURVE('',#5022,#5020,#631,.T.);
#6389=EDGE_CURVE('',#4900,#5023,#632,.T.);
#6390=EDGE_CURVE('',#5023,#5021,#1493,.T.);
#6391=EDGE_CURVE('',#5024,#5025,#633,.T.);
#6392=EDGE_CURVE('',#5024,#4898,#634,.T.);
#6393=EDGE_CURVE('',#5025,#4897,#635,.T.);
#6394=EDGE_CURVE('',#5023,#5026,#636,.T.);
#6395=EDGE_CURVE('',#5026,#4899,#637,.T.);
#6396=EDGE_CURVE('',#5026,#5024,#638,.T.);
#6397=EDGE_CURVE('',#4896,#5027,#639,.T.);
#6398=EDGE_CURVE('',#5027,#5025,#1494,.T.);
#6399=EDGE_CURVE('',#5028,#5029,#640,.T.);
#6400=EDGE_CURVE('',#5028,#4894,#641,.T.);
#6401=EDGE_CURVE('',#5029,#4973,#642,.T.);
#6402=EDGE_CURVE('',#5027,#5030,#643,.T.);
#6403=EDGE_CURVE('',#5030,#4895,#644,.T.);
#6404=EDGE_CURVE('',#5030,#5028,#645,.T.);
#6405=EDGE_CURVE('',#4972,#5031,#646,.T.);
#6406=EDGE_CURVE('',#5031,#5029,#1495,.T.);
#6407=EDGE_CURVE('',#5032,#5033,#647,.T.);
#6408=EDGE_CURVE('',#5032,#4970,#648,.T.);
#6409=EDGE_CURVE('',#5034,#4969,#649,.T.);
#6410=EDGE_CURVE('',#5033,#5034,#650,.T.);
#6411=EDGE_CURVE('',#5031,#5035,#651,.T.);
#6412=EDGE_CURVE('',#5035,#4971,#652,.T.);
#6413=EDGE_CURVE('',#5035,#5032,#653,.T.);
#6414=EDGE_CURVE('',#4968,#5036,#654,.T.);
#6415=EDGE_CURVE('',#5036,#5034,#1496,.T.);
#6416=EDGE_CURVE('',#5037,#5038,#655,.T.);
#6417=EDGE_CURVE('',#5037,#4966,#656,.T.);
#6418=EDGE_CURVE('',#5038,#4965,#657,.T.);
#6419=EDGE_CURVE('',#5036,#5039,#658,.T.);
#6420=EDGE_CURVE('',#5039,#4967,#659,.T.);
#6421=EDGE_CURVE('',#5039,#5037,#660,.T.);
#6422=EDGE_CURVE('',#4964,#5040,#661,.T.);
#6423=EDGE_CURVE('',#5040,#5038,#1497,.T.);
#6424=EDGE_CURVE('',#5041,#5042,#662,.T.);
#6425=EDGE_CURVE('',#5041,#4962,#663,.T.);
#6426=EDGE_CURVE('',#5042,#4961,#664,.T.);
#6427=EDGE_CURVE('',#5040,#5043,#665,.T.);
#6428=EDGE_CURVE('',#5043,#4963,#666,.T.);
#6429=EDGE_CURVE('',#5043,#5041,#667,.T.);
#6430=EDGE_CURVE('',#4960,#5044,#668,.T.);
#6431=EDGE_CURVE('',#5044,#5042,#1498,.T.);
#6432=EDGE_CURVE('',#5045,#5046,#669,.T.);
#6433=EDGE_CURVE('',#5045,#4958,#670,.T.);
#6434=EDGE_CURVE('',#5046,#4957,#671,.T.);
#6435=EDGE_CURVE('',#5044,#5047,#672,.T.);
#6436=EDGE_CURVE('',#5047,#4959,#673,.T.);
#6437=EDGE_CURVE('',#5047,#5045,#674,.T.);
#6438=EDGE_CURVE('',#4956,#5048,#675,.T.);
#6439=EDGE_CURVE('',#5048,#5046,#1499,.T.);
#6440=EDGE_CURVE('',#5049,#5050,#676,.T.);
#6441=EDGE_CURVE('',#5049,#4954,#677,.T.);
#6442=EDGE_CURVE('',#5050,#4953,#678,.T.);
#6443=EDGE_CURVE('',#5048,#5051,#679,.T.);
#6444=EDGE_CURVE('',#5051,#4955,#680,.T.);
#6445=EDGE_CURVE('',#5051,#5049,#681,.T.);
#6446=EDGE_CURVE('',#4952,#5052,#682,.T.);
#6447=EDGE_CURVE('',#5052,#5050,#1500,.T.);
#6448=EDGE_CURVE('',#5053,#5054,#683,.T.);
#6449=EDGE_CURVE('',#5053,#4950,#684,.T.);
#6450=EDGE_CURVE('',#5054,#4949,#685,.T.);
#6451=EDGE_CURVE('',#5052,#5055,#686,.T.);
#6452=EDGE_CURVE('',#5055,#4951,#687,.T.);
#6453=EDGE_CURVE('',#5055,#5053,#688,.T.);
#6454=EDGE_CURVE('',#4948,#5056,#689,.T.);
#6455=EDGE_CURVE('',#5056,#5054,#1501,.T.);
#6456=EDGE_CURVE('',#5057,#5058,#690,.T.);
#6457=EDGE_CURVE('',#5057,#4946,#691,.T.);
#6458=EDGE_CURVE('',#5058,#4945,#692,.T.);
#6459=EDGE_CURVE('',#5056,#5059,#693,.T.);
#6460=EDGE_CURVE('',#5059,#4947,#694,.T.);
#6461=EDGE_CURVE('',#5059,#5057,#695,.T.);
#6462=EDGE_CURVE('',#4944,#5060,#696,.T.);
#6463=EDGE_CURVE('',#5060,#5058,#1502,.T.);
#6464=EDGE_CURVE('',#5061,#5062,#697,.T.);
#6465=EDGE_CURVE('',#5061,#4942,#698,.T.);
#6466=EDGE_CURVE('',#5062,#4941,#699,.T.);
#6467=EDGE_CURVE('',#5060,#5063,#700,.T.);
#6468=EDGE_CURVE('',#5063,#4943,#701,.T.);
#6469=EDGE_CURVE('',#5063,#5061,#702,.T.);
#6470=EDGE_CURVE('',#4940,#5064,#703,.T.);
#6471=EDGE_CURVE('',#5064,#5062,#1503,.T.);
#6472=EDGE_CURVE('',#5065,#5066,#704,.T.);
#6473=EDGE_CURVE('',#5065,#4938,#705,.T.);
#6474=EDGE_CURVE('',#5066,#4937,#706,.T.);
#6475=EDGE_CURVE('',#5064,#5067,#707,.T.);
#6476=EDGE_CURVE('',#5067,#4939,#708,.T.);
#6477=EDGE_CURVE('',#5067,#5065,#709,.T.);
#6478=EDGE_CURVE('',#4936,#5068,#710,.T.);
#6479=EDGE_CURVE('',#5068,#5066,#1504,.T.);
#6480=EDGE_CURVE('',#5069,#4935,#711,.T.);
#6481=EDGE_CURVE('',#5068,#5069,#712,.T.);
#6482=EDGE_CURVE('',#5070,#4934,#713,.T.);
#6483=EDGE_CURVE('',#5069,#5070,#714,.T.);
#6484=EDGE_CURVE('',#5071,#4933,#715,.T.);
#6485=EDGE_CURVE('',#5070,#5071,#716,.T.);
#6486=EDGE_CURVE('',#5072,#4931,#717,.T.);
#6487=EDGE_CURVE('',#5073,#5072,#718,.T.);
#6488=EDGE_CURVE('',#4932,#5073,#719,.T.);
#6489=EDGE_CURVE('',#5074,#4930,#720,.T.);
#6490=EDGE_CURVE('',#5072,#5074,#721,.T.);
#6491=EDGE_CURVE('',#5074,#4998,#722,.T.);
#6492=EDGE_CURVE('',#5075,#5075,#1505,.T.);
#6493=EDGE_CURVE('',#5075,#5033,#3510,.T.);
#6494=EDGE_CURVE('',#5073,#5071,#1506,.T.);
#6495=EDGE_CURVE('',#5076,#5076,#1507,.T.);
#6496=EDGE_CURVE('',#5076,#5077,#3511,.T.);
#6497=EDGE_CURVE('',#5077,#5077,#1508,.T.);
#6498=EDGE_CURVE('',#5077,#5078,#3512,.T.);
#6499=EDGE_CURVE('',#5078,#5078,#1509,.T.);
#6500=EDGE_CURVE('',#5078,#5079,#3513,.T.);
#6501=EDGE_CURVE('',#5079,#5079,#1510,.T.);
#8411=ORIENTED_EDGE('',*,*,#6217,.T.);
#8412=ORIENTED_EDGE('',*,*,#6218,.T.);
#8413=ORIENTED_EDGE('',*,*,#6219,.T.);
#8414=ORIENTED_EDGE('',*,*,#6220,.T.);
#8415=ORIENTED_EDGE('',*,*,#6218,.F.);
#8416=ORIENTED_EDGE('',*,*,#6219,.F.);
#8417=ORIENTED_EDGE('',*,*,#6220,.F.);
#8418=ORIENTED_EDGE('',*,*,#6221,.T.);
#8419=ORIENTED_EDGE('',*,*,#6222,.T.);
#8420=ORIENTED_EDGE('',*,*,#6223,.T.);
#8421=ORIENTED_EDGE('',*,*,#6224,.T.);
#8422=ORIENTED_EDGE('',*,*,#6225,.T.);
#8423=ORIENTED_EDGE('',*,*,#6226,.T.);
#8424=ORIENTED_EDGE('',*,*,#6227,.T.);
#8425=ORIENTED_EDGE('',*,*,#6228,.T.);
#8426=ORIENTED_EDGE('',*,*,#6229,.T.);
#8427=ORIENTED_EDGE('',*,*,#6230,.T.);
#8428=ORIENTED_EDGE('',*,*,#6231,.T.);
#8429=ORIENTED_EDGE('',*,*,#6232,.T.);
#8430=ORIENTED_EDGE('',*,*,#6233,.T.);
#8431=ORIENTED_EDGE('',*,*,#6234,.T.);
#8432=ORIENTED_EDGE('',*,*,#6235,.T.);
#8433=ORIENTED_EDGE('',*,*,#6236,.T.);
#8434=ORIENTED_EDGE('',*,*,#6237,.T.);
#8435=ORIENTED_EDGE('',*,*,#6238,.T.);
#8436=ORIENTED_EDGE('',*,*,#6239,.T.);
#8437=ORIENTED_EDGE('',*,*,#6240,.T.);
#8438=ORIENTED_EDGE('',*,*,#6241,.T.);
#8439=ORIENTED_EDGE('',*,*,#6242,.T.);
#8440=ORIENTED_EDGE('',*,*,#6243,.T.);
#8441=ORIENTED_EDGE('',*,*,#6244,.T.);
#8442=ORIENTED_EDGE('',*,*,#6245,.T.);
#8443=ORIENTED_EDGE('',*,*,#6246,.T.);
#8444=ORIENTED_EDGE('',*,*,#6247,.T.);
#8445=ORIENTED_EDGE('',*,*,#6248,.T.);
#8446=ORIENTED_EDGE('',*,*,#6249,.T.);
#8447=ORIENTED_EDGE('',*,*,#6250,.T.);
#8448=ORIENTED_EDGE('',*,*,#6251,.T.);
#8449=ORIENTED_EDGE('',*,*,#6252,.T.);
#8450=ORIENTED_EDGE('',*,*,#6253,.T.);
#8451=ORIENTED_EDGE('',*,*,#6254,.T.);
#8452=ORIENTED_EDGE('',*,*,#6255,.T.);
#8453=ORIENTED_EDGE('',*,*,#6256,.T.);
#8454=ORIENTED_EDGE('',*,*,#6257,.T.);
#8455=ORIENTED_EDGE('',*,*,#6258,.T.);
#8456=ORIENTED_EDGE('',*,*,#6259,.T.);
#8457=ORIENTED_EDGE('',*,*,#6260,.T.);
#8458=ORIENTED_EDGE('',*,*,#6261,.T.);
#8459=ORIENTED_EDGE('',*,*,#6262,.T.);
#8460=ORIENTED_EDGE('',*,*,#6263,.T.);
#8461=ORIENTED_EDGE('',*,*,#6264,.T.);
#8462=ORIENTED_EDGE('',*,*,#6265,.T.);
#8463=ORIENTED_EDGE('',*,*,#6266,.T.);
#8464=ORIENTED_EDGE('',*,*,#6267,.T.);
#8465=ORIENTED_EDGE('',*,*,#6268,.T.);
#8466=ORIENTED_EDGE('',*,*,#6269,.T.);
#8467=ORIENTED_EDGE('',*,*,#6270,.T.);
#8468=ORIENTED_EDGE('',*,*,#6271,.T.);
#8469=ORIENTED_EDGE('',*,*,#6272,.T.);
#8470=ORIENTED_EDGE('',*,*,#6273,.T.);
#8471=ORIENTED_EDGE('',*,*,#6274,.T.);
#8472=ORIENTED_EDGE('',*,*,#6275,.T.);
#8473=ORIENTED_EDGE('',*,*,#6276,.T.);
#8474=ORIENTED_EDGE('',*,*,#6277,.T.);
#8475=ORIENTED_EDGE('',*,*,#6278,.T.);
#8476=ORIENTED_EDGE('',*,*,#6279,.T.);
#8477=ORIENTED_EDGE('',*,*,#6280,.T.);
#8478=ORIENTED_EDGE('',*,*,#6281,.T.);
#8479=ORIENTED_EDGE('',*,*,#6282,.T.);
#8480=ORIENTED_EDGE('',*,*,#6283,.T.);
#8481=ORIENTED_EDGE('',*,*,#6284,.T.);
#8482=ORIENTED_EDGE('',*,*,#6285,.T.);
#8483=ORIENTED_EDGE('',*,*,#6286,.T.);
#8484=ORIENTED_EDGE('',*,*,#6287,.T.);
#8485=ORIENTED_EDGE('',*,*,#6288,.T.);
#8486=ORIENTED_EDGE('',*,*,#6289,.T.);
#8487=ORIENTED_EDGE('',*,*,#6290,.T.);
#8488=ORIENTED_EDGE('',*,*,#6291,.T.);
#8489=ORIENTED_EDGE('',*,*,#6292,.T.);
#8490=ORIENTED_EDGE('',*,*,#6293,.T.);
#8491=ORIENTED_EDGE('',*,*,#6294,.T.);
#8492=ORIENTED_EDGE('',*,*,#6295,.T.);
#8493=ORIENTED_EDGE('',*,*,#6296,.T.);
#8494=ORIENTED_EDGE('',*,*,#6297,.T.);
#8495=ORIENTED_EDGE('',*,*,#6298,.T.);
#8496=ORIENTED_EDGE('',*,*,#6299,.T.);
#8497=ORIENTED_EDGE('',*,*,#6300,.T.);
#8498=ORIENTED_EDGE('',*,*,#6301,.T.);
#8499=ORIENTED_EDGE('',*,*,#6302,.T.);
#8500=ORIENTED_EDGE('',*,*,#6221,.F.);
#8501=ORIENTED_EDGE('',*,*,#6217,.F.);
#8502=ORIENTED_EDGE('',*,*,#6303,.F.);
#8503=ORIENTED_EDGE('',*,*,#6304,.T.);
#8504=ORIENTED_EDGE('',*,*,#6305,.F.);
#8505=ORIENTED_EDGE('',*,*,#6306,.T.);
#8506=ORIENTED_EDGE('',*,*,#6306,.F.);
#8507=ORIENTED_EDGE('',*,*,#6307,.T.);
#8508=ORIENTED_EDGE('',*,*,#6308,.T.);
#8509=ORIENTED_EDGE('',*,*,#6309,.T.);
#8510=ORIENTED_EDGE('',*,*,#6310,.T.);
#8511=ORIENTED_EDGE('',*,*,#6311,.T.);
#8512=ORIENTED_EDGE('',*,*,#6309,.F.);
#8513=ORIENTED_EDGE('',*,*,#6312,.T.);
#8514=ORIENTED_EDGE('',*,*,#6313,.T.);
#8515=ORIENTED_EDGE('',*,*,#6313,.F.);
#8516=ORIENTED_EDGE('',*,*,#6314,.F.);
#8517=ORIENTED_EDGE('',*,*,#6315,.F.);
#8518=ORIENTED_EDGE('',*,*,#6316,.F.);
#8519=ORIENTED_EDGE('',*,*,#6303,.T.);
#8520=ORIENTED_EDGE('',*,*,#6307,.F.);
#8521=ORIENTED_EDGE('',*,*,#6305,.T.);
#8522=ORIENTED_EDGE('',*,*,#6317,.F.);
#8523=ORIENTED_EDGE('',*,*,#6318,.F.);
#8524=ORIENTED_EDGE('',*,*,#6310,.F.);
#8525=ORIENTED_EDGE('',*,*,#6311,.F.);
#8526=ORIENTED_EDGE('',*,*,#6319,.T.);
#8527=ORIENTED_EDGE('',*,*,#6320,.F.);
#8528=ORIENTED_EDGE('',*,*,#6321,.F.);
#8529=ORIENTED_EDGE('',*,*,#6319,.F.);
#8530=ORIENTED_EDGE('',*,*,#6304,.F.);
#8531=ORIENTED_EDGE('',*,*,#6316,.T.);
#8532=ORIENTED_EDGE('',*,*,#6322,.T.);
#8533=ORIENTED_EDGE('',*,*,#6323,.T.);
#8534=ORIENTED_EDGE('',*,*,#6324,.T.);
#8535=ORIENTED_EDGE('',*,*,#6325,.T.);
#8536=ORIENTED_EDGE('',*,*,#6323,.F.);
#8537=ORIENTED_EDGE('',*,*,#6326,.T.);
#8538=ORIENTED_EDGE('',*,*,#6317,.T.);
#8539=ORIENTED_EDGE('',*,*,#6327,.F.);
#8540=ORIENTED_EDGE('',*,*,#6328,.F.);
#8541=ORIENTED_EDGE('',*,*,#6329,.T.);
#8542=ORIENTED_EDGE('',*,*,#6324,.F.);
#8543=ORIENTED_EDGE('',*,*,#6325,.F.);
#8544=ORIENTED_EDGE('',*,*,#6329,.F.);
#8545=ORIENTED_EDGE('',*,*,#6330,.F.);
#8546=ORIENTED_EDGE('',*,*,#6331,.T.);
#8547=ORIENTED_EDGE('',*,*,#6314,.T.);
#8548=ORIENTED_EDGE('',*,*,#6312,.F.);
#8549=ORIENTED_EDGE('',*,*,#6308,.F.);
#8550=ORIENTED_EDGE('',*,*,#6318,.T.);
#8551=ORIENTED_EDGE('',*,*,#6326,.F.);
#8552=ORIENTED_EDGE('',*,*,#6322,.F.);
#8553=ORIENTED_EDGE('',*,*,#6315,.T.);
#8554=ORIENTED_EDGE('',*,*,#6331,.F.);
#8555=ORIENTED_EDGE('',*,*,#6332,.F.);
#8556=ORIENTED_EDGE('',*,*,#6333,.T.);
#8557=ORIENTED_EDGE('',*,*,#6254,.F.);
#8558=ORIENTED_EDGE('',*,*,#6334,.F.);
#8559=ORIENTED_EDGE('',*,*,#6335,.F.);
#8560=ORIENTED_EDGE('',*,*,#6336,.F.);
#8561=ORIENTED_EDGE('',*,*,#6256,.F.);
#8562=ORIENTED_EDGE('',*,*,#6337,.F.);
#8563=ORIENTED_EDGE('',*,*,#6338,.F.);
#8564=ORIENTED_EDGE('',*,*,#6337,.T.);
#8565=ORIENTED_EDGE('',*,*,#6255,.F.);
#8566=ORIENTED_EDGE('',*,*,#6333,.F.);
#8567=ORIENTED_EDGE('',*,*,#6336,.T.);
#8568=ORIENTED_EDGE('',*,*,#6339,.T.);
#8569=ORIENTED_EDGE('',*,*,#6340,.T.);
#8570=ORIENTED_EDGE('',*,*,#6257,.F.);
#8571=ORIENTED_EDGE('',*,*,#6334,.T.);
#8572=ORIENTED_EDGE('',*,*,#6253,.F.);
#8573=ORIENTED_EDGE('',*,*,#6341,.T.);
#8574=ORIENTED_EDGE('',*,*,#6342,.T.);
#8575=ORIENTED_EDGE('',*,*,#6343,.F.);
#8576=ORIENTED_EDGE('',*,*,#6344,.T.);
#8577=ORIENTED_EDGE('',*,*,#6250,.F.);
#8578=ORIENTED_EDGE('',*,*,#6345,.F.);
#8579=ORIENTED_EDGE('',*,*,#6346,.F.);
#8580=ORIENTED_EDGE('',*,*,#6341,.F.);
#8581=ORIENTED_EDGE('',*,*,#6252,.F.);
#8582=ORIENTED_EDGE('',*,*,#6347,.F.);
#8583=ORIENTED_EDGE('',*,*,#6348,.F.);
#8584=ORIENTED_EDGE('',*,*,#6347,.T.);
#8585=ORIENTED_EDGE('',*,*,#6251,.F.);
#8586=ORIENTED_EDGE('',*,*,#6344,.F.);
#8587=ORIENTED_EDGE('',*,*,#6345,.T.);
#8588=ORIENTED_EDGE('',*,*,#6249,.F.);
#8589=ORIENTED_EDGE('',*,*,#6349,.T.);
#8590=ORIENTED_EDGE('',*,*,#6350,.T.);
#8591=ORIENTED_EDGE('',*,*,#6351,.F.);
#8592=ORIENTED_EDGE('',*,*,#6352,.T.);
#8593=ORIENTED_EDGE('',*,*,#6246,.F.);
#8594=ORIENTED_EDGE('',*,*,#6353,.F.);
#8595=ORIENTED_EDGE('',*,*,#6354,.F.);
#8596=ORIENTED_EDGE('',*,*,#6349,.F.);
#8597=ORIENTED_EDGE('',*,*,#6248,.F.);
#8598=ORIENTED_EDGE('',*,*,#6355,.F.);
#8599=ORIENTED_EDGE('',*,*,#6356,.F.);
#8600=ORIENTED_EDGE('',*,*,#6355,.T.);
#8601=ORIENTED_EDGE('',*,*,#6247,.F.);
#8602=ORIENTED_EDGE('',*,*,#6352,.F.);
#8603=ORIENTED_EDGE('',*,*,#6353,.T.);
#8604=ORIENTED_EDGE('',*,*,#6245,.F.);
#8605=ORIENTED_EDGE('',*,*,#6357,.T.);
#8606=ORIENTED_EDGE('',*,*,#6358,.T.);
#8607=ORIENTED_EDGE('',*,*,#6359,.F.);
#8608=ORIENTED_EDGE('',*,*,#6360,.T.);
#8609=ORIENTED_EDGE('',*,*,#6242,.F.);
#8610=ORIENTED_EDGE('',*,*,#6361,.F.);
#8611=ORIENTED_EDGE('',*,*,#6362,.F.);
#8612=ORIENTED_EDGE('',*,*,#6357,.F.);
#8613=ORIENTED_EDGE('',*,*,#6244,.F.);
#8614=ORIENTED_EDGE('',*,*,#6363,.F.);
#8615=ORIENTED_EDGE('',*,*,#6364,.F.);
#8616=ORIENTED_EDGE('',*,*,#6363,.T.);
#8617=ORIENTED_EDGE('',*,*,#6243,.F.);
#8618=ORIENTED_EDGE('',*,*,#6360,.F.);
#8619=ORIENTED_EDGE('',*,*,#6361,.T.);
#8620=ORIENTED_EDGE('',*,*,#6241,.F.);
#8621=ORIENTED_EDGE('',*,*,#6365,.T.);
#8622=ORIENTED_EDGE('',*,*,#6366,.T.);
#8623=ORIENTED_EDGE('',*,*,#6367,.F.);
#8624=ORIENTED_EDGE('',*,*,#6368,.T.);
#8625=ORIENTED_EDGE('',*,*,#6238,.F.);
#8626=ORIENTED_EDGE('',*,*,#6369,.F.);
#8627=ORIENTED_EDGE('',*,*,#6370,.F.);
#8628=ORIENTED_EDGE('',*,*,#6365,.F.);
#8629=ORIENTED_EDGE('',*,*,#6240,.F.);
#8630=ORIENTED_EDGE('',*,*,#6371,.F.);
#8631=ORIENTED_EDGE('',*,*,#6372,.F.);
#8632=ORIENTED_EDGE('',*,*,#6371,.T.);
#8633=ORIENTED_EDGE('',*,*,#6239,.F.);
#8634=ORIENTED_EDGE('',*,*,#6368,.F.);
#8635=ORIENTED_EDGE('',*,*,#6369,.T.);
#8636=ORIENTED_EDGE('',*,*,#6237,.F.);
#8637=ORIENTED_EDGE('',*,*,#6373,.T.);
#8638=ORIENTED_EDGE('',*,*,#6374,.T.);
#8639=ORIENTED_EDGE('',*,*,#6375,.F.);
#8640=ORIENTED_EDGE('',*,*,#6376,.T.);
#8641=ORIENTED_EDGE('',*,*,#6234,.F.);
#8642=ORIENTED_EDGE('',*,*,#6377,.F.);
#8643=ORIENTED_EDGE('',*,*,#6378,.F.);
#8644=ORIENTED_EDGE('',*,*,#6373,.F.);
#8645=ORIENTED_EDGE('',*,*,#6236,.F.);
#8646=ORIENTED_EDGE('',*,*,#6379,.F.);
#8647=ORIENTED_EDGE('',*,*,#6380,.F.);
#8648=ORIENTED_EDGE('',*,*,#6379,.T.);
#8649=ORIENTED_EDGE('',*,*,#6235,.F.);
#8650=ORIENTED_EDGE('',*,*,#6376,.F.);
#8651=ORIENTED_EDGE('',*,*,#6377,.T.);
#8652=ORIENTED_EDGE('',*,*,#6233,.F.);
#8653=ORIENTED_EDGE('',*,*,#6381,.T.);
#8654=ORIENTED_EDGE('',*,*,#6382,.T.);
#8655=ORIENTED_EDGE('',*,*,#6383,.F.);
#8656=ORIENTED_EDGE('',*,*,#6384,.T.);
#8657=ORIENTED_EDGE('',*,*,#6230,.F.);
#8658=ORIENTED_EDGE('',*,*,#6385,.F.);
#8659=ORIENTED_EDGE('',*,*,#6386,.F.);
#8660=ORIENTED_EDGE('',*,*,#6381,.F.);
#8661=ORIENTED_EDGE('',*,*,#6232,.F.);
#8662=ORIENTED_EDGE('',*,*,#6387,.F.);
#8663=ORIENTED_EDGE('',*,*,#6388,.F.);
#8664=ORIENTED_EDGE('',*,*,#6387,.T.);
#8665=ORIENTED_EDGE('',*,*,#6231,.F.);
#8666=ORIENTED_EDGE('',*,*,#6384,.F.);
#8667=ORIENTED_EDGE('',*,*,#6385,.T.);
#8668=ORIENTED_EDGE('',*,*,#6229,.F.);
#8669=ORIENTED_EDGE('',*,*,#6389,.T.);
#8670=ORIENTED_EDGE('',*,*,#6390,.T.);
#8671=ORIENTED_EDGE('',*,*,#6391,.F.);
#8672=ORIENTED_EDGE('',*,*,#6392,.T.);
#8673=ORIENTED_EDGE('',*,*,#6226,.F.);
#8674=ORIENTED_EDGE('',*,*,#6393,.F.);
#8675=ORIENTED_EDGE('',*,*,#6394,.F.);
#8676=ORIENTED_EDGE('',*,*,#6389,.F.);
#8677=ORIENTED_EDGE('',*,*,#6228,.F.);
#8678=ORIENTED_EDGE('',*,*,#6395,.F.);
#8679=ORIENTED_EDGE('',*,*,#6396,.F.);
#8680=ORIENTED_EDGE('',*,*,#6395,.T.);
#8681=ORIENTED_EDGE('',*,*,#6227,.F.);
#8682=ORIENTED_EDGE('',*,*,#6392,.F.);
#8683=ORIENTED_EDGE('',*,*,#6393,.T.);
#8684=ORIENTED_EDGE('',*,*,#6225,.F.);
#8685=ORIENTED_EDGE('',*,*,#6397,.T.);
#8686=ORIENTED_EDGE('',*,*,#6398,.T.);
#8687=ORIENTED_EDGE('',*,*,#6399,.F.);
#8688=ORIENTED_EDGE('',*,*,#6400,.T.);
#8689=ORIENTED_EDGE('',*,*,#6222,.F.);
#8690=ORIENTED_EDGE('',*,*,#6302,.F.);
#8691=ORIENTED_EDGE('',*,*,#6401,.F.);
#8692=ORIENTED_EDGE('',*,*,#6402,.F.);
#8693=ORIENTED_EDGE('',*,*,#6397,.F.);
#8694=ORIENTED_EDGE('',*,*,#6224,.F.);
#8695=ORIENTED_EDGE('',*,*,#6403,.F.);
#8696=ORIENTED_EDGE('',*,*,#6404,.F.);
#8697=ORIENTED_EDGE('',*,*,#6403,.T.);
#8698=ORIENTED_EDGE('',*,*,#6223,.F.);
#8699=ORIENTED_EDGE('',*,*,#6400,.F.);
#8700=ORIENTED_EDGE('',*,*,#6401,.T.);
#8701=ORIENTED_EDGE('',*,*,#6301,.F.);
#8702=ORIENTED_EDGE('',*,*,#6405,.T.);
#8703=ORIENTED_EDGE('',*,*,#6406,.T.);
#8704=ORIENTED_EDGE('',*,*,#6407,.F.);
#8705=ORIENTED_EDGE('',*,*,#6408,.T.);
#8706=ORIENTED_EDGE('',*,*,#6298,.F.);
#8707=ORIENTED_EDGE('',*,*,#6409,.F.);
#8708=ORIENTED_EDGE('',*,*,#6410,.F.);
#8709=ORIENTED_EDGE('',*,*,#6411,.F.);
#8710=ORIENTED_EDGE('',*,*,#6405,.F.);
#8711=ORIENTED_EDGE('',*,*,#6300,.F.);
#8712=ORIENTED_EDGE('',*,*,#6412,.F.);
#8713=ORIENTED_EDGE('',*,*,#6413,.F.);
#8714=ORIENTED_EDGE('',*,*,#6412,.T.);
#8715=ORIENTED_EDGE('',*,*,#6299,.F.);
#8716=ORIENTED_EDGE('',*,*,#6408,.F.);
#8717=ORIENTED_EDGE('',*,*,#6409,.T.);
#8718=ORIENTED_EDGE('',*,*,#6297,.F.);
#8719=ORIENTED_EDGE('',*,*,#6414,.T.);
#8720=ORIENTED_EDGE('',*,*,#6415,.T.);
#8721=ORIENTED_EDGE('',*,*,#6416,.F.);
#8722=ORIENTED_EDGE('',*,*,#6417,.T.);
#8723=ORIENTED_EDGE('',*,*,#6294,.F.);
#8724=ORIENTED_EDGE('',*,*,#6418,.F.);
#8725=ORIENTED_EDGE('',*,*,#6419,.F.);
#8726=ORIENTED_EDGE('',*,*,#6414,.F.);
#8727=ORIENTED_EDGE('',*,*,#6296,.F.);
#8728=ORIENTED_EDGE('',*,*,#6420,.F.);
#8729=ORIENTED_EDGE('',*,*,#6421,.F.);
#8730=ORIENTED_EDGE('',*,*,#6420,.T.);
#8731=ORIENTED_EDGE('',*,*,#6295,.F.);
#8732=ORIENTED_EDGE('',*,*,#6417,.F.);
#8733=ORIENTED_EDGE('',*,*,#6418,.T.);
#8734=ORIENTED_EDGE('',*,*,#6293,.F.);
#8735=ORIENTED_EDGE('',*,*,#6422,.T.);
#8736=ORIENTED_EDGE('',*,*,#6423,.T.);
#8737=ORIENTED_EDGE('',*,*,#6424,.F.);
#8738=ORIENTED_EDGE('',*,*,#6425,.T.);
#8739=ORIENTED_EDGE('',*,*,#6290,.F.);
#8740=ORIENTED_EDGE('',*,*,#6426,.F.);
#8741=ORIENTED_EDGE('',*,*,#6427,.F.);
#8742=ORIENTED_EDGE('',*,*,#6422,.F.);
#8743=ORIENTED_EDGE('',*,*,#6292,.F.);
#8744=ORIENTED_EDGE('',*,*,#6428,.F.);
#8745=ORIENTED_EDGE('',*,*,#6429,.F.);
#8746=ORIENTED_EDGE('',*,*,#6428,.T.);
#8747=ORIENTED_EDGE('',*,*,#6291,.F.);
#8748=ORIENTED_EDGE('',*,*,#6425,.F.);
#8749=ORIENTED_EDGE('',*,*,#6426,.T.);
#8750=ORIENTED_EDGE('',*,*,#6289,.F.);
#8751=ORIENTED_EDGE('',*,*,#6430,.T.);
#8752=ORIENTED_EDGE('',*,*,#6431,.T.);
#8753=ORIENTED_EDGE('',*,*,#6432,.F.);
#8754=ORIENTED_EDGE('',*,*,#6433,.T.);
#8755=ORIENTED_EDGE('',*,*,#6286,.F.);
#8756=ORIENTED_EDGE('',*,*,#6434,.F.);
#8757=ORIENTED_EDGE('',*,*,#6435,.F.);
#8758=ORIENTED_EDGE('',*,*,#6430,.F.);
#8759=ORIENTED_EDGE('',*,*,#6288,.F.);
#8760=ORIENTED_EDGE('',*,*,#6436,.F.);
#8761=ORIENTED_EDGE('',*,*,#6437,.F.);
#8762=ORIENTED_EDGE('',*,*,#6436,.T.);
#8763=ORIENTED_EDGE('',*,*,#6287,.F.);
#8764=ORIENTED_EDGE('',*,*,#6433,.F.);
#8765=ORIENTED_EDGE('',*,*,#6434,.T.);
#8766=ORIENTED_EDGE('',*,*,#6285,.F.);
#8767=ORIENTED_EDGE('',*,*,#6438,.T.);
#8768=ORIENTED_EDGE('',*,*,#6439,.T.);
#8769=ORIENTED_EDGE('',*,*,#6440,.F.);
#8770=ORIENTED_EDGE('',*,*,#6441,.T.);
#8771=ORIENTED_EDGE('',*,*,#6282,.F.);
#8772=ORIENTED_EDGE('',*,*,#6442,.F.);
#8773=ORIENTED_EDGE('',*,*,#6443,.F.);
#8774=ORIENTED_EDGE('',*,*,#6438,.F.);
#8775=ORIENTED_EDGE('',*,*,#6284,.F.);
#8776=ORIENTED_EDGE('',*,*,#6444,.F.);
#8777=ORIENTED_EDGE('',*,*,#6445,.F.);
#8778=ORIENTED_EDGE('',*,*,#6444,.T.);
#8779=ORIENTED_EDGE('',*,*,#6283,.F.);
#8780=ORIENTED_EDGE('',*,*,#6441,.F.);
#8781=ORIENTED_EDGE('',*,*,#6442,.T.);
#8782=ORIENTED_EDGE('',*,*,#6281,.F.);
#8783=ORIENTED_EDGE('',*,*,#6446,.T.);
#8784=ORIENTED_EDGE('',*,*,#6447,.T.);
#8785=ORIENTED_EDGE('',*,*,#6448,.F.);
#8786=ORIENTED_EDGE('',*,*,#6449,.T.);
#8787=ORIENTED_EDGE('',*,*,#6278,.F.);
#8788=ORIENTED_EDGE('',*,*,#6450,.F.);
#8789=ORIENTED_EDGE('',*,*,#6451,.F.);
#8790=ORIENTED_EDGE('',*,*,#6446,.F.);
#8791=ORIENTED_EDGE('',*,*,#6280,.F.);
#8792=ORIENTED_EDGE('',*,*,#6452,.F.);
#8793=ORIENTED_EDGE('',*,*,#6453,.F.);
#8794=ORIENTED_EDGE('',*,*,#6452,.T.);
#8795=ORIENTED_EDGE('',*,*,#6279,.F.);
#8796=ORIENTED_EDGE('',*,*,#6449,.F.);
#8797=ORIENTED_EDGE('',*,*,#6450,.T.);
#8798=ORIENTED_EDGE('',*,*,#6277,.F.);
#8799=ORIENTED_EDGE('',*,*,#6454,.T.);
#8800=ORIENTED_EDGE('',*,*,#6455,.T.);
#8801=ORIENTED_EDGE('',*,*,#6456,.F.);
#8802=ORIENTED_EDGE('',*,*,#6457,.T.);
#8803=ORIENTED_EDGE('',*,*,#6274,.F.);
#8804=ORIENTED_EDGE('',*,*,#6458,.F.);
#8805=ORIENTED_EDGE('',*,*,#6459,.F.);
#8806=ORIENTED_EDGE('',*,*,#6454,.F.);
#8807=ORIENTED_EDGE('',*,*,#6276,.F.);
#8808=ORIENTED_EDGE('',*,*,#6460,.F.);
#8809=ORIENTED_EDGE('',*,*,#6461,.F.);
#8810=ORIENTED_EDGE('',*,*,#6460,.T.);
#8811=ORIENTED_EDGE('',*,*,#6275,.F.);
#8812=ORIENTED_EDGE('',*,*,#6457,.F.);
#8813=ORIENTED_EDGE('',*,*,#6458,.T.);
#8814=ORIENTED_EDGE('',*,*,#6273,.F.);
#8815=ORIENTED_EDGE('',*,*,#6462,.T.);
#8816=ORIENTED_EDGE('',*,*,#6463,.T.);
#8817=ORIENTED_EDGE('',*,*,#6464,.F.);
#8818=ORIENTED_EDGE('',*,*,#6465,.T.);
#8819=ORIENTED_EDGE('',*,*,#6270,.F.);
#8820=ORIENTED_EDGE('',*,*,#6466,.F.);
#8821=ORIENTED_EDGE('',*,*,#6467,.F.);
#8822=ORIENTED_EDGE('',*,*,#6462,.F.);
#8823=ORIENTED_EDGE('',*,*,#6272,.F.);
#8824=ORIENTED_EDGE('',*,*,#6468,.F.);
#8825=ORIENTED_EDGE('',*,*,#6469,.F.);
#8826=ORIENTED_EDGE('',*,*,#6468,.T.);
#8827=ORIENTED_EDGE('',*,*,#6271,.F.);
#8828=ORIENTED_EDGE('',*,*,#6465,.F.);
#8829=ORIENTED_EDGE('',*,*,#6466,.T.);
#8830=ORIENTED_EDGE('',*,*,#6269,.F.);
#8831=ORIENTED_EDGE('',*,*,#6470,.T.);
#8832=ORIENTED_EDGE('',*,*,#6471,.T.);
#8833=ORIENTED_EDGE('',*,*,#6472,.F.);
#8834=ORIENTED_EDGE('',*,*,#6473,.T.);
#8835=ORIENTED_EDGE('',*,*,#6266,.F.);
#8836=ORIENTED_EDGE('',*,*,#6474,.F.);
#8837=ORIENTED_EDGE('',*,*,#6475,.F.);
#8838=ORIENTED_EDGE('',*,*,#6470,.F.);
#8839=ORIENTED_EDGE('',*,*,#6268,.F.);
#8840=ORIENTED_EDGE('',*,*,#6476,.F.);
#8841=ORIENTED_EDGE('',*,*,#6477,.F.);
#8842=ORIENTED_EDGE('',*,*,#6476,.T.);
#8843=ORIENTED_EDGE('',*,*,#6267,.F.);
#8844=ORIENTED_EDGE('',*,*,#6473,.F.);
#8845=ORIENTED_EDGE('',*,*,#6474,.T.);
#8846=ORIENTED_EDGE('',*,*,#6265,.F.);
#8847=ORIENTED_EDGE('',*,*,#6478,.T.);
#8848=ORIENTED_EDGE('',*,*,#6479,.T.);
#8849=ORIENTED_EDGE('',*,*,#6264,.F.);
#8850=ORIENTED_EDGE('',*,*,#6480,.F.);
#8851=ORIENTED_EDGE('',*,*,#6481,.F.);
#8852=ORIENTED_EDGE('',*,*,#6478,.F.);
#8853=ORIENTED_EDGE('',*,*,#6263,.F.);
#8854=ORIENTED_EDGE('',*,*,#6482,.F.);
#8855=ORIENTED_EDGE('',*,*,#6483,.F.);
#8856=ORIENTED_EDGE('',*,*,#6480,.T.);
#8857=ORIENTED_EDGE('',*,*,#6262,.F.);
#8858=ORIENTED_EDGE('',*,*,#6484,.F.);
#8859=ORIENTED_EDGE('',*,*,#6485,.F.);
#8860=ORIENTED_EDGE('',*,*,#6482,.T.);
#8861=ORIENTED_EDGE('',*,*,#6260,.F.);
#8862=ORIENTED_EDGE('',*,*,#6486,.F.);
#8863=ORIENTED_EDGE('',*,*,#6487,.F.);
#8864=ORIENTED_EDGE('',*,*,#6488,.F.);
#8865=ORIENTED_EDGE('',*,*,#6259,.F.);
#8866=ORIENTED_EDGE('',*,*,#6489,.F.);
#8867=ORIENTED_EDGE('',*,*,#6490,.F.);
#8868=ORIENTED_EDGE('',*,*,#6486,.T.);
#8869=ORIENTED_EDGE('',*,*,#6258,.F.);
#8870=ORIENTED_EDGE('',*,*,#6340,.F.);
#8871=ORIENTED_EDGE('',*,*,#6491,.F.);
#8872=ORIENTED_EDGE('',*,*,#6489,.T.);
#8873=ORIENTED_EDGE('',*,*,#6492,.T.);
#8874=ORIENTED_EDGE('',*,*,#6493,.T.);
#8875=ORIENTED_EDGE('',*,*,#6410,.T.);
#8876=ORIENTED_EDGE('',*,*,#6415,.F.);
#8877=ORIENTED_EDGE('',*,*,#6419,.T.);
#8878=ORIENTED_EDGE('',*,*,#6421,.T.);
#8879=ORIENTED_EDGE('',*,*,#6416,.T.);
#8880=ORIENTED_EDGE('',*,*,#6423,.F.);
#8881=ORIENTED_EDGE('',*,*,#6427,.T.);
#8882=ORIENTED_EDGE('',*,*,#6429,.T.);
#8883=ORIENTED_EDGE('',*,*,#6424,.T.);
#8884=ORIENTED_EDGE('',*,*,#6431,.F.);
#8885=ORIENTED_EDGE('',*,*,#6435,.T.);
#8886=ORIENTED_EDGE('',*,*,#6437,.T.);
#8887=ORIENTED_EDGE('',*,*,#6432,.T.);
#8888=ORIENTED_EDGE('',*,*,#6439,.F.);
#8889=ORIENTED_EDGE('',*,*,#6443,.T.);
#8890=ORIENTED_EDGE('',*,*,#6445,.T.);
#8891=ORIENTED_EDGE('',*,*,#6440,.T.);
#8892=ORIENTED_EDGE('',*,*,#6447,.F.);
#8893=ORIENTED_EDGE('',*,*,#6451,.T.);
#8894=ORIENTED_EDGE('',*,*,#6453,.T.);
#8895=ORIENTED_EDGE('',*,*,#6448,.T.);
#8896=ORIENTED_EDGE('',*,*,#6455,.F.);
#8897=ORIENTED_EDGE('',*,*,#6459,.T.);
#8898=ORIENTED_EDGE('',*,*,#6461,.T.);
#8899=ORIENTED_EDGE('',*,*,#6456,.T.);
#8900=ORIENTED_EDGE('',*,*,#6463,.F.);
#8901=ORIENTED_EDGE('',*,*,#6467,.T.);
#8902=ORIENTED_EDGE('',*,*,#6469,.T.);
#8903=ORIENTED_EDGE('',*,*,#6464,.T.);
#8904=ORIENTED_EDGE('',*,*,#6471,.F.);
#8905=ORIENTED_EDGE('',*,*,#6475,.T.);
#8906=ORIENTED_EDGE('',*,*,#6477,.T.);
#8907=ORIENTED_EDGE('',*,*,#6472,.T.);
#8908=ORIENTED_EDGE('',*,*,#6479,.F.);
#8909=ORIENTED_EDGE('',*,*,#6481,.T.);
#8910=ORIENTED_EDGE('',*,*,#6483,.T.);
#8911=ORIENTED_EDGE('',*,*,#6485,.T.);
#8912=ORIENTED_EDGE('',*,*,#6494,.F.);
#8913=ORIENTED_EDGE('',*,*,#6487,.T.);
#8914=ORIENTED_EDGE('',*,*,#6490,.T.);
#8915=ORIENTED_EDGE('',*,*,#6491,.T.);
#8916=ORIENTED_EDGE('',*,*,#6339,.F.);
#8917=ORIENTED_EDGE('',*,*,#6335,.T.);
#8918=ORIENTED_EDGE('',*,*,#6338,.T.);
#8919=ORIENTED_EDGE('',*,*,#6332,.T.);
#8920=ORIENTED_EDGE('',*,*,#6342,.F.);
#8921=ORIENTED_EDGE('',*,*,#6346,.T.);
#8922=ORIENTED_EDGE('',*,*,#6348,.T.);
#8923=ORIENTED_EDGE('',*,*,#6343,.T.);
#8924=ORIENTED_EDGE('',*,*,#6350,.F.);
#8925=ORIENTED_EDGE('',*,*,#6354,.T.);
#8926=ORIENTED_EDGE('',*,*,#6356,.T.);
#8927=ORIENTED_EDGE('',*,*,#6351,.T.);
#8928=ORIENTED_EDGE('',*,*,#6358,.F.);
#8929=ORIENTED_EDGE('',*,*,#6362,.T.);
#8930=ORIENTED_EDGE('',*,*,#6364,.T.);
#8931=ORIENTED_EDGE('',*,*,#6359,.T.);
#8932=ORIENTED_EDGE('',*,*,#6366,.F.);
#8933=ORIENTED_EDGE('',*,*,#6370,.T.);
#8934=ORIENTED_EDGE('',*,*,#6372,.T.);
#8935=ORIENTED_EDGE('',*,*,#6367,.T.);
#8936=ORIENTED_EDGE('',*,*,#6374,.F.);
#8937=ORIENTED_EDGE('',*,*,#6378,.T.);
#8938=ORIENTED_EDGE('',*,*,#6380,.T.);
#8939=ORIENTED_EDGE('',*,*,#6375,.T.);
#8940=ORIENTED_EDGE('',*,*,#6382,.F.);
#8941=ORIENTED_EDGE('',*,*,#6386,.T.);
#8942=ORIENTED_EDGE('',*,*,#6388,.T.);
#8943=ORIENTED_EDGE('',*,*,#6383,.T.);
#8944=ORIENTED_EDGE('',*,*,#6390,.F.);
#8945=ORIENTED_EDGE('',*,*,#6394,.T.);
#8946=ORIENTED_EDGE('',*,*,#6396,.T.);
#8947=ORIENTED_EDGE('',*,*,#6391,.T.);
#8948=ORIENTED_EDGE('',*,*,#6398,.F.);
#8949=ORIENTED_EDGE('',*,*,#6402,.T.);
#8950=ORIENTED_EDGE('',*,*,#6404,.T.);
#8951=ORIENTED_EDGE('',*,*,#6399,.T.);
#8952=ORIENTED_EDGE('',*,*,#6406,.F.);
#8953=ORIENTED_EDGE('',*,*,#6411,.T.);
#8954=ORIENTED_EDGE('',*,*,#6413,.T.);
#8955=ORIENTED_EDGE('',*,*,#6407,.T.);
#8956=ORIENTED_EDGE('',*,*,#6493,.F.);
#8957=ORIENTED_EDGE('',*,*,#6484,.T.);
#8958=ORIENTED_EDGE('',*,*,#6261,.F.);
#8959=ORIENTED_EDGE('',*,*,#6488,.T.);
#8960=ORIENTED_EDGE('',*,*,#6494,.T.);
#8961=ORIENTED_EDGE('',*,*,#6330,.T.);
#8962=ORIENTED_EDGE('',*,*,#6495,.F.);
#8963=ORIENTED_EDGE('',*,*,#6495,.T.);
#8964=ORIENTED_EDGE('',*,*,#6496,.T.);
#8965=ORIENTED_EDGE('',*,*,#6497,.F.);
#8966=ORIENTED_EDGE('',*,*,#6496,.F.);
#8967=ORIENTED_EDGE('',*,*,#6497,.T.);
#8968=ORIENTED_EDGE('',*,*,#6498,.T.);
#8969=ORIENTED_EDGE('',*,*,#6499,.F.);
#8970=ORIENTED_EDGE('',*,*,#6498,.F.);
#8971=ORIENTED_EDGE('',*,*,#6327,.T.);
#8972=ORIENTED_EDGE('',*,*,#6328,.T.);
#8973=ORIENTED_EDGE('',*,*,#6320,.T.);
#8974=ORIENTED_EDGE('',*,*,#6321,.T.);
#8975=ORIENTED_EDGE('',*,*,#6499,.T.);
#8976=ORIENTED_EDGE('',*,*,#6500,.T.);
#8977=ORIENTED_EDGE('',*,*,#6501,.F.);
#8978=ORIENTED_EDGE('',*,*,#6500,.F.);
#8979=ORIENTED_EDGE('',*,*,#6492,.F.);
#8980=ORIENTED_EDGE('',*,*,#6501,.T.);
#11557=PLANE('',#12802);
#11558=PLANE('',#12856);
#11559=PLANE('',#12864);
#11915=ADVANCED_FACE('',(#1948),#376,.T.);
#11916=ADVANCED_FACE('',(#1949),#377,.T.);
#11917=ADVANCED_FACE('',(#1950,#1360),#11557,.T.);
#11918=ADVANCED_FACE('',(#1951),#1206,.T.);
#11919=ADVANCED_FACE('',(#1952),#263,.T.);
#11920=ADVANCED_FACE('',(#1953),#264,.T.);
#11921=ADVANCED_FACE('',(#1954),#265,.F.);
#11922=ADVANCED_FACE('',(#1955),#1207,.T.);
#11923=ADVANCED_FACE('',(#1956),#266,.F.);
#11924=ADVANCED_FACE('',(#1957),#378,.T.);
#11925=ADVANCED_FACE('',(#1958),#1208,.F.);
#11926=ADVANCED_FACE('',(#1959),#1209,.F.);
#11927=ADVANCED_FACE('',(#1960),#1210,.F.);
#11928=ADVANCED_FACE('',(#1961),#379,.T.);
#11929=ADVANCED_FACE('',(#1962),#380,.T.);
#11930=ADVANCED_FACE('',(#1963),#1211,.F.);
#11931=ADVANCED_FACE('',(#1964),#1212,.F.);
#11932=ADVANCED_FACE('',(#1965),#1213,.F.);
#11933=ADVANCED_FACE('',(#1966),#381,.T.);
#11934=ADVANCED_FACE('',(#1967),#1214,.F.);
#11935=ADVANCED_FACE('',(#1968),#1215,.F.);
#11936=ADVANCED_FACE('',(#1969),#1216,.F.);
#11937=ADVANCED_FACE('',(#1970),#382,.T.);
#11938=ADVANCED_FACE('',(#1971),#1217,.F.);
#11939=ADVANCED_FACE('',(#1972),#1218,.F.);
#11940=ADVANCED_FACE('',(#1973),#1219,.F.);
#11941=ADVANCED_FACE('',(#1974),#383,.T.);
#11942=ADVANCED_FACE('',(#1975),#1220,.F.);
#11943=ADVANCED_FACE('',(#1976),#1221,.F.);
#11944=ADVANCED_FACE('',(#1977),#1222,.F.);
#11945=ADVANCED_FACE('',(#1978),#384,.T.);
#11946=ADVANCED_FACE('',(#1979),#1223,.F.);
#11947=ADVANCED_FACE('',(#1980),#1224,.F.);
#11948=ADVANCED_FACE('',(#1981),#1225,.F.);
#11949=ADVANCED_FACE('',(#1982),#385,.T.);
#11950=ADVANCED_FACE('',(#1983),#1226,.F.);
#11951=ADVANCED_FACE('',(#1984),#1227,.F.);
#11952=ADVANCED_FACE('',(#1985),#1228,.F.);
#11953=ADVANCED_FACE('',(#1986),#386,.T.);
#11954=ADVANCED_FACE('',(#1987),#1229,.F.);
#11955=ADVANCED_FACE('',(#1988),#1230,.F.);
#11956=ADVANCED_FACE('',(#1989),#1231,.F.);
#11957=ADVANCED_FACE('',(#1990),#387,.T.);
#11958=ADVANCED_FACE('',(#1991),#1232,.F.);
#11959=ADVANCED_FACE('',(#1992),#1233,.F.);
#11960=ADVANCED_FACE('',(#1993),#1234,.F.);
#11961=ADVANCED_FACE('',(#1994),#388,.T.);
#11962=ADVANCED_FACE('',(#1995),#1235,.F.);
#11963=ADVANCED_FACE('',(#1996),#1236,.F.);
#11964=ADVANCED_FACE('',(#1997),#1237,.F.);
#11965=ADVANCED_FACE('',(#1998),#389,.T.);
#11966=ADVANCED_FACE('',(#1999),#1238,.F.);
#11967=ADVANCED_FACE('',(#2000),#1239,.F.);
#11968=ADVANCED_FACE('',(#2001),#1240,.F.);
#11969=ADVANCED_FACE('',(#2002),#390,.T.);
#11970=ADVANCED_FACE('',(#2003),#1241,.F.);
#11971=ADVANCED_FACE('',(#2004),#1242,.F.);
#11972=ADVANCED_FACE('',(#2005),#1243,.F.);
#11973=ADVANCED_FACE('',(#2006),#391,.T.);
#11974=ADVANCED_FACE('',(#2007),#1244,.F.);
#11975=ADVANCED_FACE('',(#2008),#1245,.F.);
#11976=ADVANCED_FACE('',(#2009),#1246,.F.);
#11977=ADVANCED_FACE('',(#2010),#392,.T.);
#11978=ADVANCED_FACE('',(#2011),#1247,.F.);
#11979=ADVANCED_FACE('',(#2012),#1248,.F.);
#11980=ADVANCED_FACE('',(#2013),#1249,.F.);
#11981=ADVANCED_FACE('',(#2014),#393,.T.);
#11982=ADVANCED_FACE('',(#2015),#1250,.F.);
#11983=ADVANCED_FACE('',(#2016),#1251,.F.);
#11984=ADVANCED_FACE('',(#2017),#1252,.F.);
#11985=ADVANCED_FACE('',(#2018),#394,.T.);
#11986=ADVANCED_FACE('',(#2019),#1253,.F.);
#11987=ADVANCED_FACE('',(#2020),#1254,.F.);
#11988=ADVANCED_FACE('',(#2021),#1255,.F.);
#11989=ADVANCED_FACE('',(#2022),#395,.T.);
#11990=ADVANCED_FACE('',(#2023),#1256,.F.);
#11991=ADVANCED_FACE('',(#2024),#1257,.F.);
#11992=ADVANCED_FACE('',(#2025),#1258,.F.);
#11993=ADVANCED_FACE('',(#2026),#396,.T.);
#11994=ADVANCED_FACE('',(#2027),#1259,.F.);
#11995=ADVANCED_FACE('',(#2028),#1260,.F.);
#11996=ADVANCED_FACE('',(#2029),#1261,.F.);
#11997=ADVANCED_FACE('',(#2030),#397,.T.);
#11998=ADVANCED_FACE('',(#2031),#1262,.F.);
#11999=ADVANCED_FACE('',(#2032),#1263,.F.);
#12000=ADVANCED_FACE('',(#2033),#1264,.F.);
#12001=ADVANCED_FACE('',(#2034),#1265,.F.);
#12002=ADVANCED_FACE('',(#2035),#1266,.F.);
#12003=ADVANCED_FACE('',(#2036),#1267,.F.);
#12004=ADVANCED_FACE('',(#2037),#398,.F.);
#12005=ADVANCED_FACE('',(#2038),#399,.T.);
#12006=ADVANCED_FACE('',(#2039,#1361),#11558,.T.);
#12007=ADVANCED_FACE('',(#2040),#400,.F.);
#12008=ADVANCED_FACE('',(#2041,#1362,#1363),#267,.F.);
#12009=ADVANCED_FACE('',(#2042),#401,.F.);
#12010=ADVANCED_FACE('',(#2043,#1364),#11559,.T.);
#12481=CLOSED_SHELL('',(#11915,#11916,#11917,#11918,#11919,#11920,#11921,
#11922,#11923,#11924,#11925,#11926,#11927,#11928,#11929,#11930,#11931,#11932,
#11933,#11934,#11935,#11936,#11937,#11938,#11939,#11940,#11941,#11942,#11943,
#11944,#11945,#11946,#11947,#11948,#11949,#11950,#11951,#11952,#11953,#11954,
#11955,#11956,#11957,#11958,#11959,#11960,#11961,#11962,#11963,#11964,#11965,
#11966,#11967,#11968,#11969,#11970,#11971,#11972,#11973,#11974,#11975,#11976,
#11977,#11978,#11979,#11980,#11981,#11982,#11983,#11984,#11985,#11986,#11987,
#11988,#11989,#11990,#11991,#11992,#11993,#11994,#11995,#11996,#11997,#11998,
#11999,#12000,#12001,#12002,#12003,#12004,#12005,#12006,#12007,#12008,#12009,
#12010));
#12776=AXIS2_PLACEMENT_3D('',#17553,#14179,#14180);
#12777=AXIS2_PLACEMENT_3D('',#17554,#14181,#14182);
#12778=AXIS2_PLACEMENT_3D('',#17556,#14183,#14184);
#12779=AXIS2_PLACEMENT_3D('',#17560,#14186,#14187);
#12780=AXIS2_PLACEMENT_3D('',#17561,#14188,#14189);
#12781=AXIS2_PLACEMENT_3D('',#17562,#14190,#14191);
#12782=AXIS2_PLACEMENT_3D('',#17590,#14193,#14194);
#12783=AXIS2_PLACEMENT_3D('',#17616,#14195,#14196);
#12784=AXIS2_PLACEMENT_3D('',#17642,#14197,#14198);
#12785=AXIS2_PLACEMENT_3D('',#17668,#14199,#14200);
#12786=AXIS2_PLACEMENT_3D('',#17694,#14201,#14202);
#12787=AXIS2_PLACEMENT_3D('',#17720,#14203,#14204);
#12788=AXIS2_PLACEMENT_3D('',#17746,#14205,#14206);
#12789=AXIS2_PLACEMENT_3D('',#17772,#14207,#14208);
#12790=AXIS2_PLACEMENT_3D('',#17798,#14209,#14210);
#12791=AXIS2_PLACEMENT_3D('',#17824,#14211,#14212);
#12792=AXIS2_PLACEMENT_3D('',#17850,#14213,#14214);
#12793=AXIS2_PLACEMENT_3D('',#17876,#14215,#14216);
#12794=AXIS2_PLACEMENT_3D('',#17902,#14217,#14218);
#12795=AXIS2_PLACEMENT_3D('',#17928,#14219,#14220);
#12796=AXIS2_PLACEMENT_3D('',#17954,#14221,#14222);
#12797=AXIS2_PLACEMENT_3D('',#17980,#14223,#14224);
#12798=AXIS2_PLACEMENT_3D('',#18006,#14225,#14226);
#12799=AXIS2_PLACEMENT_3D('',#18032,#14227,#14228);
#12800=AXIS2_PLACEMENT_3D('',#18058,#14229,#14230);
#12801=AXIS2_PLACEMENT_3D('',#18084,#14231,#14232);
#12802=AXIS2_PLACEMENT_3D('',#18089,#14233,#14234);
#12803=AXIS2_PLACEMENT_3D('',#18092,#14235,#14236);
#12804=AXIS2_PLACEMENT_3D('',#18132,#14237,#14238);
#12805=AXIS2_PLACEMENT_3D('',#18379,#14239,#14240);
#12806=AXIS2_PLACEMENT_3D('',#18381,#14241,#14242);
#12807=AXIS2_PLACEMENT_3D('',#18383,#14243,#14244);
#12808=AXIS2_PLACEMENT_3D('',#18396,#14245,#14246);
#12809=AXIS2_PLACEMENT_3D('',#18412,#14247,#14248);
#12810=AXIS2_PLACEMENT_3D('',#18413,#14249,#14250);
#12811=AXIS2_PLACEMENT_3D('',#18630,#14252,#14253);
#12812=AXIS2_PLACEMENT_3D('',#18670,#14255,#14256);
#12813=AXIS2_PLACEMENT_3D('',#18672,#14257,#14258);
#12814=AXIS2_PLACEMENT_3D('',#18791,#14260,#14261);
#12815=AXIS2_PLACEMENT_3D('',#18793,#14262,#14263);
#12816=AXIS2_PLACEMENT_3D('',#18802,#14264,#14265);
#12817=AXIS2_PLACEMENT_3D('',#18812,#14266,#14267);
#12818=AXIS2_PLACEMENT_3D('',#18921,#14268,#14269);
#12819=AXIS2_PLACEMENT_3D('',#18931,#14270,#14271);
#12820=AXIS2_PLACEMENT_3D('',#19040,#14272,#14273);
#12821=AXIS2_PLACEMENT_3D('',#19050,#14274,#14275);
#12822=AXIS2_PLACEMENT_3D('',#19159,#14276,#14277);
#12823=AXIS2_PLACEMENT_3D('',#19169,#14278,#14279);
#12824=AXIS2_PLACEMENT_3D('',#19278,#14280,#14281);
#12825=AXIS2_PLACEMENT_3D('',#19288,#14282,#14283);
#12826=AXIS2_PLACEMENT_3D('',#19397,#14284,#14285);
#12827=AXIS2_PLACEMENT_3D('',#19407,#14286,#14287);
#12828=AXIS2_PLACEMENT_3D('',#19516,#14288,#14289);
#12829=AXIS2_PLACEMENT_3D('',#19526,#14290,#14291);
#12830=AXIS2_PLACEMENT_3D('',#19635,#14292,#14293);
#12831=AXIS2_PLACEMENT_3D('',#19645,#14294,#14295);
#12832=AXIS2_PLACEMENT_3D('',#19754,#14296,#14297);
#12833=AXIS2_PLACEMENT_3D('',#19764,#14298,#14299);
#12834=AXIS2_PLACEMENT_3D('',#19878,#14300,#14301);
#12835=AXIS2_PLACEMENT_3D('',#19888,#14302,#14303);
#12836=AXIS2_PLACEMENT_3D('',#19997,#14304,#14305);
#12837=AXIS2_PLACEMENT_3D('',#20007,#14306,#14307);
#12838=AXIS2_PLACEMENT_3D('',#20116,#14308,#14309);
#12839=AXIS2_PLACEMENT_3D('',#20126,#14310,#14311);
#12840=AXIS2_PLACEMENT_3D('',#20235,#14312,#14313);
#12841=AXIS2_PLACEMENT_3D('',#20245,#14314,#14315);
#12842=AXIS2_PLACEMENT_3D('',#20354,#14316,#14317);
#12843=AXIS2_PLACEMENT_3D('',#20364,#14318,#14319);
#12844=AXIS2_PLACEMENT_3D('',#20473,#14320,#14321);
#12845=AXIS2_PLACEMENT_3D('',#20483,#14322,#14323);
#12846=AXIS2_PLACEMENT_3D('',#20592,#14324,#14325);
#12847=AXIS2_PLACEMENT_3D('',#20602,#14326,#14327);
#12848=AXIS2_PLACEMENT_3D('',#20711,#14328,#14329);
#12849=AXIS2_PLACEMENT_3D('',#20721,#14330,#14331);
#12850=AXIS2_PLACEMENT_3D('',#20830,#14332,#14333);
#12851=AXIS2_PLACEMENT_3D('',#20840,#14334,#14335);
#12852=AXIS2_PLACEMENT_3D('',#21057,#14336,#14337);
#12853=AXIS2_PLACEMENT_3D('',#21059,#14338,#14339);
#12854=AXIS2_PLACEMENT_3D('',#21061,#14341,#14342);
#12855=AXIS2_PLACEMENT_3D('',#21062,#14343,#14344);
#12856=AXIS2_PLACEMENT_3D('',#21063,#14345,#14346);
#12857=AXIS2_PLACEMENT_3D('',#21065,#14347,#14348);
#12858=AXIS2_PLACEMENT_3D('',#21066,#14349,#14350);
#12859=AXIS2_PLACEMENT_3D('',#21069,#14352,#14353);
#12860=AXIS2_PLACEMENT_3D('',#21070,#14354,#14355);
#12861=AXIS2_PLACEMENT_3D('',#21073,#14357,#14358);
#12862=AXIS2_PLACEMENT_3D('',#21074,#14359,#14360);
#12863=AXIS2_PLACEMENT_3D('',#21077,#14362,#14363);
#12864=AXIS2_PLACEMENT_3D('',#21078,#14364,#14365);
#14179=DIRECTION('axis',(0.,0.,1.));
#14180=DIRECTION('refdir',(1.,0.,0.));
#14181=DIRECTION('center_axis',(0.,-2.48590929741675E-15,-1.));
#14182=DIRECTION('ref_axis',(-1.,-3.15543818946224E-17,0.));
#14183=DIRECTION('center_axis',(0.,0.,-1.));
#14184=DIRECTION('ref_axis',(-1.,0.,0.));
#14185=DIRECTION('',(0.923879532511287,-8.09021243661474E-16,-0.382683432365089));
#14186=DIRECTION('center_axis',(0.,0.,1.));
#14187=DIRECTION('ref_axis',(-1.,-6.12323399573677E-17,0.));
#14188=DIRECTION('center_axis',(0.,0.,1.));
#14189=DIRECTION('ref_axis',(-1.,-6.12323399573677E-17,0.));
#14190=DIRECTION('center_axis',(0.,0.,-1.));
#14191=DIRECTION('ref_axis',(1.,0.,0.));
#14192=DIRECTION('',(-0.707106781186548,-8.65956056235493E-17,-0.707106781186548));
#14193=DIRECTION('center_axis',(0.,0.,1.));
#14194=DIRECTION('ref_axis',(1.,0.,0.));
#14195=DIRECTION('center_axis',(0.,0.,1.));
#14196=DIRECTION('ref_axis',(1.,0.,0.));
#14197=DIRECTION('center_axis',(0.,0.,1.));
#14198=DIRECTION('ref_axis',(1.,0.,0.));
#14199=DIRECTION('center_axis',(0.,0.,1.));
#14200=DIRECTION('ref_axis',(1.,0.,0.));
#14201=DIRECTION('center_axis',(0.,0.,1.));
#14202=DIRECTION('ref_axis',(1.,0.,0.));
#14203=DIRECTION('center_axis',(0.,0.,1.));
#14204=DIRECTION('ref_axis',(1.,0.,0.));
#14205=DIRECTION('center_axis',(0.,0.,1.));
#14206=DIRECTION('ref_axis',(1.,0.,0.));
#14207=DIRECTION('center_axis',(0.,0.,1.));
#14208=DIRECTION('ref_axis',(1.,0.,0.));
#14209=DIRECTION('center_axis',(0.,0.,1.));
#14210=DIRECTION('ref_axis',(1.,0.,0.));
#14211=DIRECTION('center_axis',(0.,0.,1.));
#14212=DIRECTION('ref_axis',(1.,0.,0.));
#14213=DIRECTION('center_axis',(0.,0.,1.));
#14214=DIRECTION('ref_axis',(1.,0.,0.));
#14215=DIRECTION('center_axis',(0.,0.,1.));
#14216=DIRECTION('ref_axis',(1.,0.,0.));
#14217=DIRECTION('center_axis',(0.,0.,1.));
#14218=DIRECTION('ref_axis',(1.,0.,0.));
#14219=DIRECTION('center_axis',(0.,0.,1.));
#14220=DIRECTION('ref_axis',(1.,0.,0.));
#14221=DIRECTION('center_axis',(0.,0.,1.));
#14222=DIRECTION('ref_axis',(1.,0.,0.));
#14223=DIRECTION('center_axis',(0.,0.,1.));
#14224=DIRECTION('ref_axis',(1.,0.,0.));
#14225=DIRECTION('center_axis',(0.,0.,1.));
#14226=DIRECTION('ref_axis',(1.,0.,0.));
#14227=DIRECTION('center_axis',(0.,0.,1.));
#14228=DIRECTION('ref_axis',(1.,0.,0.));
#14229=DIRECTION('center_axis',(0.,0.,1.));
#14230=DIRECTION('ref_axis',(1.,0.,0.));
#14231=DIRECTION('center_axis',(0.,0.,1.));
#14232=DIRECTION('ref_axis',(1.,0.,0.));
#14233=DIRECTION('center_axis',(0.,0.,1.));
#14234=DIRECTION('ref_axis',(1.,0.,0.));
#14235=DIRECTION('center_axis',(0.,0.,1.));
#14236=DIRECTION('ref_axis',(1.,0.,0.));
#14237=DIRECTION('center_axis',(0.,0.,1.));
#14238=DIRECTION('ref_axis',(1.,0.,0.));
#14239=DIRECTION('center_axis',(0.,0.,1.));
#14240=DIRECTION('ref_axis',(-0.707106781186547,-0.707106781186548,0.));
#14241=DIRECTION('center_axis',(0.,0.,1.));
#14242=DIRECTION('ref_axis',(1.,0.,0.));
#14243=DIRECTION('center_axis',(0.,0.,1.));
#14244=DIRECTION('ref_axis',(1.,0.,0.));
#14245=DIRECTION('center_axis',(0.,0.,1.));
#14246=DIRECTION('ref_axis',(1.,0.,0.));
#14247=DIRECTION('center_axis',(0.,0.,1.));
#14248=DIRECTION('ref_axis',(1.,0.,0.));
#14249=DIRECTION('center_axis',(-1.,0.,0.));
#14250=DIRECTION('ref_axis',(0.,0.,1.));
#14251=DIRECTION('',(-1.,0.,0.));
#14252=DIRECTION('center_axis',(6.12323399573677E-17,1.,0.));
#14253=DIRECTION('ref_axis',(1.7303891563162E-32,0.,1.));
#14254=DIRECTION('',(6.12323399573677E-17,1.,0.));
#14255=DIRECTION('center_axis',(0.,0.,-1.));
#14256=DIRECTION('ref_axis',(1.,0.,0.));
#14257=DIRECTION('center_axis',(0.,0.,1.));
#14258=DIRECTION('ref_axis',(1.,0.,0.));
#14259=DIRECTION('',(-0.707106781186546,-8.65956056235491E-17,-0.707106781186549));
#14260=DIRECTION('center_axis',(0.,0.,1.));
#14261=DIRECTION('ref_axis',(1.,0.,0.));
#14262=DIRECTION('center_axis',(0.,0.,1.));
#14263=DIRECTION('ref_axis',(1.,0.,0.));
#14264=DIRECTION('center_axis',(0.,0.,1.));
#14265=DIRECTION('ref_axis',(1.,0.,0.));
#14266=DIRECTION('center_axis',(0.,0.,1.));
#14267=DIRECTION('ref_axis',(1.,0.,0.));
#14268=DIRECTION('center_axis',(0.,0.,1.));
#14269=DIRECTION('ref_axis',(1.,0.,0.));
#14270=DIRECTION('center_axis',(0.,0.,1.));
#14271=DIRECTION('ref_axis',(1.,0.,0.));
#14272=DIRECTION('center_axis',(0.,0.,1.));
#14273=DIRECTION('ref_axis',(1.,0.,0.));
#14274=DIRECTION('center_axis',(0.,0.,1.));
#14275=DIRECTION('ref_axis',(1.,0.,0.));
#14276=DIRECTION('center_axis',(0.,0.,1.));
#14277=DIRECTION('ref_axis',(1.,0.,0.));
#14278=DIRECTION('center_axis',(0.,0.,1.));
#14279=DIRECTION('ref_axis',(1.,0.,0.));
#14280=DIRECTION('center_axis',(0.,0.,1.));
#14281=DIRECTION('ref_axis',(1.,0.,0.));
#14282=DIRECTION('center_axis',(0.,0.,1.));
#14283=DIRECTION('ref_axis',(1.,0.,0.));
#14284=DIRECTION('center_axis',(0.,0.,1.));
#14285=DIRECTION('ref_axis',(1.,0.,0.));
#14286=DIRECTION('center_axis',(0.,0.,1.));
#14287=DIRECTION('ref_axis',(1.,0.,0.));
#14288=DIRECTION('center_axis',(0.,0.,1.));
#14289=DIRECTION('ref_axis',(1.,0.,0.));
#14290=DIRECTION('center_axis',(0.,0.,1.));
#14291=DIRECTION('ref_axis',(1.,0.,0.));
#14292=DIRECTION('center_axis',(0.,0.,1.));
#14293=DIRECTION('ref_axis',(1.,0.,0.));
#14294=DIRECTION('center_axis',(0.,0.,1.));
#14295=DIRECTION('ref_axis',(1.,0.,0.));
#14296=DIRECTION('center_axis',(0.,0.,1.));
#14297=DIRECTION('ref_axis',(-0.994427391317185,-0.105423732613193,0.));
#14298=DIRECTION('center_axis',(0.,0.,1.));
#14299=DIRECTION('ref_axis',(1.,0.,0.));
#14300=DIRECTION('center_axis',(0.,0.,1.));
#14301=DIRECTION('ref_axis',(1.,0.,0.));
#14302=DIRECTION('center_axis',(0.,0.,1.));
#14303=DIRECTION('ref_axis',(1.,0.,0.));
#14304=DIRECTION('center_axis',(0.,0.,1.));
#14305=DIRECTION('ref_axis',(1.,0.,0.));
#14306=DIRECTION('center_axis',(0.,0.,1.));
#14307=DIRECTION('ref_axis',(1.,0.,0.));
#14308=DIRECTION('center_axis',(0.,0.,1.));
#14309=DIRECTION('ref_axis',(1.,0.,0.));
#14310=DIRECTION('center_axis',(0.,0.,1.));
#14311=DIRECTION('ref_axis',(1.,0.,0.));
#14312=DIRECTION('center_axis',(0.,0.,1.));
#14313=DIRECTION('ref_axis',(1.,0.,0.));
#14314=DIRECTION('center_axis',(0.,0.,1.));
#14315=DIRECTION('ref_axis',(1.,0.,0.));
#14316=DIRECTION('center_axis',(0.,0.,1.));
#14317=DIRECTION('ref_axis',(1.,0.,0.));
#14318=DIRECTION('center_axis',(0.,0.,1.));
#14319=DIRECTION('ref_axis',(1.,0.,0.));
#14320=DIRECTION('center_axis',(0.,0.,1.));
#14321=DIRECTION('ref_axis',(1.,0.,0.));
#14322=DIRECTION('center_axis',(0.,0.,1.));
#14323=DIRECTION('ref_axis',(1.,0.,0.));
#14324=DIRECTION('center_axis',(0.,0.,1.));
#14325=DIRECTION('ref_axis',(1.,0.,0.));
#14326=DIRECTION('center_axis',(0.,0.,1.));
#14327=DIRECTION('ref_axis',(1.,0.,0.));
#14328=DIRECTION('center_axis',(0.,0.,1.));
#14329=DIRECTION('ref_axis',(1.,0.,0.));
#14330=DIRECTION('center_axis',(0.,0.,1.));
#14331=DIRECTION('ref_axis',(1.,0.,0.));
#14332=DIRECTION('center_axis',(0.,0.,1.));
#14333=DIRECTION('ref_axis',(1.,0.,0.));
#14334=DIRECTION('center_axis',(0.,0.,1.));
#14335=DIRECTION('ref_axis',(1.,0.,0.));
#14336=DIRECTION('center_axis',(0.,0.,-1.));
#14337=DIRECTION('ref_axis',(1.,0.,0.));
#14338=DIRECTION('center_axis',(0.,0.,1.));
#14339=DIRECTION('ref_axis',(1.,0.,0.));
#14340=DIRECTION('',(-0.707106781186548,-8.65956056235493E-17,-0.707106781186548));
#14341=DIRECTION('center_axis',(0.,0.,1.));
#14342=DIRECTION('ref_axis',(1.,0.,0.));
#14343=DIRECTION('center_axis',(0.,0.,1.));
#14344=DIRECTION('ref_axis',(1.,0.,0.));
#14345=DIRECTION('center_axis',(0.,0.,1.));
#14346=DIRECTION('ref_axis',(1.,0.,0.));
#14347=DIRECTION('center_axis',(0.,0.,1.));
#14348=DIRECTION('ref_axis',(1.,0.,0.));
#14349=DIRECTION('center_axis',(0.,0.,1.));
#14350=DIRECTION('ref_axis',(1.,0.,0.));
#14351=DIRECTION('',(0.707106781186547,8.65956056235493E-17,-0.707106781186547));
#14352=DIRECTION('center_axis',(0.,0.,1.));
#14353=DIRECTION('ref_axis',(1.,0.,0.));
#14354=DIRECTION('center_axis',(0.,0.,1.));
#14355=DIRECTION('ref_axis',(1.,0.,0.));
#14356=DIRECTION('',(0.,0.,-1.));
#14357=DIRECTION('center_axis',(0.,0.,1.));
#14358=DIRECTION('ref_axis',(1.,0.,0.));
#14359=DIRECTION('center_axis',(0.,0.,-1.));
#14360=DIRECTION('ref_axis',(1.,0.,0.));
#14361=DIRECTION('',(-0.70710678118655,-8.65956056235496E-17,-0.707106781186545));
#14362=DIRECTION('center_axis',(0.,0.,1.));
#14363=DIRECTION('ref_axis',(1.,0.,0.));
#14364=DIRECTION('center_axis',(0.,0.,-1.));
#14365=DIRECTION('ref_axis',(-1.,0.,0.));
#17553=CARTESIAN_POINT('',(0.,0.,0.));
#17554=CARTESIAN_POINT('Origin',(0.,-4.39450830404517E-17,2.08232233047034));
#17555=CARTESIAN_POINT('',(1.35,-1.65327317884893E-16,2.1));
#17556=CARTESIAN_POINT('Origin',(0.,0.,2.1));
#17557=CARTESIAN_POINT('',(1.43535533905933,1.75780332161807E-16,2.06464466094067));
#17558=CARTESIAN_POINT('',(1.39267766952966,1.7055382502335E-16,2.08232233047034));
#17559=CARTESIAN_POINT('',(-1.43535533905933,-1.75780332161807E-16,2.06464466094067));
#17560=CARTESIAN_POINT('Origin',(0.,-8.78901660809035E-17,2.06464466094067));
#17561=CARTESIAN_POINT('Origin',(0.,-8.78901660809035E-17,2.06464466094067));
#17562=CARTESIAN_POINT('Origin',(0.,0.,1.86807790411448));
#17563=CARTESIAN_POINT('',(-1.82153560215913,6.70435414410743E-13,1.67846439784087));
#17564=CARTESIAN_POINT('',(-1.63192209588552,-1.99852817118404E-16,1.86807790411448));
#17565=CARTESIAN_POINT('',(-1.58980227845634,-0.0690572297370878,1.90869858745619));
#17566=CARTESIAN_POINT('Ctrl Pts',(-1.82153560215913,1.34132982498869E-12,
1.67846439784087));
#17567=CARTESIAN_POINT('Ctrl Pts',(-1.79844488399902,-0.0142452763777164,
1.70155511600098));
#17568=CARTESIAN_POINT('Ctrl Pts',(-1.77621769100022,-0.0263518482108029,
1.7236179719196));
#17569=CARTESIAN_POINT('Ctrl Pts',(-1.73494412567812,-0.0458782640980182,
1.76447740749199));
#17570=CARTESIAN_POINT('Ctrl Pts',(-1.70513299984439,-0.0588876017641377,
1.79387050688965));
#17571=CARTESIAN_POINT('Ctrl Pts',(-1.65153927195835,-0.0709952547837174,
1.84694613619239));
#17572=CARTESIAN_POINT('Ctrl Pts',(-1.62431631612136,-0.0738960377458574,
1.87400707649559));
#17573=CARTESIAN_POINT('Ctrl Pts',(-1.58980227845634,-0.0690572297370876,
1.90869858745619));
#17574=CARTESIAN_POINT('',(-1.5699559447672,-0.259766273896473,1.90869858745619));
#17575=CARTESIAN_POINT('Ctrl Pts',(-1.58980227845634,-0.0690572297370881,
1.90869858745619));
#17576=CARTESIAN_POINT('Ctrl Pts',(-1.58741971380287,-0.10016208146902,
1.90972905962805));
#17577=CARTESIAN_POINT('Ctrl Pts',(-1.58467291856134,-0.131250509699782,
1.91020759537532));
#17578=CARTESIAN_POINT('Ctrl Pts',(-1.58148476202963,-0.162313364909724,
1.91020766105751));
#17579=CARTESIAN_POINT('Ctrl Pts',(-1.57814413491694,-0.194861771890304,
1.91020772988089));
#17580=CARTESIAN_POINT('Ctrl Pts',(-1.57432303476077,-0.227345240254554,
1.90968253191571));
#17581=CARTESIAN_POINT('Ctrl Pts',(-1.5699559447672,-0.259766273896472,
1.90869858745619));
#17582=CARTESIAN_POINT('',(-1.81394816223928,-0.428377445609996,1.63615580822897));
#17583=CARTESIAN_POINT('Ctrl Pts',(-1.5699559447672,-0.259766273896473,
1.90869858745619));
#17584=CARTESIAN_POINT('Ctrl Pts',(-1.61720542751897,-0.262319849600338,
1.86166605258312));
#17585=CARTESIAN_POINT('Ctrl Pts',(-1.6527385648653,-0.277648859152455,
1.82419649030025));
#17586=CARTESIAN_POINT('Ctrl Pts',(-1.72174825233757,-0.325349196383375,
1.74786428230184));
#17587=CARTESIAN_POINT('Ctrl Pts',(-1.76741714130056,-0.365195041946486,
1.69596272615694));
#17588=CARTESIAN_POINT('Ctrl Pts',(-1.81394816223928,-0.428377445609996,
1.63615580822897));
#17589=CARTESIAN_POINT('',(-1.78098192700405,-0.549562141057365,1.63615580822897));
#17590=CARTESIAN_POINT('Origin',(0.,0.,1.63615580822897));
#17591=CARTESIAN_POINT('',(-1.49065195897357,-0.55695325007777,1.90869858745619));
#17592=CARTESIAN_POINT('Ctrl Pts',(-1.78098192700405,-0.549562141057365,
1.63615580822897));
#17593=CARTESIAN_POINT('Ctrl Pts',(-1.73615378095071,-0.563182934028249,
1.67497485013899));
#17594=CARTESIAN_POINT('Ctrl Pts',(-1.69503929836625,-0.572158425678775,
1.71107791524196));
#17595=CARTESIAN_POINT('Ctrl Pts',(-1.63585275285353,-0.579760041152499,
1.76447740749373));
#17596=CARTESIAN_POINT('Ctrl Pts',(-1.60348058094793,-0.582920512008146,
1.79387050689049));
#17597=CARTESIAN_POINT('Ctrl Pts',(-1.54876844626294,-0.577874201600641,
1.84694613619458));
#17598=CARTESIAN_POINT('Ctrl Pts',(-1.52198148548954,-0.572220654147733,
1.87400707649755));
#17599=CARTESIAN_POINT('Ctrl Pts',(-1.49065195897357,-0.55695325007777,
1.90869858745619));
#17600=CARTESIAN_POINT('',(-1.41284463836769,-0.732195474855993,1.90869858745619));
#17601=CARTESIAN_POINT('Ctrl Pts',(-1.49065195897357,-0.556953250077769,
1.90869858745619));
#17602=CARTESIAN_POINT('Ctrl Pts',(-1.47877407754171,-0.585799469037713,
1.90972905962805));
#17603=CARTESIAN_POINT('Ctrl Pts',(-1.4665548673766,-0.614517514878265,
1.91020759537532));
#17604=CARTESIAN_POINT('Ctrl Pts',(-1.45392380017848,-0.643074851191362,
1.91020766105751));
#17605=CARTESIAN_POINT('Ctrl Pts',(-1.44068866409761,-0.672997915195582,
1.91020772988089));
#17606=CARTESIAN_POINT('Ctrl Pts',(-1.42701663813388,-0.702710744569809,
1.90968253191571));
#17607=CARTESIAN_POINT('Ctrl Pts',(-1.41284463836769,-0.732195474855993,
1.90869858745619));
#17608=CARTESIAN_POINT('',(-1.59279130921887,-0.967951970128403,1.63615580822897));
#17609=CARTESIAN_POINT('Ctrl Pts',(-1.41284463836769,-0.732195474855993,
1.90869858745619));
#17610=CARTESIAN_POINT('Ctrl Pts',(-1.45699246854074,-0.74922496281447,
1.86166605258385));
#17611=CARTESIAN_POINT('Ctrl Pts',(-1.48604956590001,-0.774784060540386,
1.82419649030103));
#17612=CARTESIAN_POINT('Ctrl Pts',(-1.53694146401283,-0.841474943294401,
1.74786428230768));
#17613=CARTESIAN_POINT('Ctrl Pts',(-1.56806211502062,-0.893483057166951,
1.69596272616206));
#17614=CARTESIAN_POINT('Ctrl Pts',(-1.59279130921887,-0.967951970128403,
1.63615580822897));
#17615=CARTESIAN_POINT('',(-1.5239904260293,-1.07301833748062,1.63615580822897));
#17616=CARTESIAN_POINT('Origin',(0.,0.,1.63615580822897));
#17617=CARTESIAN_POINT('',(-1.24558623976356,-0.990330805779365,1.90869858745619));
#17618=CARTESIAN_POINT('Ctrl Pts',(-1.5239904260293,-1.07301833748062,1.63615580822897));
#17619=CARTESIAN_POINT('Ctrl Pts',(-1.47714726910887,-1.07211982243591,
1.67497485013742));
#17620=CARTESIAN_POINT('Ctrl Pts',(-1.43527149308025,-1.06795094842396,
1.71107791523994));
#17621=CARTESIAN_POINT('Ctrl Pts',(-1.37663271492071,-1.05689086595159,
1.76447740749771));
#17622=CARTESIAN_POINT('Ctrl Pts',(-1.34486831068169,-1.04989310109001,
1.79387050689188));
#17623=CARTESIAN_POINT('Ctrl Pts',(-1.29439337414606,-1.02818679527844,
1.8469461361937));
#17624=CARTESIAN_POINT('Ctrl Pts',(-1.27066450279186,-1.01453232602662,
1.87400707649691));
#17625=CARTESIAN_POINT('Ctrl Pts',(-1.24558623976356,-0.990330805779365,
1.90869858745619));
#17626=CARTESIAN_POINT('',(-1.11743425489732,-1.13295228123076,1.90869858745619));
#17627=CARTESIAN_POINT('Ctrl Pts',(-1.24558623976356,-0.990330805779365,
1.90869858745619));
#17628=CARTESIAN_POINT('Ctrl Pts',(-1.22537573134593,-1.01409472307207,
1.90972905962805));
#17629=CARTESIAN_POINT('Ctrl Pts',(-1.20488020768447,-1.03763126410513,
1.91020759537532));
#17630=CARTESIAN_POINT('Ctrl Pts',(-1.18404264668309,-1.06088769047244,
1.91020766105751));
#17631=CARTESIAN_POINT('Ctrl Pts',(-1.16220854896825,-1.08525633350931,
1.91020772988089));
#17632=CARTESIAN_POINT('Ctrl Pts',(-1.14002391035689,-1.1092900251329,1.90968253191571));
#17633=CARTESIAN_POINT('Ctrl Pts',(-1.11743425489732,-1.13295228123076,
1.90869858745619));
#17634=CARTESIAN_POINT('',(-1.21572094522251,-1.4127766116927,1.63615580822897));
#17635=CARTESIAN_POINT('Ctrl Pts',(-1.11743425489733,-1.13295228123076,
1.90869858745619));
#17636=CARTESIAN_POINT('Ctrl Pts',(-1.15415893527728,-1.16279071650968,
1.86166605258608));
#17637=CARTESIAN_POINT('Ctrl Pts',(-1.17389568150815,-1.19607799984267,
1.82419649030342));
#17638=CARTESIAN_POINT('Ctrl Pts',(-1.20168813669714,-1.27523125986505,
1.74786428230159));
#17639=CARTESIAN_POINT('Ctrl Pts',(-1.21521424359529,-1.33431072550216,
1.69596272615648));
#17640=CARTESIAN_POINT('Ctrl Pts',(-1.21572094522251,-1.4127766116927,1.63615580822897));
#17641=CARTESIAN_POINT('',(-1.11782012388912,-1.4914400228729,1.63615580822897));
#17642=CARTESIAN_POINT('Origin',(0.,0.,1.63615580822897));
#17643=CARTESIAN_POINT('',(-0.878593860895847,-1.32676788217082,1.90869858745619));
#17644=CARTESIAN_POINT('Ctrl Pts',(-1.11782012388912,-1.4914400228729,1.63615580822897));
#17645=CARTESIAN_POINT('Ctrl Pts',(-1.07354729067195,-1.47611015272513,
1.67497485013978));
#17646=CARTESIAN_POINT('Ctrl Pts',(-1.03500931392296,-1.45920499148488,
1.71107791524182));
#17647=CARTESIAN_POINT('Ctrl Pts',(-0.982658275295231,-1.43056584900102,
1.76447740749414));
#17648=CARTESIAN_POINT('Ctrl Pts',(-0.954610959919589,-1.41409483840259,
1.79387050689094));
#17649=CARTESIAN_POINT('Ctrl Pts',(-0.913314059997475,-1.37785330163525,
1.84694613619429));
#17650=CARTESIAN_POINT('Ctrl Pts',(-0.894966025319891,-1.35753450517084,
1.87400707649751));
#17651=CARTESIAN_POINT('Ctrl Pts',(-0.878593860895848,-1.32676788217082,
1.90869858745619));
#17652=CARTESIAN_POINT('',(-0.712641620935351,-1.42280782457595,1.90869858745619));
#17653=CARTESIAN_POINT('Ctrl Pts',(-0.878593860895848,-1.32676788217082,
1.90869858745619));
#17654=CARTESIAN_POINT('Ctrl Pts',(-0.852029070871246,-1.34312331999875,
1.90972905962805));
#17655=CARTESIAN_POINT('Ctrl Pts',(-0.8252634783701,-1.35917443559929,1.91020759537532));
#17656=CARTESIAN_POINT('Ctrl Pts',(-0.798259149220139,-1.37485345097089,
1.91020766105751));
#17657=CARTESIAN_POINT('Ctrl Pts',(-0.769963363482765,-1.39128230047366,
1.91020772988089));
#17658=CARTESIAN_POINT('Ctrl Pts',(-0.741437699220515,-1.40728426915793,
1.9096825319157));
#17659=CARTESIAN_POINT('Ctrl Pts',(-0.712641620935351,-1.42280782457595,
1.90869858745619));
#17660=CARTESIAN_POINT('',(-0.719647344681869,-1.71930883511106,1.63615580822897));
#17661=CARTESIAN_POINT('Ctrl Pts',(-0.712641620935352,-1.42280782457595,
1.90869858745619));
#17662=CARTESIAN_POINT('Ctrl Pts',(-0.738348283935276,-1.4625344132382,
1.8616660525816));
#17663=CARTESIAN_POINT('Ctrl Pts',(-0.746832708799745,-1.5002914909622,
1.82419649029873));
#17664=CARTESIAN_POINT('Ctrl Pts',(-0.748805201903997,-1.58415905565693,
1.74786428230083));
#17665=CARTESIAN_POINT('Ctrl Pts',(-0.743412735108965,-1.64452676332901,
1.69596272615631));
#17666=CARTESIAN_POINT('Ctrl Pts',(-0.719647344681869,-1.71930883511106,
1.63615580822897));
#17667=CARTESIAN_POINT('',(-0.602229799711922,-1.76386916735271,1.63615580822897));
#17668=CARTESIAN_POINT('Origin',(0.,0.,1.63615580822897));
#17669=CARTESIAN_POINT('',(-0.425598593400272,-1.53333167412,1.90869858745619));
#17670=CARTESIAN_POINT('Ctrl Pts',(-0.602229799711921,-1.76386916735271,
1.63615580822897));
#17671=CARTESIAN_POINT('Ctrl Pts',(-0.56486102358392,-1.73560853660211,
1.67497485013891));
#17672=CARTESIAN_POINT('Ctrl Pts',(-0.533433211787428,-1.70762188310109,
1.71107791524129));
#17673=CARTESIAN_POINT('Ctrl Pts',(-0.492494397097019,-1.664207079411,1.7644774074943));
#17674=CARTESIAN_POINT('Ctrl Pts',(-0.470909637234242,-1.63987512035428,
1.79387050689047));
#17675=CARTESIAN_POINT('Ctrl Pts',(-0.442833202224615,-1.5926459267614,
1.84694613619249));
#17676=CARTESIAN_POINT('Ctrl Pts',(-0.431662037695392,-1.56765174845206,
1.87400707649573));
#17677=CARTESIAN_POINT('Ctrl Pts',(-0.425598593400271,-1.53333167412,1.90869858745619));
#17678=CARTESIAN_POINT('',(-0.238090659850088,-1.57338902476662,1.90869858745619));
#17679=CARTESIAN_POINT('Ctrl Pts',(-0.425598593400272,-1.53333167412,1.90869858745619));
#17680=CARTESIAN_POINT('Ctrl Pts',(-0.395279868504098,-1.5406776482735,
1.90972905962805));
#17681=CARTESIAN_POINT('Ctrl Pts',(-0.364864209844148,-1.54767214341183,
1.91020759537532));
#17682=CARTESIAN_POINT('Ctrl Pts',(-0.334336484432989,-1.55423897652106,
1.91020766105751));
#17683=CARTESIAN_POINT('Ctrl Pts',(-0.302348799329381,-1.56111986223385,
1.91020772988089));
#17684=CARTESIAN_POINT('Ctrl Pts',(-0.270274400184222,-1.56752372379171,
1.9096825319157));
#17685=CARTESIAN_POINT('Ctrl Pts',(-0.238090659850088,-1.57338902476662,
1.90869858745619));
#17686=CARTESIAN_POINT('',(-0.153129647965883,-1.85754313061971,1.63615580822897));
#17687=CARTESIAN_POINT('Ctrl Pts',(-0.238090659850089,-1.57338902476662,
1.90869858745619));
#17688=CARTESIAN_POINT('Ctrl Pts',(-0.25026295818307,-1.61911505151921,
1.86166605258207));
#17689=CARTESIAN_POINT('Ctrl Pts',(-0.246664547063089,-1.6576459977954,
1.82419649029927));
#17690=CARTESIAN_POINT('Ctrl Pts',(-0.226553376416707,-1.72488162993613,
1.76034062848752));
#17691=CARTESIAN_POINT('Ctrl Pts',(-0.206497613058332,-1.78308197878352,
1.70598062725551));
#17692=CARTESIAN_POINT('Ctrl Pts',(-0.153129647965884,-1.85754313061971,
1.63615580822897));
#17693=CARTESIAN_POINT('',(-0.0276890267571698,-1.86363850813291,1.63615580822897));
#17694=CARTESIAN_POINT('Origin',(0.,0.,1.63615580822897));
#17695=CARTESIAN_POINT('',(0.0690572297370874,-1.58980227845634,1.90869858745619));
#17696=CARTESIAN_POINT('Ctrl Pts',(-0.0276890267571705,-1.86363850813291,
1.63615580822897));
#17697=CARTESIAN_POINT('Ctrl Pts',(-0.000882223887656915,-1.82521346421937,
1.67497485013994));
#17698=CARTESIAN_POINT('Ctrl Pts',(0.0203590497666264,-1.78888484709669,
1.71107791524241));
#17699=CARTESIAN_POINT('Ctrl Pts',(0.0458782640980426,-1.73494412567807,
1.76447740749204));
#17700=CARTESIAN_POINT('Ctrl Pts',(0.0588876017641393,-1.70513299984438,
1.79387050688965));
#17701=CARTESIAN_POINT('Ctrl Pts',(0.0709952547834971,-1.65153927195932,
1.84694613619142));
#17702=CARTESIAN_POINT('Ctrl Pts',(0.0738960377459689,-1.62431631612213,
1.87400707649481));
#17703=CARTESIAN_POINT('Ctrl Pts',(0.0690572297370878,-1.58980227845634,
1.90869858745619));
#17704=CARTESIAN_POINT('',(0.259766273896473,-1.5699559447672,1.90869858745619));
#17705=CARTESIAN_POINT('Ctrl Pts',(0.0690572297370876,-1.58980227845634,
1.90869858745619));
#17706=CARTESIAN_POINT('Ctrl Pts',(0.100162081469028,-1.58741971380287,
1.90972905962805));
#17707=CARTESIAN_POINT('Ctrl Pts',(0.131250509699797,-1.58467291856134,
1.91020759537532));
#17708=CARTESIAN_POINT('Ctrl Pts',(0.162313364909724,-1.58148476202963,
1.91020766105751));
#17709=CARTESIAN_POINT('Ctrl Pts',(0.194861771890304,-1.57814413491694,
1.91020772988089));
#17710=CARTESIAN_POINT('Ctrl Pts',(0.227345240254553,-1.57432303476077,
1.90968253191571));
#17711=CARTESIAN_POINT('Ctrl Pts',(0.259766273896472,-1.5699559447672,1.90869858745619));
#17712=CARTESIAN_POINT('',(0.428377445609996,-1.81394816223928,1.63615580822897));
#17713=CARTESIAN_POINT('Ctrl Pts',(0.259766273896472,-1.5699559447672,1.90869858745619));
#17714=CARTESIAN_POINT('Ctrl Pts',(0.262319849600408,-1.61720542752026,
1.86166605258184));
#17715=CARTESIAN_POINT('Ctrl Pts',(0.277648859153229,-1.65273856486642,
1.824196490299));
#17716=CARTESIAN_POINT('Ctrl Pts',(0.325349196385585,-1.72174825234076,
1.74786428229831));
#17717=CARTESIAN_POINT('Ctrl Pts',(0.365195041949575,-1.76741714130283,
1.69596272615402));
#17718=CARTESIAN_POINT('Ctrl Pts',(0.428377445609996,-1.81394816223928,
1.63615580822897));
#17719=CARTESIAN_POINT('',(0.549562141057364,-1.78098192700405,1.63615580822897));
#17720=CARTESIAN_POINT('Origin',(0.,0.,1.63615580822897));
#17721=CARTESIAN_POINT('',(0.556953250077769,-1.49065195897357,1.90869858745619));
#17722=CARTESIAN_POINT('Ctrl Pts',(0.549562141057365,-1.78098192700405,
1.63615580822897));
#17723=CARTESIAN_POINT('Ctrl Pts',(0.563182934028143,-1.73615378095104,
1.6749748501387));
#17724=CARTESIAN_POINT('Ctrl Pts',(0.572158425678644,-1.69503929836728,
1.71107791524103));
#17725=CARTESIAN_POINT('Ctrl Pts',(0.579760041152732,-1.63585275285171,
1.76447740749537));
#17726=CARTESIAN_POINT('Ctrl Pts',(0.582920512008082,-1.60348058094729,
1.79387050689112));
#17727=CARTESIAN_POINT('Ctrl Pts',(0.577874201600642,-1.54876844626293,
1.84694613619459));
#17728=CARTESIAN_POINT('Ctrl Pts',(0.572220654147706,-1.52198148548948,
1.87400707649761));
#17729=CARTESIAN_POINT('Ctrl Pts',(0.556953250077769,-1.49065195897357,
1.90869858745619));
#17730=CARTESIAN_POINT('',(0.732195474855992,-1.41284463836769,1.90869858745619));
#17731=CARTESIAN_POINT('Ctrl Pts',(0.556953250077769,-1.49065195897357,
1.90869858745619));
#17732=CARTESIAN_POINT('Ctrl Pts',(0.585799469037704,-1.47877407754171,
1.90972905962805));
#17733=CARTESIAN_POINT('Ctrl Pts',(0.614517514878248,-1.46655486737661,
1.91020759537532));
#17734=CARTESIAN_POINT('Ctrl Pts',(0.643074851191361,-1.45392380017848,
1.91020766105751));
#17735=CARTESIAN_POINT('Ctrl Pts',(0.672997915195573,-1.44068866409761,
1.91020772988089));
#17736=CARTESIAN_POINT('Ctrl Pts',(0.702710744569794,-1.42701663813388,
1.90968253191571));
#17737=CARTESIAN_POINT('Ctrl Pts',(0.732195474855992,-1.41284463836769,
1.90869858745619));
#17738=CARTESIAN_POINT('',(0.967951970128402,-1.59279130921887,1.63615580822897));
#17739=CARTESIAN_POINT('Ctrl Pts',(0.732195474855992,-1.41284463836769,
1.90869858745619));
#17740=CARTESIAN_POINT('Ctrl Pts',(0.749224962814994,-1.4569924685421,1.8616660525824));
#17741=CARTESIAN_POINT('Ctrl Pts',(0.774784060541701,-1.48604956590099,
1.82419649029954));
#17742=CARTESIAN_POINT('Ctrl Pts',(0.841474943298512,-1.53694146401599,
1.74786428230295));
#17743=CARTESIAN_POINT('Ctrl Pts',(0.893483057171948,-1.56806211502227,
1.69596272615805));
#17744=CARTESIAN_POINT('Ctrl Pts',(0.967951970128402,-1.59279130921887,
1.63615580822897));
#17745=CARTESIAN_POINT('',(1.07301833748062,-1.52399042602929,1.63615580822897));
#17746=CARTESIAN_POINT('Origin',(0.,0.,1.63615580822897));
#17747=CARTESIAN_POINT('',(0.990330805779365,-1.24558623976355,1.90869858745619));
#17748=CARTESIAN_POINT('Ctrl Pts',(1.07301833748062,-1.52399042602929,1.63615580822897));
#17749=CARTESIAN_POINT('Ctrl Pts',(1.07211982243578,-1.4771472691025,1.6749748501427));
#17750=CARTESIAN_POINT('Ctrl Pts',(1.06795094842305,-1.43527149307552,1.71107791524426));
#17751=CARTESIAN_POINT('Ctrl Pts',(1.05689086595362,-1.37663271493145,1.76447740748792));
#17752=CARTESIAN_POINT('Ctrl Pts',(1.04989310109149,-1.34486831068513,1.79387050688826));
#17753=CARTESIAN_POINT('Ctrl Pts',(1.0281867952793,-1.29439337414807,1.8469461361916));
#17754=CARTESIAN_POINT('Ctrl Pts',(1.01453232602804,-1.27066450279334,1.87400707649487));
#17755=CARTESIAN_POINT('Ctrl Pts',(0.990330805779366,-1.24558623976355,
1.90869858745619));
#17756=CARTESIAN_POINT('',(1.13295228123076,-1.11743425489732,1.90869858745619));
#17757=CARTESIAN_POINT('Ctrl Pts',(0.990330805779366,-1.24558623976355,
1.90869858745619));
#17758=CARTESIAN_POINT('Ctrl Pts',(1.01409472307207,-1.22537573134593,1.90972905962805));
#17759=CARTESIAN_POINT('Ctrl Pts',(1.03763126410513,-1.20488020768447,1.91020759537532));
#17760=CARTESIAN_POINT('Ctrl Pts',(1.06088769047244,-1.18404264668309,1.91020766105751));
#17761=CARTESIAN_POINT('Ctrl Pts',(1.08525633350931,-1.16220854896825,1.91020772988089));
#17762=CARTESIAN_POINT('Ctrl Pts',(1.1092900251329,-1.14002391035689,1.90968253191571));
#17763=CARTESIAN_POINT('Ctrl Pts',(1.13295228123076,-1.11743425489732,1.90869858745619));
#17764=CARTESIAN_POINT('',(1.4127766116927,-1.21572094522251,1.63615580822897));
#17765=CARTESIAN_POINT('Ctrl Pts',(1.13295228123076,-1.11743425489733,1.90869858745619));
#17766=CARTESIAN_POINT('Ctrl Pts',(1.16279071651073,-1.15415893527858,1.86166605258442));
#17767=CARTESIAN_POINT('Ctrl Pts',(1.19607799984447,-1.17389568150877,1.82419649030168));
#17768=CARTESIAN_POINT('Ctrl Pts',(1.27523125986793,-1.20168813669816,1.74786428229881));
#17769=CARTESIAN_POINT('Ctrl Pts',(1.33431072550509,-1.2152142435953,1.69596272615425));
#17770=CARTESIAN_POINT('Ctrl Pts',(1.4127766116927,-1.21572094522251,1.63615580822897));
#17771=CARTESIAN_POINT('',(1.4914400228729,-1.11782012388912,1.63615580822897));
#17772=CARTESIAN_POINT('Origin',(0.,0.,1.63615580822897));
#17773=CARTESIAN_POINT('',(1.32676788217082,-0.878593860895847,1.90869858745619));
#17774=CARTESIAN_POINT('Ctrl Pts',(1.4914400228729,-1.11782012388912,1.63615580822897));
#17775=CARTESIAN_POINT('Ctrl Pts',(1.47611015272491,-1.07354729067132,1.67497485014032));
#17776=CARTESIAN_POINT('Ctrl Pts',(1.45920499148449,-1.03500931392226,1.71107791524254));
#17777=CARTESIAN_POINT('Ctrl Pts',(1.43056584900227,-0.9826582752975,1.76447740749182));
#17778=CARTESIAN_POINT('Ctrl Pts',(1.41409483840349,-0.954610959920599,
1.79387050688963));
#17779=CARTESIAN_POINT('Ctrl Pts',(1.37785330163609,-0.913314059998434,
1.84694613619306));
#17780=CARTESIAN_POINT('Ctrl Pts',(1.35753450517206,-0.894966025320543,
1.87400707649614));
#17781=CARTESIAN_POINT('Ctrl Pts',(1.32676788217082,-0.878593860895848,
1.90869858745619));
#17782=CARTESIAN_POINT('',(1.42280782457595,-0.712641620935351,1.90869858745619));
#17783=CARTESIAN_POINT('Ctrl Pts',(1.32676788217082,-0.878593860895847,
1.90869858745619));
#17784=CARTESIAN_POINT('Ctrl Pts',(1.34312331999875,-0.852029070871249,
1.90972905962805));
#17785=CARTESIAN_POINT('Ctrl Pts',(1.35917443559929,-0.825263478370106,
1.91020759537532));
#17786=CARTESIAN_POINT('Ctrl Pts',(1.37485345097089,-0.798259149220139,
1.91020766105751));
#17787=CARTESIAN_POINT('Ctrl Pts',(1.39128230047366,-0.769963363482759,
1.91020772988089));
#17788=CARTESIAN_POINT('Ctrl Pts',(1.40728426915793,-0.741437699220503,
1.9096825319157));
#17789=CARTESIAN_POINT('Ctrl Pts',(1.42280782457595,-0.712641620935351,
1.90869858745619));
#17790=CARTESIAN_POINT('',(1.71930883511106,-0.719647344681869,1.63615580822897));
#17791=CARTESIAN_POINT('Ctrl Pts',(1.42280782457595,-0.712641620935352,
1.90869858745619));
#17792=CARTESIAN_POINT('Ctrl Pts',(1.46253441323553,-0.738348283933551,
1.86166605258476));
#17793=CARTESIAN_POINT('Ctrl Pts',(1.50029149095869,-0.746832708799665,
1.82419649030192));
#17794=CARTESIAN_POINT('Ctrl Pts',(1.5841590556494,-0.748805201903815,1.74786428230768));
#17795=CARTESIAN_POINT('Ctrl Pts',(1.64452676332205,-0.743412735111191,
1.69596272616187));
#17796=CARTESIAN_POINT('Ctrl Pts',(1.71930883511106,-0.719647344681869,
1.63615580822897));
#17797=CARTESIAN_POINT('',(1.76386916735271,-0.602229799711922,1.63615580822897));
#17798=CARTESIAN_POINT('Origin',(0.,0.,1.63615580822897));
#17799=CARTESIAN_POINT('',(1.53333167412,-0.425598593400271,1.90869858745619));
#17800=CARTESIAN_POINT('Ctrl Pts',(1.76386916735271,-0.602229799711921,
1.63615580822897));
#17801=CARTESIAN_POINT('Ctrl Pts',(1.73560853660213,-0.564861023583931,
1.6749748501389));
#17802=CARTESIAN_POINT('Ctrl Pts',(1.7076218831011,-0.533433211787444,1.71107791524128));
#17803=CARTESIAN_POINT('Ctrl Pts',(1.66420707941097,-0.492494397096992,
1.76447740749434));
#17804=CARTESIAN_POINT('Ctrl Pts',(1.6398751203543,-0.470909637234254,1.79387050689044));
#17805=CARTESIAN_POINT('Ctrl Pts',(1.59264592676154,-0.442833202224699,
1.84694613619233));
#17806=CARTESIAN_POINT('Ctrl Pts',(1.56765174845221,-0.431662037695425,
1.87400707649557));
#17807=CARTESIAN_POINT('Ctrl Pts',(1.53333167412,-0.425598593400271,1.90869858745619));
#17808=CARTESIAN_POINT('',(1.57338902476662,-0.238090659850088,1.90869858745619));
#17809=CARTESIAN_POINT('Ctrl Pts',(1.53333167412,-0.425598593400272,1.90869858745619));
#17810=CARTESIAN_POINT('Ctrl Pts',(1.54067764827351,-0.395279868504085,
1.90972905962805));
#17811=CARTESIAN_POINT('Ctrl Pts',(1.54767214341184,-0.364864209844123,
1.91020759537532));
#17812=CARTESIAN_POINT('Ctrl Pts',(1.55423897652106,-0.334336484432989,
1.91020766105751));
#17813=CARTESIAN_POINT('Ctrl Pts',(1.56111986223385,-0.302348799329382,
1.91020772988089));
#17814=CARTESIAN_POINT('Ctrl Pts',(1.56752372379171,-0.270274400184223,
1.9096825319157));
#17815=CARTESIAN_POINT('Ctrl Pts',(1.57338902476662,-0.238090659850088,
1.90869858745619));
#17816=CARTESIAN_POINT('',(1.85754313061971,-0.153129647965884,1.63615580822897));
#17817=CARTESIAN_POINT('Ctrl Pts',(1.57338902476662,-0.238090659850088,
1.90869858745619));
#17818=CARTESIAN_POINT('Ctrl Pts',(1.61911505151656,-0.250262958182363,
1.8616660525848));
#17819=CARTESIAN_POINT('Ctrl Pts',(1.65764599779255,-0.246664547063935,
1.82419649030197));
#17820=CARTESIAN_POINT('Ctrl Pts',(1.72488162993741,-0.226553376416327,
1.7603406284863));
#17821=CARTESIAN_POINT('Ctrl Pts',(1.78308197878428,-0.206497613057801,
1.70598062725479));
#17822=CARTESIAN_POINT('Ctrl Pts',(1.85754313061971,-0.153129647965883,
1.63615580822897));
#17823=CARTESIAN_POINT('',(1.86363850813291,-0.0276890267571702,1.63615580822897));
#17824=CARTESIAN_POINT('Origin',(0.,0.,1.63615580822897));
#17825=CARTESIAN_POINT('',(1.58980227845634,0.0690572297370882,1.90869858745619));
#17826=CARTESIAN_POINT('Ctrl Pts',(1.86363850813291,-0.0276890267571701,
1.63615580822897));
#17827=CARTESIAN_POINT('Ctrl Pts',(1.82521346421932,-0.0008822238876082,
1.67497485014));
#17828=CARTESIAN_POINT('Ctrl Pts',(1.788884847097,0.0203590497664785,1.7110779152421));
#17829=CARTESIAN_POINT('Ctrl Pts',(1.73494412567664,0.045878264098721,1.76447740749345));
#17830=CARTESIAN_POINT('Ctrl Pts',(1.70513299984346,0.0588876017643422,
1.79387050689057));
#17831=CARTESIAN_POINT('Ctrl Pts',(1.6515392719567,0.0709952547840949,1.84694613619402));
#17832=CARTESIAN_POINT('Ctrl Pts',(1.62431631611976,0.0738960377456204,
1.87400707649719));
#17833=CARTESIAN_POINT('Ctrl Pts',(1.58980227845634,0.0690572297370886,
1.90869858745619));
#17834=CARTESIAN_POINT('',(1.5699559447672,0.259766273896473,1.90869858745619));
#17835=CARTESIAN_POINT('Ctrl Pts',(1.58980227845634,0.0690572297370888,
1.90869858745619));
#17836=CARTESIAN_POINT('Ctrl Pts',(1.58741971380287,0.100162081469027,1.90972905962805));
#17837=CARTESIAN_POINT('Ctrl Pts',(1.58467291856134,0.131250509699795,1.91020759537532));
#17838=CARTESIAN_POINT('Ctrl Pts',(1.58148476202963,0.162313364909724,1.91020766105751));
#17839=CARTESIAN_POINT('Ctrl Pts',(1.57814413491694,0.194861771890306,1.91020772988089));
#17840=CARTESIAN_POINT('Ctrl Pts',(1.57432303476077,0.227345240254558,1.9096825319157));
#17841=CARTESIAN_POINT('Ctrl Pts',(1.5699559447672,0.259766273896474,1.90869858745619));
#17842=CARTESIAN_POINT('',(1.81394816223928,0.428377445609997,1.63615580822897));
#17843=CARTESIAN_POINT('Ctrl Pts',(1.5699559447672,0.259766273896473,1.90869858745619));
#17844=CARTESIAN_POINT('Ctrl Pts',(1.61720542751669,0.262319849600217,1.86166605258539));
#17845=CARTESIAN_POINT('Ctrl Pts',(1.65273856486316,0.277648859150948,1.82419649030262));
#17846=CARTESIAN_POINT('Ctrl Pts',(1.72174825233291,0.325349196380191,1.74786428230698));
#17847=CARTESIAN_POINT('Ctrl Pts',(1.76741714129725,0.365195041941967,1.69596272616121));
#17848=CARTESIAN_POINT('Ctrl Pts',(1.81394816223928,0.428377445609997,1.63615580822897));
#17849=CARTESIAN_POINT('',(1.78098192700405,0.549562141057365,1.63615580822897));
#17850=CARTESIAN_POINT('Origin',(0.,0.,1.63615580822897));
#17851=CARTESIAN_POINT('',(1.49065195897357,0.556953250077769,1.90869858745619));
#17852=CARTESIAN_POINT('Ctrl Pts',(1.78098192700405,0.549562141057366,1.63615580822897));
#17853=CARTESIAN_POINT('Ctrl Pts',(1.73615378094971,0.563182934028546,1.67497485013986));
#17854=CARTESIAN_POINT('Ctrl Pts',(1.69503929836622,0.572158425678773,1.71107791524199));
#17855=CARTESIAN_POINT('Ctrl Pts',(1.63585275285416,0.579760041152422,1.76447740749316));
#17856=CARTESIAN_POINT('Ctrl Pts',(1.6034805809482,0.582920512008171,1.79387050689023));
#17857=CARTESIAN_POINT('Ctrl Pts',(1.54876844626462,0.577874201600796,1.84694613619294));
#17858=CARTESIAN_POINT('Ctrl Pts',(1.52198148549077,0.572220654148339,1.87400707649618));
#17859=CARTESIAN_POINT('Ctrl Pts',(1.49065195897357,0.556953250077769,1.90869858745619));
#17860=CARTESIAN_POINT('',(1.41284463836769,0.732195474855992,1.90869858745619));
#17861=CARTESIAN_POINT('Ctrl Pts',(1.49065195897357,0.55695325007777,1.90869858745619));
#17862=CARTESIAN_POINT('Ctrl Pts',(1.47877407754171,0.585799469037693,1.90972905962805));
#17863=CARTESIAN_POINT('Ctrl Pts',(1.46655486737662,0.614517514878226,1.91020759537532));
#17864=CARTESIAN_POINT('Ctrl Pts',(1.45392380017848,0.643074851191361,1.91020766105751));
#17865=CARTESIAN_POINT('Ctrl Pts',(1.44068866409761,0.672997915195586,1.91020772988089));
#17866=CARTESIAN_POINT('Ctrl Pts',(1.42701663813387,0.702710744569819,1.9096825319157));
#17867=CARTESIAN_POINT('Ctrl Pts',(1.41284463836769,0.732195474855992,1.90869858745619));
#17868=CARTESIAN_POINT('',(1.59279130921887,0.967951970128402,1.63615580822897));
#17869=CARTESIAN_POINT('Ctrl Pts',(1.41284463836769,0.732195474855992,1.90869858745619));
#17870=CARTESIAN_POINT('Ctrl Pts',(1.45699246854266,0.749224962815207,1.86166605258181));
#17871=CARTESIAN_POINT('Ctrl Pts',(1.48604956590136,0.774784060542144,1.82419649029901));
#17872=CARTESIAN_POINT('Ctrl Pts',(1.53694146401919,0.841474943302744,1.74786428229814));
#17873=CARTESIAN_POINT('Ctrl Pts',(1.56806211502394,0.89348305717702,1.69596272615399));
#17874=CARTESIAN_POINT('Ctrl Pts',(1.59279130921887,0.967951970128403,1.63615580822897));
#17875=CARTESIAN_POINT('',(1.5239904260293,1.07301833748062,1.63615580822897));
#17876=CARTESIAN_POINT('Origin',(0.,0.,1.63615580822897));
#17877=CARTESIAN_POINT('',(1.24558623976356,0.990330805779365,1.90869858745619));
#17878=CARTESIAN_POINT('Ctrl Pts',(1.5239904260293,1.07301833748062,1.63615580822897));
#17879=CARTESIAN_POINT('Ctrl Pts',(1.4771472691066,1.07211982243586,1.67497485013931));
#17880=CARTESIAN_POINT('Ctrl Pts',(1.43527149307835,1.06795094842359,1.71107791524167));
#17881=CARTESIAN_POINT('Ctrl Pts',(1.37663271492478,1.05689086595236,1.764477407494));
#17882=CARTESIAN_POINT('Ctrl Pts',(1.34486831068293,1.04989310109054,1.79387050689058));
#17883=CARTESIAN_POINT('Ctrl Pts',(1.29439337414837,1.02818679527943,1.84694613619127));
#17884=CARTESIAN_POINT('Ctrl Pts',(1.27066450279333,1.01453232602804,1.87400707649488));
#17885=CARTESIAN_POINT('Ctrl Pts',(1.24558623976356,0.990330805779365,1.90869858745619));
#17886=CARTESIAN_POINT('',(1.11743425489732,1.13295228123076,1.90869858745619));
#17887=CARTESIAN_POINT('Ctrl Pts',(1.24558623976356,0.990330805779365,1.90869858745619));
#17888=CARTESIAN_POINT('Ctrl Pts',(1.22537573134592,1.01409472307208,1.90972905962805));
#17889=CARTESIAN_POINT('Ctrl Pts',(1.20488020768446,1.03763126410514,1.91020759537532));
#17890=CARTESIAN_POINT('Ctrl Pts',(1.18404264668309,1.06088769047244,1.91020766105751));
#17891=CARTESIAN_POINT('Ctrl Pts',(1.16220854896825,1.08525633350931,1.91020772988089));
#17892=CARTESIAN_POINT('Ctrl Pts',(1.14002391035688,1.10929002513291,1.90968253191571));
#17893=CARTESIAN_POINT('Ctrl Pts',(1.11743425489733,1.13295228123076,1.90869858745619));
#17894=CARTESIAN_POINT('',(1.21572094522251,1.4127766116927,1.63615580822897));
#17895=CARTESIAN_POINT('Ctrl Pts',(1.11743425489733,1.13295228123076,1.90869858745619));
#17896=CARTESIAN_POINT('Ctrl Pts',(1.15415893527859,1.16279071651074,1.8616660525844));
#17897=CARTESIAN_POINT('Ctrl Pts',(1.17389568150877,1.19607799984457,1.82419649030161));
#17898=CARTESIAN_POINT('Ctrl Pts',(1.20168813669685,1.2752312598641,1.74786428230248));
#17899=CARTESIAN_POINT('Ctrl Pts',(1.21521424359528,1.33431072550103,1.69596272615734));
#17900=CARTESIAN_POINT('Ctrl Pts',(1.21572094522251,1.4127766116927,1.63615580822897));
#17901=CARTESIAN_POINT('',(1.11782012388912,1.4914400228729,1.63615580822897));
#17902=CARTESIAN_POINT('Origin',(0.,0.,1.63615580822897));
#17903=CARTESIAN_POINT('',(0.878593860895847,1.32676788217082,1.90869858745619));
#17904=CARTESIAN_POINT('Ctrl Pts',(1.11782012388912,1.4914400228729,1.63615580822897));
#17905=CARTESIAN_POINT('Ctrl Pts',(1.073547290672,1.47611015272516,1.67497485013972));
#17906=CARTESIAN_POINT('Ctrl Pts',(1.03500931392244,1.45920499148459,1.71107791524236));
#17907=CARTESIAN_POINT('Ctrl Pts',(0.982658275295369,1.4305658490011,1.76447740749399));
#17908=CARTESIAN_POINT('Ctrl Pts',(0.954610959919495,1.41409483840251,1.79387050689106));
#17909=CARTESIAN_POINT('Ctrl Pts',(0.913314059996841,1.3778533016347,1.8469461361951));
#17910=CARTESIAN_POINT('Ctrl Pts',(0.894966025319547,1.35753450517017,1.87400707649826));
#17911=CARTESIAN_POINT('Ctrl Pts',(0.878593860895847,1.32676788217082,1.90869858745619));
#17912=CARTESIAN_POINT('',(0.712641620935351,1.42280782457595,1.90869858745619));
#17913=CARTESIAN_POINT('Ctrl Pts',(0.878593860895847,1.32676788217082,1.90869858745619));
#17914=CARTESIAN_POINT('Ctrl Pts',(0.852029070871252,1.34312331999875,1.90972905962805));
#17915=CARTESIAN_POINT('Ctrl Pts',(0.825263478370114,1.35917443559928,1.91020759537532));
#17916=CARTESIAN_POINT('Ctrl Pts',(0.798259149220138,1.37485345097089,1.91020766105751));
#17917=CARTESIAN_POINT('Ctrl Pts',(0.769963363482762,1.39128230047366,1.91020772988089));
#17918=CARTESIAN_POINT('Ctrl Pts',(0.741437699220509,1.40728426915793,1.9096825319157));
#17919=CARTESIAN_POINT('Ctrl Pts',(0.71264162093535,1.42280782457595,1.90869858745619));
#17920=CARTESIAN_POINT('',(0.719647344681868,1.71930883511106,1.63615580822897));
#17921=CARTESIAN_POINT('Ctrl Pts',(0.712641620935351,1.42280782457595,1.90869858745619));
#17922=CARTESIAN_POINT('Ctrl Pts',(0.73834828393456,1.46253441323709,1.86166605258291));
#17923=CARTESIAN_POINT('Ctrl Pts',(0.746832708799669,1.50029149096089,1.82419649029994));
#17924=CARTESIAN_POINT('Ctrl Pts',(0.748805201904025,1.58415905565637,1.74786428230132));
#17925=CARTESIAN_POINT('Ctrl Pts',(0.743412735108989,1.64452676332897,1.69596272615633));
#17926=CARTESIAN_POINT('Ctrl Pts',(0.719647344681868,1.71930883511106,1.63615580822897));
#17927=CARTESIAN_POINT('',(0.602229799711921,1.76386916735271,1.63615580822897));
#17928=CARTESIAN_POINT('Origin',(0.,0.,1.63615580822897));
#17929=CARTESIAN_POINT('',(0.425598593400272,1.53333167412,1.90869858745619));
#17930=CARTESIAN_POINT('Ctrl Pts',(0.602229799711921,1.76386916735271,1.63615580822897));
#17931=CARTESIAN_POINT('Ctrl Pts',(0.564861023582366,1.73560853660092,1.67497485014054));
#17932=CARTESIAN_POINT('Ctrl Pts',(0.533433211786253,1.70762188309983,1.71107791524284));
#17933=CARTESIAN_POINT('Ctrl Pts',(0.492494397099151,1.66420707941326,1.76447740749151));
#17934=CARTESIAN_POINT('Ctrl Pts',(0.47090963723466,1.63987512035499,1.79387050688967));
#17935=CARTESIAN_POINT('Ctrl Pts',(0.442833202224378,1.592645926761,1.84694613619294));
#17936=CARTESIAN_POINT('Ctrl Pts',(0.431662037695335,1.56765174845163,1.87400707649615));
#17937=CARTESIAN_POINT('Ctrl Pts',(0.425598593400271,1.53333167412,1.90869858745619));
#17938=CARTESIAN_POINT('',(0.238090659850088,1.57338902476662,1.90869858745619));
#17939=CARTESIAN_POINT('Ctrl Pts',(0.425598593400271,1.53333167412,1.90869858745619));
#17940=CARTESIAN_POINT('Ctrl Pts',(0.3952798685041,1.5406776482735,1.90972905962805));
#17941=CARTESIAN_POINT('Ctrl Pts',(0.364864209844155,1.54767214341183,1.91020759537532));
#17942=CARTESIAN_POINT('Ctrl Pts',(0.334336484432989,1.55423897652106,1.91020766105751));
#17943=CARTESIAN_POINT('Ctrl Pts',(0.302348799329389,1.56111986223385,1.91020772988089));
#17944=CARTESIAN_POINT('Ctrl Pts',(0.270274400184237,1.56752372379171,1.90968253191571));
#17945=CARTESIAN_POINT('Ctrl Pts',(0.238090659850088,1.57338902476662,1.90869858745619));
#17946=CARTESIAN_POINT('',(0.153129647965883,1.85754313061971,1.63615580822897));
#17947=CARTESIAN_POINT('Ctrl Pts',(0.238090659850088,1.57338902476662,1.90869858745619));
#17948=CARTESIAN_POINT('Ctrl Pts',(0.250262958182808,1.61911505151823,1.86166605258308));
#17949=CARTESIAN_POINT('Ctrl Pts',(0.246664547063409,1.65764599779437,1.82419649030024));
#17950=CARTESIAN_POINT('Ctrl Pts',(0.226553376414497,1.72488162994349,1.76034062848052));
#17951=CARTESIAN_POINT('Ctrl Pts',(0.206497613055206,1.78308197878789,1.7059806272514));
#17952=CARTESIAN_POINT('Ctrl Pts',(0.153129647965883,1.85754313061971,1.63615580822897));
#17953=CARTESIAN_POINT('',(0.0276890267571704,1.86363850813291,1.63615580822897));
#17954=CARTESIAN_POINT('Origin',(0.,0.,1.63615580822897));
#17955=CARTESIAN_POINT('',(-0.0690572297370879,1.58980227845634,1.90869858745619));
#17956=CARTESIAN_POINT('Ctrl Pts',(0.0276890267571701,1.86363850813291,
1.63615580822897));
#17957=CARTESIAN_POINT('Ctrl Pts',(0.000882223887733506,1.82521346421949,
1.67497485013983));
#17958=CARTESIAN_POINT('Ctrl Pts',(-0.0203590497665907,1.78888484709677,
1.71107791524233));
#17959=CARTESIAN_POINT('Ctrl Pts',(-0.045878264098098,1.73494412567795,
1.76447740749215));
#17960=CARTESIAN_POINT('Ctrl Pts',(-0.0588876017641423,1.70513299984437,
1.79387050688967));
#17961=CARTESIAN_POINT('Ctrl Pts',(-0.0709952547835986,1.65153927195887,
1.84694613619187));
#17962=CARTESIAN_POINT('Ctrl Pts',(-0.0738960377459196,1.62431631612179,
1.87400707649515));
#17963=CARTESIAN_POINT('Ctrl Pts',(-0.0690572297370876,1.58980227845634,
1.90869858745619));
#17964=CARTESIAN_POINT('',(-0.259766273896473,1.5699559447672,1.90869858745619));
#17965=CARTESIAN_POINT('Ctrl Pts',(-0.0690572297370876,1.58980227845634,
1.90869858745619));
#17966=CARTESIAN_POINT('Ctrl Pts',(-0.100162081469031,1.58741971380287,
1.90972905962805));
#17967=CARTESIAN_POINT('Ctrl Pts',(-0.131250509699804,1.58467291856134,
1.91020759537532));
#17968=CARTESIAN_POINT('Ctrl Pts',(-0.162313364909724,1.58148476202963,
1.91020766105751));
#17969=CARTESIAN_POINT('Ctrl Pts',(-0.194861771890307,1.57814413491694,
1.91020772988089));
#17970=CARTESIAN_POINT('Ctrl Pts',(-0.22734524025456,1.57432303476077,1.9096825319157));
#17971=CARTESIAN_POINT('Ctrl Pts',(-0.259766273896473,1.5699559447672,1.90869858745619));
#17972=CARTESIAN_POINT('',(-0.428377445609996,1.81394816223928,1.63615580822897));
#17973=CARTESIAN_POINT('Ctrl Pts',(-0.259766273896472,1.5699559447672,1.90869858745619));
#17974=CARTESIAN_POINT('Ctrl Pts',(-0.262319849600359,1.61720542751929,
1.8616660525828));
#17975=CARTESIAN_POINT('Ctrl Pts',(-0.277648859152491,1.65273856486546,
1.82419649030008));
#17976=CARTESIAN_POINT('Ctrl Pts',(-0.325349196384362,1.72174825233888,
1.74786428230037));
#17977=CARTESIAN_POINT('Ctrl Pts',(-0.36519504194757,1.76741714130135,1.69596272615592));
#17978=CARTESIAN_POINT('Ctrl Pts',(-0.428377445609996,1.81394816223928,
1.63615580822897));
#17979=CARTESIAN_POINT('',(-0.549562141057365,1.78098192700405,1.63615580822897));
#17980=CARTESIAN_POINT('Origin',(0.,0.,1.63615580822897));
#17981=CARTESIAN_POINT('',(-0.55695325007777,1.49065195897357,1.90869858745619));
#17982=CARTESIAN_POINT('Ctrl Pts',(-0.549562141057366,1.78098192700405,
1.63615580822897));
#17983=CARTESIAN_POINT('Ctrl Pts',(-0.56318293402824,1.73615378095071,1.67497485013899));
#17984=CARTESIAN_POINT('Ctrl Pts',(-0.572158425678774,1.69503929836625,
1.71107791524196));
#17985=CARTESIAN_POINT('Ctrl Pts',(-0.579760041152499,1.63585275285353,
1.76447740749373));
#17986=CARTESIAN_POINT('Ctrl Pts',(-0.582920512008146,1.60348058094794,
1.79387050689049));
#17987=CARTESIAN_POINT('Ctrl Pts',(-0.577874201600643,1.54876844626296,
1.84694613619456));
#17988=CARTESIAN_POINT('Ctrl Pts',(-0.572220654147739,1.52198148548955,
1.87400707649754));
#17989=CARTESIAN_POINT('Ctrl Pts',(-0.55695325007777,1.49065195897357,1.90869858745619));
#17990=CARTESIAN_POINT('',(-0.732195474855993,1.41284463836769,1.90869858745619));
#17991=CARTESIAN_POINT('Ctrl Pts',(-0.55695325007777,1.49065195897357,1.90869858745619));
#17992=CARTESIAN_POINT('Ctrl Pts',(-0.585799469037708,1.47877407754171,
1.90972905962805));
#17993=CARTESIAN_POINT('Ctrl Pts',(-0.614517514878255,1.46655486737661,
1.91020759537532));
#17994=CARTESIAN_POINT('Ctrl Pts',(-0.643074851191362,1.45392380017848,
1.91020766105751));
#17995=CARTESIAN_POINT('Ctrl Pts',(-0.672997915195577,1.44068866409761,
1.91020772988089));
#17996=CARTESIAN_POINT('Ctrl Pts',(-0.702710744569799,1.42701663813388,
1.90968253191571));
#17997=CARTESIAN_POINT('Ctrl Pts',(-0.732195474855993,1.41284463836769,
1.90869858745619));
#17998=CARTESIAN_POINT('',(-0.967951970128403,1.59279130921887,1.63615580822897));
#17999=CARTESIAN_POINT('Ctrl Pts',(-0.732195474855993,1.41284463836769,
1.90869858745619));
#18000=CARTESIAN_POINT('Ctrl Pts',(-0.749224962815114,1.45699246854241,
1.86166605258207));
#18001=CARTESIAN_POINT('Ctrl Pts',(-0.774784060541914,1.48604956590117,
1.82419649029929));
#18002=CARTESIAN_POINT('Ctrl Pts',(-0.841474943298866,1.53694146401625,
1.74786428230256));
#18003=CARTESIAN_POINT('Ctrl Pts',(-0.893483057172211,1.56806211502235,
1.69596272615784));
#18004=CARTESIAN_POINT('Ctrl Pts',(-0.967951970128403,1.59279130921887,
1.63615580822897));
#18005=CARTESIAN_POINT('',(-1.07301833748062,1.5239904260293,1.63615580822897));
#18006=CARTESIAN_POINT('Origin',(0.,0.,1.63615580822897));
#18007=CARTESIAN_POINT('',(-0.990330805779365,1.24558623976355,1.90869858745619));
#18008=CARTESIAN_POINT('Ctrl Pts',(-1.07301833748062,1.5239904260293,1.63615580822897));
#18009=CARTESIAN_POINT('Ctrl Pts',(-1.07211982243592,1.47714726910886,1.67497485013742));
#18010=CARTESIAN_POINT('Ctrl Pts',(-1.06795094842396,1.43527149308025,1.71107791523994));
#18011=CARTESIAN_POINT('Ctrl Pts',(-1.05689086595159,1.37663271492071,1.7644774074977));
#18012=CARTESIAN_POINT('Ctrl Pts',(-1.04989310109001,1.34486831068169,1.79387050689188));
#18013=CARTESIAN_POINT('Ctrl Pts',(-1.02818679527844,1.29439337414607,1.8469461361937));
#18014=CARTESIAN_POINT('Ctrl Pts',(-1.01453232602662,1.27066450279187,1.87400707649691));
#18015=CARTESIAN_POINT('Ctrl Pts',(-0.990330805779365,1.24558623976356,
1.90869858745619));
#18016=CARTESIAN_POINT('',(-1.13295228123076,1.11743425489732,1.90869858745619));
#18017=CARTESIAN_POINT('Ctrl Pts',(-0.990330805779366,1.24558623976356,
1.90869858745619));
#18018=CARTESIAN_POINT('Ctrl Pts',(-1.01409472307207,1.22537573134593,1.90972905962805));
#18019=CARTESIAN_POINT('Ctrl Pts',(-1.03763126410513,1.20488020768446,1.91020759537532));
#18020=CARTESIAN_POINT('Ctrl Pts',(-1.06088769047244,1.18404264668309,1.91020766105751));
#18021=CARTESIAN_POINT('Ctrl Pts',(-1.08525633350932,1.16220854896824,1.91020772988089));
#18022=CARTESIAN_POINT('Ctrl Pts',(-1.10929002513292,1.14002391035687,1.9096825319157));
#18023=CARTESIAN_POINT('Ctrl Pts',(-1.13295228123076,1.11743425489732,1.90869858745619));
#18024=CARTESIAN_POINT('',(-1.4127766116927,1.21572094522251,1.63615580822897));
#18025=CARTESIAN_POINT('Ctrl Pts',(-1.13295228123076,1.11743425489733,1.90869858745619));
#18026=CARTESIAN_POINT('Ctrl Pts',(-1.16279071651051,1.15415893527831,1.86166605258477));
#18027=CARTESIAN_POINT('Ctrl Pts',(-1.19607799984402,1.17389568150863,1.82419649030211));
#18028=CARTESIAN_POINT('Ctrl Pts',(-1.27523125986877,1.20168813669844,1.74786428229801));
#18029=CARTESIAN_POINT('Ctrl Pts',(-1.33431072550602,1.21521424359531,1.69596272615354));
#18030=CARTESIAN_POINT('Ctrl Pts',(-1.4127766116927,1.21572094522251,1.63615580822897));
#18031=CARTESIAN_POINT('',(-1.4914400228729,1.11782012388913,1.63615580822897));
#18032=CARTESIAN_POINT('Origin',(0.,0.,1.63615580822897));
#18033=CARTESIAN_POINT('',(-1.32676788217082,0.878593860895847,1.90869858745619));
#18034=CARTESIAN_POINT('Ctrl Pts',(-1.4914400228729,1.11782012388913,1.63615580822897));
#18035=CARTESIAN_POINT('Ctrl Pts',(-1.4761101527255,1.07354729067302,1.67497485013884));
#18036=CARTESIAN_POINT('Ctrl Pts',(-1.45920499148537,1.03500931392384,1.71107791524092));
#18037=CARTESIAN_POINT('Ctrl Pts',(-1.43056584900109,0.982658275295367,
1.764477407494));
#18038=CARTESIAN_POINT('Ctrl Pts',(-1.41409483840328,0.954610959920349,
1.79387050688994));
#18039=CARTESIAN_POINT('Ctrl Pts',(-1.37785330163753,0.913314060000089,
1.84694613619094));
#18040=CARTESIAN_POINT('Ctrl Pts',(-1.35753450517376,0.894966025321443,
1.87400707649422));
#18041=CARTESIAN_POINT('Ctrl Pts',(-1.32676788217082,0.878593860895847,
1.90869858745619));
#18042=CARTESIAN_POINT('',(-1.42280782457595,0.712641620935351,1.90869858745619));
#18043=CARTESIAN_POINT('Ctrl Pts',(-1.32676788217082,0.878593860895847,
1.90869858745619));
#18044=CARTESIAN_POINT('Ctrl Pts',(-1.34312331999875,0.852029070871253,
1.90972905962805));
#18045=CARTESIAN_POINT('Ctrl Pts',(-1.35917443559928,0.825263478370115,
1.91020759537532));
#18046=CARTESIAN_POINT('Ctrl Pts',(-1.37485345097089,0.798259149220139,
1.91020766105751));
#18047=CARTESIAN_POINT('Ctrl Pts',(-1.39128230047365,0.769963363482771,
1.91020772988089));
#18048=CARTESIAN_POINT('Ctrl Pts',(-1.40728426915792,0.741437699220528,
1.90968253191571));
#18049=CARTESIAN_POINT('Ctrl Pts',(-1.42280782457595,0.712641620935352,
1.90869858745619));
#18050=CARTESIAN_POINT('',(-1.71930883511106,0.719647344681869,1.63615580822897));
#18051=CARTESIAN_POINT('Ctrl Pts',(-1.42280782457595,0.712641620935352,
1.90869858745619));
#18052=CARTESIAN_POINT('Ctrl Pts',(-1.46253441323564,0.738348283933626,
1.86166605258463));
#18053=CARTESIAN_POINT('Ctrl Pts',(-1.50029149095907,0.746832708799589,
1.82419649030161));
#18054=CARTESIAN_POINT('Ctrl Pts',(-1.58415905564638,0.748805201903826,
1.7478642823104));
#18055=CARTESIAN_POINT('Ctrl Pts',(-1.64452676331943,0.743412735112008,
1.69596272616397));
#18056=CARTESIAN_POINT('Ctrl Pts',(-1.71930883511106,0.719647344681869,
1.63615580822897));
#18057=CARTESIAN_POINT('',(-1.76386916735271,0.602229799711921,1.63615580822897));
#18058=CARTESIAN_POINT('Origin',(0.,0.,1.63615580822897));
#18059=CARTESIAN_POINT('',(-1.53333167412,0.425598593400271,1.90869858745619));
#18060=CARTESIAN_POINT('Ctrl Pts',(-1.76386916735271,0.602229799711921,
1.63615580822897));
#18061=CARTESIAN_POINT('Ctrl Pts',(-1.73560853660219,0.56486102358402,1.67497485013881));
#18062=CARTESIAN_POINT('Ctrl Pts',(-1.70762188310117,0.533433211787508,
1.71107791524119));
#18063=CARTESIAN_POINT('Ctrl Pts',(-1.66420707941108,0.492494397097101,
1.76447740749419));
#18064=CARTESIAN_POINT('Ctrl Pts',(-1.63987512035448,0.470909637234355,
1.79387050689024));
#18065=CARTESIAN_POINT('Ctrl Pts',(-1.59264592676207,0.442833202225016,
1.84694613619173));
#18066=CARTESIAN_POINT('Ctrl Pts',(-1.56765174845278,0.431662037695519,
1.874007076495));
#18067=CARTESIAN_POINT('Ctrl Pts',(-1.53333167412,0.425598593400271,1.90869858745619));
#18068=CARTESIAN_POINT('',(-1.57338902476662,0.238090659850088,1.90869858745619));
#18069=CARTESIAN_POINT('Ctrl Pts',(-1.53333167412,0.425598593400272,1.90869858745619));
#18070=CARTESIAN_POINT('Ctrl Pts',(-1.54067764827351,0.395279868504089,
1.90972905962805));
#18071=CARTESIAN_POINT('Ctrl Pts',(-1.54767214341184,0.364864209844131,
1.91020759537532));
#18072=CARTESIAN_POINT('Ctrl Pts',(-1.55423897652106,0.334336484432989,
1.91020766105751));
#18073=CARTESIAN_POINT('Ctrl Pts',(-1.56111986223385,0.302348799329394,
1.91020772988089));
#18074=CARTESIAN_POINT('Ctrl Pts',(-1.5675237237917,0.270274400184246,1.90968253191571));
#18075=CARTESIAN_POINT('Ctrl Pts',(-1.57338902476662,0.238090659850088,
1.90869858745619));
#18076=CARTESIAN_POINT('',(-1.85754313061971,0.153129647965883,1.63615580822897));
#18077=CARTESIAN_POINT('Ctrl Pts',(-1.57338902476662,0.238090659850089,
1.90869858745619));
#18078=CARTESIAN_POINT('Ctrl Pts',(-1.61911505151772,0.250262958182671,
1.86166605258361));
#18079=CARTESIAN_POINT('Ctrl Pts',(-1.6576459977938,0.246664547063569,1.82419649030078));
#18080=CARTESIAN_POINT('Ctrl Pts',(-1.72488162993957,0.226553376415675,
1.76034062848425));
#18081=CARTESIAN_POINT('Ctrl Pts',(-1.78308197878557,0.20649761305687,1.70598062725359));
#18082=CARTESIAN_POINT('Ctrl Pts',(-1.85754313061971,0.153129647965884,
1.63615580822897));
#18083=CARTESIAN_POINT('',(-1.86363850813291,0.0276890267571705,1.63615580822897));
#18084=CARTESIAN_POINT('Origin',(0.,0.,1.63615580822897));
#18085=CARTESIAN_POINT('Ctrl Pts',(-1.86363850813291,0.0276890267571706,
1.63615580822897));
#18086=CARTESIAN_POINT('Ctrl Pts',(-1.84930856933126,0.0176919049463911,
1.65063268159767));
#18087=CARTESIAN_POINT('Ctrl Pts',(-1.83526820787236,0.00847200864278421,
1.66473179212764));
#18088=CARTESIAN_POINT('Ctrl Pts',(-1.82153560215913,1.34132982498869E-12,
1.67846439784087));
#18089=CARTESIAN_POINT('Origin',(1.,0.,2.1));
#18090=CARTESIAN_POINT('',(-0.0502392594122347,0.998737211088938,2.10000000017302));
#18091=CARTESIAN_POINT('',(0.998737211088938,-0.0502392594122345,2.10000000017302));
#18092=CARTESIAN_POINT('Origin',(0.,0.,2.1));
#18093=CARTESIAN_POINT('',(0.0502392594122347,0.998737211088938,2.10000000017302));
#18094=CARTESIAN_POINT('Ctrl Pts',(-0.0501579420662037,0.998754980171774,
2.09996629646059));
#18095=CARTESIAN_POINT('Ctrl Pts',(-0.0455541516249309,0.998081971740583,
2.09994285225375));
#18096=CARTESIAN_POINT('Ctrl Pts',(-0.0409493960495382,0.997497248478843,
2.09992115702739));
#18097=CARTESIAN_POINT('Ctrl Pts',(-0.0363408599228962,0.997001962981805,
2.0999069394429));
#18098=CARTESIAN_POINT('Ctrl Pts',(-0.0344254769968775,0.996796114235378,
2.09990103038244));
#18099=CARTESIAN_POINT('Ctrl Pts',(-0.0325094393882293,0.996605701141417,
2.09989644467646));
#18100=CARTESIAN_POINT('Ctrl Pts',(-0.030591027199469,0.996431064903213,
2.0998929904383));
#18101=CARTESIAN_POINT('Ctrl Pts',(-0.0241570348712139,0.995845367927649,
2.09988140557563));
#18102=CARTESIAN_POINT('Ctrl Pts',(-0.0177195435991528,0.995439341015549,
2.09988208911745));
#18103=CARTESIAN_POINT('Ctrl Pts',(-0.0112042061332443,0.99522006377236,
2.09989207709953));
#18104=CARTESIAN_POINT('Ctrl Pts',(-0.0091395956891891,0.995150578179511,
2.09989524213775));
#18105=CARTESIAN_POINT('Ctrl Pts',(-0.00706875291999245,0.995099879623312,
2.09989939288935));
#18106=CARTESIAN_POINT('Ctrl Pts',(-0.00498909077113959,0.995068038205673,
2.09990458544879));
#18107=CARTESIAN_POINT('Ctrl Pts',(-0.00372411379059672,0.995048670319229,
2.09990774387919));
#18108=CARTESIAN_POINT('Ctrl Pts',(-0.00245612535390708,0.995036282497343,
2.09991128863539));
#18109=CARTESIAN_POINT('Ctrl Pts',(-0.00118453247084987,0.995030876493846,
2.09991524595687));
#18110=CARTESIAN_POINT('Ctrl Pts',(-4.37845315938809E-5,0.995026026759759,
2.09991879607608));
#18111=CARTESIAN_POINT('Ctrl Pts',(0.00109970303547405,0.995026788370882,
2.09992271042795));
#18112=CARTESIAN_POINT('Ctrl Pts',(0.00223928716687367,0.995033203141033,
2.09992682811702));
#18113=CARTESIAN_POINT('Ctrl Pts',(0.0036616886009847,0.995041209902455,
2.09993196771721));
#18114=CARTESIAN_POINT('Ctrl Pts',(0.00508052255109117,0.995058026539435,
2.09993740601942));
#18115=CARTESIAN_POINT('Ctrl Pts',(0.00649660255618722,0.99508373088496,
2.09994278957186));
#18116=CARTESIAN_POINT('Ctrl Pts',(0.00927146453168093,0.99513409951579,
2.09995333884513));
#18117=CARTESIAN_POINT('Ctrl Pts',(0.0120342525028786,0.995218575771198,
2.09996364717532));
#18118=CARTESIAN_POINT('Ctrl Pts',(0.0147909036437984,0.995337528356299,
2.0999713663429));
#18119=CARTESIAN_POINT('Ctrl Pts',(0.0158423647792016,0.995382900082279,
2.09997431064172));
#18120=CARTESIAN_POINT('Ctrl Pts',(0.0168924947237524,0.995433267490783,
2.09997688114622));
#18121=CARTESIAN_POINT('Ctrl Pts',(0.0179416114429507,0.995488633595717,
2.09997896362948));
#18122=CARTESIAN_POINT('Ctrl Pts',(0.0227736532195703,0.995743639856846,
2.09998855517054));
#18123=CARTESIAN_POINT('Ctrl Pts',(0.027584328345019,0.996104743818564,
2.09998770209067));
#18124=CARTESIAN_POINT('Ctrl Pts',(0.0323893668042188,0.996568206430001,
2.09998210436156));
#18125=CARTESIAN_POINT('Ctrl Pts',(0.0368950513274315,0.997002795316889,
2.09997685537102));
#18126=CARTESIAN_POINT('Ctrl Pts',(0.0413861399780065,0.997526459114176,
2.09996745668706));
#18127=CARTESIAN_POINT('Ctrl Pts',(0.0458741854723339,0.99813430097851,
2.09995967180744));
#18128=CARTESIAN_POINT('Ctrl Pts',(0.0473368418337277,0.998332396958311,
2.09995713471112));
#18129=CARTESIAN_POINT('Ctrl Pts',(0.0487991635875438,0.99853942952464,
2.09995477525694));
#18130=CARTESIAN_POINT('Ctrl Pts',(0.0502611215119263,0.998755291264538,
2.09995263618594));
#18131=CARTESIAN_POINT('',(0.998737211088938,0.0502392594122345,2.10000000017302));
#18132=CARTESIAN_POINT('Origin',(0.,0.,2.1));
#18133=CARTESIAN_POINT('Ctrl Pts',(0.998741489349531,0.0501276226578845,
2.09998790761528));
#18134=CARTESIAN_POINT('Ctrl Pts',(0.998209106442774,0.0465065804968853,
2.0999823604152));
#18135=CARTESIAN_POINT('Ctrl Pts',(0.997731917482903,0.0428858888083561,
2.09997532142456));
#18136=CARTESIAN_POINT('Ctrl Pts',(0.99731100353809,0.0392650986878338,
2.09996763820277));
#18137=CARTESIAN_POINT('Ctrl Pts',(0.996973673612343,0.0363633158470504,
2.0999614806956));
#18138=CARTESIAN_POINT('Ctrl Pts',(0.996672480569791,0.0334615115052595,
2.09995491761494));
#18139=CARTESIAN_POINT('Ctrl Pts',(0.996408345014525,0.0305539602702526,
2.09994817558028));
#18140=CARTESIAN_POINT('Ctrl Pts',(0.995823734577335,0.0241186857880212,
2.09993325345505));
#18141=CARTESIAN_POINT('Ctrl Pts',(0.995422878237189,0.0176782325627147,
2.09991691990568));
#18142=CARTESIAN_POINT('Ctrl Pts',(0.995209369745946,0.0111608079949593,
2.0999080411453));
#18143=CARTESIAN_POINT('Ctrl Pts',(0.99514171218205,0.00909553618039141,
2.09990522760241));
#18144=CARTESIAN_POINT('Ctrl Pts',(0.995092895768509,0.00702412914613266,
2.09990323613576));
#18145=CARTESIAN_POINT('Ctrl Pts',(0.99506286554661,0.00494410069252508,
2.0999025509242));
#18146=CARTESIAN_POINT('Ctrl Pts',(0.99504459933955,0.00367890090298719,
2.09990213413686));
#18147=CARTESIAN_POINT('Ctrl Pts',(0.995033286585864,0.00241076308799952,
2.09990220272711));
#18148=CARTESIAN_POINT('Ctrl Pts',(0.995028899524127,0.00113911783449072,
2.09990288388685));
#18149=CARTESIAN_POINT('Ctrl Pts',(0.995024963884268,-1.67708640180092E-6,
2.09990349495629));
#18150=CARTESIAN_POINT('Ctrl Pts',(0.995026593989671,-0.00114513314823198,
2.09990463268876));
#18151=CARTESIAN_POINT('Ctrl Pts',(0.995033805529301,-0.00228459200009584,
2.09990622411078));
#18152=CARTESIAN_POINT('Ctrl Pts',(0.995042806799174,-0.00370683706316931,
2.09990821048536));
#18153=CARTESIAN_POINT('Ctrl Pts',(0.995060508292759,-0.00512536873273449,
2.09991087886862));
#18154=CARTESIAN_POINT('Ctrl Pts',(0.99508694937675,-0.00654097371496716,
2.0999140064208));
#18155=CARTESIAN_POINT('Ctrl Pts',(0.995138761674284,-0.00931490486528927,
2.09992013497682));
#18156=CARTESIAN_POINT('Ctrl Pts',(0.995224111395307,-0.0120760964135134,
2.09992800145899));
#18157=CARTESIAN_POINT('Ctrl Pts',(0.995343089287915,-0.0148303143798948,
2.09993619328405));
#18158=CARTESIAN_POINT('Ctrl Pts',(0.995539967164857,-0.0193878382523947,
2.09994974865211));
#18159=CARTESIAN_POINT('Ctrl Pts',(0.995828617967945,-0.0239182715715797,
2.09996404004403));
#18160=CARTESIAN_POINT('Ctrl Pts',(0.996207735735797,-0.0284458173699921,
2.09997472302851));
#18161=CARTESIAN_POINT('Ctrl Pts',(0.99631850279087,-0.0297686330154764,
2.09997784428219));
#18162=CARTESIAN_POINT('Ctrl Pts',(0.996436986832906,-0.0310911807891784,
2.09998067371155));
#18163=CARTESIAN_POINT('Ctrl Pts',(0.996563166797704,-0.0324135784390754,
2.09998318511707));
#18164=CARTESIAN_POINT('Ctrl Pts',(0.997133221361869,-0.0383878931186965,
2.09999453111945));
#18165=CARTESIAN_POINT('Ctrl Pts',(0.997858925779834,-0.0443424598651534,
2.09999902027607));
#18166=CARTESIAN_POINT('Ctrl Pts',(0.998734041876947,-0.0502864563072932,
2.0999972397247));
#18167=CARTESIAN_POINT('Ctrl Pts',(0.999999999998244,-1.87406103457374E-6,
2.60499999999311));
#18168=CARTESIAN_POINT('Ctrl Pts',(1.00000006288704,0.033555619638003,2.60500024661583));
#18169=CARTESIAN_POINT('Ctrl Pts',(0.996432788538549,0.100793877077062,
2.59172126532562));
#18170=CARTESIAN_POINT('Ctrl Pts',(0.987779661769916,0.157562252712982,
2.55296011060328));
#18171=CARTESIAN_POINT('Ctrl Pts',(0.977968286593196,0.211192459212548,
2.49909481560466));
#18172=CARTESIAN_POINT('Ctrl Pts',(0.970281147530057,0.242238373929747,
2.44471009644067));
#18173=CARTESIAN_POINT('Ctrl Pts',(0.967388261055284,0.253317392831602,
2.37452193295668));
#18174=CARTESIAN_POINT('Ctrl Pts',(0.967116369990459,0.254356366300813,
2.34056467313598));
#18175=CARTESIAN_POINT('Ctrl Pts',(0.968060909182331,0.250746912814477,
2.30584393595531));
#18176=CARTESIAN_POINT('Ctrl Pts',(0.971275486994325,0.238235555290696,
2.25382796860057));
#18177=CARTESIAN_POINT('Ctrl Pts',(0.978160761261309,0.209370469448592,
2.20003517000389));
#18178=CARTESIAN_POINT('Ctrl Pts',(0.986928061083623,0.163194558725017,
2.1514224394046));
#18179=CARTESIAN_POINT('Ctrl Pts',(0.994800163464163,0.109016749833536,
2.11560611365411));
#18180=CARTESIAN_POINT('Ctrl Pts',(1.00003726905853,0.0393234864952561,
2.09484257852823));
#18181=CARTESIAN_POINT('Ctrl Pts',(1.00039359739908,-0.0285679116079913,
2.09347899005165));
#18182=CARTESIAN_POINT('Ctrl Pts',(0.995946129986918,-0.098499816085455,
2.11089539860567));
#18183=CARTESIAN_POINT('Ctrl Pts',(0.987595534630939,-0.160108842507484,
2.14787016428115));
#18184=CARTESIAN_POINT('Ctrl Pts',(0.978767296657426,-0.20640426202618,
2.19598850651528));
#18185=CARTESIAN_POINT('Ctrl Pts',(0.97062172581105,-0.241091125419321,
2.25963518301816));
#18186=CARTESIAN_POINT('Ctrl Pts',(0.967038345237899,-0.254607790735269,
2.32400532558939));
#18187=CARTESIAN_POINT('Ctrl Pts',(0.967372392238064,-0.253367892292085,
2.39214155711082));
#18188=CARTESIAN_POINT('Ctrl Pts',(0.971848592631414,-0.236216524025834,
2.45101723423612));
#18189=CARTESIAN_POINT('Ctrl Pts',(0.977999994055034,-0.208938409888944,
2.49656599568729));
#18190=CARTESIAN_POINT('Ctrl Pts',(0.982365078241419,-0.187417224408925,
2.52354132496555));
#18191=CARTESIAN_POINT('Ctrl Pts',(0.986694720178997,-0.163267539196543,
2.54663242388917));
#18192=CARTESIAN_POINT('Ctrl Pts',(0.99244571253526,-0.125541882265517,
2.57418619605903));
#18193=CARTESIAN_POINT('Ctrl Pts',(0.998300344088637,-0.0706101566680352,
2.59849422048893));
#18194=CARTESIAN_POINT('Ctrl Pts',(0.999999955756101,-0.0236095057558304,
2.60499982649452));
#18195=CARTESIAN_POINT('Ctrl Pts',(0.999999999998244,-1.87406103457374E-6,
2.60499999999311));
#18196=CARTESIAN_POINT('Ctrl Pts',(0.983333333331803,-1.72646341714646E-6,
2.58833333332708));
#18197=CARTESIAN_POINT('Ctrl Pts',(0.983325070408895,0.0309254949332375,
2.58831701644367));
#18198=CARTESIAN_POINT('Ctrl Pts',(0.980235431771385,0.0928701985922922,
2.5763334457126));
#18199=CARTESIAN_POINT('Ctrl Pts',(0.97262951086769,0.146010496479255,2.54070549738907));
#18200=CARTESIAN_POINT('Ctrl Pts',(0.963966193226361,0.196619990384259,
2.49071684326285));
#18201=CARTESIAN_POINT('Ctrl Pts',(0.957121635980358,0.226408216243534,
2.43967803502293));
#18202=CARTESIAN_POINT('Ctrl Pts',(0.954530758590317,0.237116103160976,
2.37322988185745));
#18203=CARTESIAN_POINT('Ctrl Pts',(0.954292056495262,0.238108034056394,
2.34106055897148));
#18204=CARTESIAN_POINT('Ctrl Pts',(0.955131698824161,0.234634460337268,
2.30818704053657));
#18205=CARTESIAN_POINT('Ctrl Pts',(0.958005717805603,0.222572733944937,
2.2590085409333));
#18206=CARTESIAN_POINT('Ctrl Pts',(0.964133168526514,0.194921019608955,
2.20849850875947));
#18207=CARTESIAN_POINT('Ctrl Pts',(0.971886775166395,0.151277899039362,
2.16333241887712));
#18208=CARTESIAN_POINT('Ctrl Pts',(0.978798486508062,0.100613721566294,
2.13040797264567));
#18209=CARTESIAN_POINT('Ctrl Pts',(0.983369400970407,0.0361963313628681,
2.11151394416968));
#18210=CARTESIAN_POINT('Ctrl Pts',(0.983676824334791,-0.0262950908417384,
2.11028422573118));
#18211=CARTESIAN_POINT('Ctrl Pts',(0.979801092832465,-0.0908603189323969,
2.12610656815928));
#18212=CARTESIAN_POINT('Ctrl Pts',(0.972473802924845,-0.148358154753562,
2.16004581981554));
#18213=CARTESIAN_POINT('Ctrl Pts',(0.964672149439096,-0.192110727398231,
2.20471275196644));
#18214=CARTESIAN_POINT('Ctrl Pts',(0.957427193110245,-0.225297504050057,
2.26446164543395));
#18215=CARTESIAN_POINT('Ctrl Pts',(0.954222830159563,-0.238355411074918,
2.32536038420973));
#18216=CARTESIAN_POINT('Ctrl Pts',(0.954522079095343,-0.2371523061421,2.3899277120541));
#18217=CARTESIAN_POINT('Ctrl Pts',(0.958517953243843,-0.220614507903057,
2.4455635357429));
#18218=CARTESIAN_POINT('Ctrl Pts',(0.963982071416956,-0.194581079725971,
2.48825477624319));
#18219=CARTESIAN_POINT('Ctrl Pts',(0.967849868185066,-0.174169675975904,
2.51340938027297));
#18220=CARTESIAN_POINT('Ctrl Pts',(0.97167321111088,-0.151401045973518,
2.53482806141593));
#18221=CARTESIAN_POINT('Ctrl Pts',(0.976733295652627,-0.116052309467583,
2.56023494607926));
#18222=CARTESIAN_POINT('Ctrl Pts',(0.981853837292877,-0.0650450913579237,
2.58243716495324));
#18223=CARTESIAN_POINT('Ctrl Pts',(0.983332905880957,-0.0217501188318965,
2.58833203941799));
#18224=CARTESIAN_POINT('Ctrl Pts',(0.983333333331803,-1.72646341714646E-6,
2.58833333332708));
#18225=CARTESIAN_POINT('Ctrl Pts',(0.966666666665363,-1.57886579971917E-6,
2.57166666666104));
#18226=CARTESIAN_POINT('Ctrl Pts',(0.966675031089233,0.0282574067618839,
2.57168340910161));
#18227=CARTESIAN_POINT('Ctrl Pts',(0.964030995123869,0.0849671350523733,
2.56092437077672));
#18228=CARTESIAN_POINT('Ctrl Pts',(0.957496079669552,0.134432741424285,
2.52848314020048));
#18229=CARTESIAN_POINT('Ctrl Pts',(0.949965488618089,0.18202293386404,2.48231761863255));
#18230=CARTESIAN_POINT('Ctrl Pts',(0.943960096058651,0.210589600813346,
2.4346289274524));
#18231=CARTESIAN_POINT('Ctrl Pts',(0.941686431722323,0.220882428486858,
2.3719223211333));
#18232=CARTESIAN_POINT('Ctrl Pts',(0.94146963989202,0.221854615130021,2.34155719007975));
#18233=CARTESIAN_POINT('Ctrl Pts',(0.942215861234142,0.218493014540143,
2.31051805593517));
#18234=CARTESIAN_POINT('Ctrl Pts',(0.944737453851974,0.206900615314252,
2.26419080172698));
#18235=CARTESIAN_POINT('Ctrl Pts',(0.950105713610565,0.180489574889026,
2.21697132240232));
#18236=CARTESIAN_POINT('Ctrl Pts',(0.956837948144641,0.139371349739201,
2.17526823220057));
#18237=CARTESIAN_POINT('Ctrl Pts',(0.962797300252717,0.0922406494407946,
2.14521214199563));
#18238=CARTESIAN_POINT('Ctrl Pts',(0.966692768725039,0.0330593334366949,
2.12821013824094));
#18239=CARTESIAN_POINT('Ctrl Pts',(0.966958180635997,-0.0240006511464648,
2.12709572724774));
#18240=CARTESIAN_POINT('Ctrl Pts',(0.963654605188848,-0.08321040561347,
2.1413234011611));
#18241=CARTESIAN_POINT('Ctrl Pts',(0.957353720921044,-0.136587098613656,
2.17220985324203));
#18242=CARTESIAN_POINT('Ctrl Pts',(0.950573235959199,-0.177820331414012,
2.21345060010943));
#18243=CARTESIAN_POINT('Ctrl Pts',(0.944223169736954,-0.209514123317684,
2.26930212368042));
#18244=CARTESIAN_POINT('Ctrl Pts',(0.941403959395846,-0.222103494504004,
2.32673583609555));
#18245=CARTESIAN_POINT('Ctrl Pts',(0.941667556372663,-0.220946133881027,
2.38772812706794));
#18246=CARTESIAN_POINT('Ctrl Pts',(0.945187704752525,-0.205008502652309,
2.44011245850097));
#18247=CARTESIAN_POINT('Ctrl Pts',(0.94997031235299,-0.180221173921234,
2.47994404421443));
#18248=CARTESIAN_POINT('Ctrl Pts',(0.953336718390379,-0.160920110206714,
2.5032802399603));
#18249=CARTESIAN_POINT('Ctrl Pts',(0.956651963018509,-0.139538170190601,
2.5230099883211));
#18250=CARTESIAN_POINT('Ctrl Pts',(0.961021973375283,-0.10656485199273,
2.54628159282629));
#18251=CARTESIAN_POINT('Ctrl Pts',(0.965409168116845,-0.0594989402485911,
2.56637680898634));
#18252=CARTESIAN_POINT('Ctrl Pts',(0.966667022710479,-0.0198905682807695,
2.57166766119149));
#18253=CARTESIAN_POINT('Ctrl Pts',(0.966666666665363,-1.57886579971917E-6,
2.57166666666104));
#18254=CARTESIAN_POINT('Ctrl Pts',(0.949999999998922,-1.43126818229188E-6,
2.554999999995));
#18255=CARTESIAN_POINT('Ctrl Pts',(0.950000038611092,0.0256272820571184,
2.55500017892945));
#18256=CARTESIAN_POINT('Ctrl Pts',(0.947833638356706,0.077043456567603,
2.5455365511637));
#18257=CARTESIAN_POINT('Ctrl Pts',(0.942345928767326,0.122880985190557,
2.51622852698627));
#18258=CARTESIAN_POINT('Ctrl Pts',(0.935963395251255,0.167450465035751,
2.47393964629074));
#18259=CARTESIAN_POINT('Ctrl Pts',(0.930800584508952,0.194759443127133,
2.42959686603466));
#18260=CARTESIAN_POINT('Ctrl Pts',(0.928828929257356,0.204681138816232,
2.37063027003408));
#18261=CARTESIAN_POINT('Ctrl Pts',(0.928645326396822,0.205606282885602,
2.34205307591525));
#18262=CARTESIAN_POINT('Ctrl Pts',(0.929286650875972,0.202380562062934,
2.31286116051643));
#18263=CARTESIAN_POINT('Ctrl Pts',(0.931467684663253,0.191237793968494,
2.26937137405972));
#18264=CARTESIAN_POINT('Ctrl Pts',(0.93607812087577,0.166040125049389,2.2254346611579));
#18265=CARTESIAN_POINT('Ctrl Pts',(0.941796662227414,0.127454690053546,
2.18717821167308));
#18266=CARTESIAN_POINT('Ctrl Pts',(0.946795623296616,0.0838376211735529,
2.16001400098719));
#18267=CARTESIAN_POINT('Ctrl Pts',(0.950024900636915,0.0299321783043069,
2.14488150388239));
#18268=CARTESIAN_POINT('Ctrl Pts',(0.950241407571709,-0.0217278303802119,
2.14390096292727));
#18269=CARTESIAN_POINT('Ctrl Pts',(0.947509568034395,-0.0755709084604119,
2.15653457071471));
#18270=CARTESIAN_POINT('Ctrl Pts',(0.942231989214949,-0.124836410859733,
2.18438550877642));
#18271=CARTESIAN_POINT('Ctrl Pts',(0.936478088740869,-0.163526796786063,
2.22217484556059));
#18272=CARTESIAN_POINT('Ctrl Pts',(0.931028637036149,-0.19372050194842,
2.27412858609622));
#18273=CARTESIAN_POINT('Ctrl Pts',(0.92858844431751,-0.205851114843653,
2.32809089471589));
#18274=CARTESIAN_POINT('Ctrl Pts',(0.928817243229942,-0.204730547731042,
2.38551428201123));
#18275=CARTESIAN_POINT('Ctrl Pts',(0.931857065364954,-0.189406486529532,
2.43465876000775));
#18276=CARTESIAN_POINT('Ctrl Pts',(0.935952389714912,-0.165863843758261,
2.47163282477033));
#18277=CARTESIAN_POINT('Ctrl Pts',(0.938821508334025,-0.147672561773693,
2.49314829526772));
#18278=CARTESIAN_POINT('Ctrl Pts',(0.941630453950392,-0.127671676967576,
2.51120562584786));
#18279=CARTESIAN_POINT('Ctrl Pts',(0.945309556492649,-0.0970752791947962,
2.53233034284651));
#18280=CARTESIAN_POINT('Ctrl Pts',(0.948962661321086,-0.0539338749384796,
2.55031975345065));
#18281=CARTESIAN_POINT('Ctrl Pts',(0.949999972835335,-0.0180311813568356,
2.55499987411497));
#18282=CARTESIAN_POINT('Ctrl Pts',(0.949999999998922,-1.43126818229188E-6,
2.554999999995));
#18283=CARTESIAN_POINT('',(0.987458837468112,0.157876674357314,2.54999999999916));
#18284=CARTESIAN_POINT('Ctrl Pts',(0.998741489263531,0.0501276243402692,
2.09998790795724));
#18285=CARTESIAN_POINT('Ctrl Pts',(0.997746174412029,0.0695985876399753,
2.10394554683626));
#18286=CARTESIAN_POINT('Ctrl Pts',(0.994363645806935,0.112020975270126,
2.11759217250489));
#18287=CARTESIAN_POINT('Ctrl Pts',(0.986928061083623,0.163194558725017,
2.1514224394046));
#18288=CARTESIAN_POINT('Ctrl Pts',(0.978160761261309,0.209370469448592,
2.20003517000389));
#18289=CARTESIAN_POINT('Ctrl Pts',(0.971275486994325,0.238235555290696,
2.25382796860057));
#18290=CARTESIAN_POINT('Ctrl Pts',(0.968060909182331,0.250746912814477,
2.30584393595531));
#18291=CARTESIAN_POINT('Ctrl Pts',(0.967116369990459,0.254356366300813,
2.34056467313598));
#18292=CARTESIAN_POINT('Ctrl Pts',(0.967388261055284,0.253317392831602,
2.37452193295668));
#18293=CARTESIAN_POINT('Ctrl Pts',(0.970281147530057,0.242238373929747,
2.44471009644067));
#18294=CARTESIAN_POINT('Ctrl Pts',(0.977968286593196,0.211192459212548,
2.49909481560466));
#18295=CARTESIAN_POINT('Ctrl Pts',(0.98494013308223,0.173083472433883,2.53737085347425));
#18296=CARTESIAN_POINT('Ctrl Pts',(0.986199840262143,0.165761961406214,
2.54388428246999));
#18297=CARTESIAN_POINT('Ctrl Pts',(0.987440095705288,0.157976027584706,
2.55002758371622));
#18298=CARTESIAN_POINT('',(0.972500000001548,-1.63052496584468E-6,2.57749999999709));
#18299=CARTESIAN_POINT('Ctrl Pts',(0.987458837468451,0.157876674355192,
2.55));
#18300=CARTESIAN_POINT('Ctrl Pts',(0.985294697406766,0.146794280964263,
2.55388665064189));
#18301=CARTESIAN_POINT('Ctrl Pts',(0.983354421647032,0.135549889588831,
2.55740912752908));
#18302=CARTESIAN_POINT('Ctrl Pts',(0.977055328631449,0.0935709003424381,
2.56892572544489));
#18303=CARTESIAN_POINT('Ctrl Pts',(0.974161715360584,0.0622013742464855,
2.57437596695135));
#18304=CARTESIAN_POINT('Ctrl Pts',(0.972834706545006,0.0246194032981655,
2.57687004873351));
#18305=CARTESIAN_POINT('Ctrl Pts',(0.972691422895011,0.0189840464089377,
2.57713968402705));
#18306=CARTESIAN_POINT('Ctrl Pts',(0.972559701868467,0.0105124985263587,
2.57738760007473));
#18307=CARTESIAN_POINT('Ctrl Pts',(0.972529696233088,0.0076814295447408,
2.5774440907214));
#18308=CARTESIAN_POINT('Ctrl Pts',(0.972504563213093,0.00323267114025078,
2.57749140831944));
#18309=CARTESIAN_POINT('Ctrl Pts',(0.972499996930093,0.00161553516506767,
2.57750000577993));
#18310=CARTESIAN_POINT('Ctrl Pts',(0.972500000001548,-1.63052496584468E-6,
2.57749999999708));
#18311=CARTESIAN_POINT('',(0.949999999998922,-1.43126818229188E-6,2.554999999995));
#18312=CARTESIAN_POINT('Ctrl Pts',(0.972500000001548,-1.63052496584468E-6,
2.57749999999709));
#18313=CARTESIAN_POINT('Ctrl Pts',(0.965000000000673,-1.56410603799375E-6,
2.56999999999639));
#18314=CARTESIAN_POINT('Ctrl Pts',(0.957499999999797,-1.49768711014282E-6,
2.5624999999957));
#18315=CARTESIAN_POINT('Ctrl Pts',(0.949999999998922,-1.43126818229188E-6,
2.554999999995));
#18316=CARTESIAN_POINT('',(0.950017413548361,2.77722566314428E-6,2.14493017758226));
#18317=CARTESIAN_POINT('Ctrl Pts',(0.949999999998922,-1.43126818229188E-6,
2.554999999995));
#18318=CARTESIAN_POINT('Ctrl Pts',(0.950000038611092,0.0256272820571184,
2.55500017892945));
#18319=CARTESIAN_POINT('Ctrl Pts',(0.947833638356706,0.077043456567603,
2.5455365511637));
#18320=CARTESIAN_POINT('Ctrl Pts',(0.942345928767326,0.122880985190557,
2.51622852698627));
#18321=CARTESIAN_POINT('Ctrl Pts',(0.935963395251255,0.167450465035751,
2.47393964629074));
#18322=CARTESIAN_POINT('Ctrl Pts',(0.930800584508952,0.194759443127133,
2.42959686603466));
#18323=CARTESIAN_POINT('Ctrl Pts',(0.928828929257356,0.204681138816232,
2.37063027003408));
#18324=CARTESIAN_POINT('Ctrl Pts',(0.928645326396822,0.205606282885602,
2.34205307591525));
#18325=CARTESIAN_POINT('Ctrl Pts',(0.929286650875972,0.202380562062934,
2.31286116051643));
#18326=CARTESIAN_POINT('Ctrl Pts',(0.931467684663253,0.191237793968494,
2.26937137405972));
#18327=CARTESIAN_POINT('Ctrl Pts',(0.93607812087577,0.166040125049389,2.2254346611579));
#18328=CARTESIAN_POINT('Ctrl Pts',(0.941796662227414,0.127454690053546,
2.18717821167308));
#18329=CARTESIAN_POINT('Ctrl Pts',(0.946795623296616,0.0838376211735529,
2.16001400098719));
#18330=CARTESIAN_POINT('Ctrl Pts',(0.949571221584807,0.0375053185605399,
2.14700745845955));
#18331=CARTESIAN_POINT('Ctrl Pts',(0.950019209030419,0.0100740119424525,
2.1449223021834));
#18332=CARTESIAN_POINT('Ctrl Pts',(0.950017413548361,2.77722566314337E-6,
2.14493017758226));
#18333=CARTESIAN_POINT('Ctrl Pts',(0.950017413548361,2.77722566314337E-6,
2.14493017758226));
#18334=CARTESIAN_POINT('Ctrl Pts',(0.950016105516441,-0.0073342476264757,
2.14493591491227));
#18335=CARTESIAN_POINT('Ctrl Pts',(0.949714588734556,-0.0321111444056223,
2.14633727826451));
#18336=CARTESIAN_POINT('Ctrl Pts',(0.947509568034395,-0.0755709084604119,
2.15653457071471));
#18337=CARTESIAN_POINT('Ctrl Pts',(0.942231989214949,-0.124836410859733,
2.18438550877642));
#18338=CARTESIAN_POINT('Ctrl Pts',(0.936478088740869,-0.163526796786063,
2.22217484556059));
#18339=CARTESIAN_POINT('Ctrl Pts',(0.931028637036149,-0.19372050194842,
2.27412858609622));
#18340=CARTESIAN_POINT('Ctrl Pts',(0.92858844431751,-0.205851114843653,
2.32809089471589));
#18341=CARTESIAN_POINT('Ctrl Pts',(0.928817243229942,-0.204730547731042,
2.38551428201123));
#18342=CARTESIAN_POINT('Ctrl Pts',(0.931857065364954,-0.189406486529532,
2.43465876000775));
#18343=CARTESIAN_POINT('Ctrl Pts',(0.935952389714912,-0.165863843758261,
2.47163282477033));
#18344=CARTESIAN_POINT('Ctrl Pts',(0.938821508334025,-0.147672561773693,
2.49314829526772));
#18345=CARTESIAN_POINT('Ctrl Pts',(0.941630453950392,-0.127671676967576,
2.51120562584786));
#18346=CARTESIAN_POINT('Ctrl Pts',(0.945309556492649,-0.0970752791947962,
2.53233034284651));
#18347=CARTESIAN_POINT('Ctrl Pts',(0.948962661321086,-0.0539338749384796,
2.55031975345065));
#18348=CARTESIAN_POINT('Ctrl Pts',(0.949999972835335,-0.0180311813568356,
2.55499987411497));
#18349=CARTESIAN_POINT('Ctrl Pts',(0.949999999998922,-1.43126818229188E-6,
2.554999999995));
#18350=CARTESIAN_POINT('',(0.987458837468112,-0.157876674357314,2.54999999999916));
#18351=CARTESIAN_POINT('Ctrl Pts',(0.972500000001548,-1.63052496584468E-6,
2.57749999999708));
#18352=CARTESIAN_POINT('Ctrl Pts',(0.972500001100936,-0.00058047386256792,
2.57749999792719));
#18353=CARTESIAN_POINT('Ctrl Pts',(0.972500587629742,-0.00115932100720252,
2.5774988936244));
#18354=CARTESIAN_POINT('Ctrl Pts',(0.972506627935273,-0.00414265020170195,
2.57748752117621));
#18355=CARTESIAN_POINT('Ctrl Pts',(0.972521597304209,-0.00654688441944551,
2.57745933671442));
#18356=CARTESIAN_POINT('Ctrl Pts',(0.972586968658232,-0.0128156465435284,
2.57733627628346));
#18357=CARTESIAN_POINT('Ctrl Pts',(0.972653363288269,-0.016678636176991,
2.57721129835072));
#18358=CARTESIAN_POINT('Ctrl Pts',(0.972929256482295,-0.0281987946478753,
2.57669227394828));
#18359=CARTESIAN_POINT('Ctrl Pts',(0.973215079278776,-0.0358422720486581,
2.57615478699383));
#18360=CARTESIAN_POINT('Ctrl Pts',(0.974562717145952,-0.0623401377173552,
2.57362665221117));
#18361=CARTESIAN_POINT('Ctrl Pts',(0.976141626745025,-0.0810078079633483,
2.57067014303824));
#18362=CARTESIAN_POINT('Ctrl Pts',(0.980686505593143,-0.119336271682647,
2.56227318576719));
#18363=CARTESIAN_POINT('Ctrl Pts',(0.98374047439577,-0.138835225480723,
2.55667793110024));
#18364=CARTESIAN_POINT('Ctrl Pts',(0.987458837468451,-0.157876674355193,
2.55));
#18365=CARTESIAN_POINT('Ctrl Pts',(0.987454582400007,-0.157881308716372,
2.55005328965836));
#18366=CARTESIAN_POINT('Ctrl Pts',(0.987200786017512,-0.159467384180762,
2.5487918471679));
#18367=CARTESIAN_POINT('Ctrl Pts',(0.985506430965119,-0.169895526191808,
2.54029497054242));
#18368=CARTESIAN_POINT('Ctrl Pts',(0.982365078241419,-0.187417224408925,
2.52354132496555));
#18369=CARTESIAN_POINT('Ctrl Pts',(0.977999994055034,-0.208938409888944,
2.49656599568729));
#18370=CARTESIAN_POINT('Ctrl Pts',(0.971848592631414,-0.236216524025834,
2.45101723423612));
#18371=CARTESIAN_POINT('Ctrl Pts',(0.967372392238064,-0.253367892292085,
2.39214155711082));
#18372=CARTESIAN_POINT('Ctrl Pts',(0.967038345237899,-0.254607790735269,
2.32400532558939));
#18373=CARTESIAN_POINT('Ctrl Pts',(0.97062172581105,-0.241091125419321,
2.25963518301816));
#18374=CARTESIAN_POINT('Ctrl Pts',(0.978767296657426,-0.20640426202618,
2.19598850651528));
#18375=CARTESIAN_POINT('Ctrl Pts',(0.987595534630939,-0.160108842507484,
2.14787016428115));
#18376=CARTESIAN_POINT('Ctrl Pts',(0.995084474394307,-0.104856939129847,
2.11471063719305));
#18377=CARTESIAN_POINT('Ctrl Pts',(0.997930949375477,-0.066177461549665,
2.10319104189167));
#18378=CARTESIAN_POINT('Ctrl Pts',(0.998734041791771,-0.0502864579926989,
2.09999724006344));
#18379=CARTESIAN_POINT('Origin',(0.,0.,2.325));
#18380=CARTESIAN_POINT('',(-1.,-1.22464679914735E-16,2.55));
#18381=CARTESIAN_POINT('Origin',(0.,0.,2.55));
#18382=CARTESIAN_POINT('',(-0.157876674357314,0.987458837468112,2.54999999999916));
#18383=CARTESIAN_POINT('Origin',(0.,0.,2.55));
#18384=CARTESIAN_POINT('Ctrl Pts',(-0.0501579437468834,0.998754980083996,
2.09996629680899));
#18385=CARTESIAN_POINT('Ctrl Pts',(-0.0826028085300709,0.997060472227549,
2.10669206239688));
#18386=CARTESIAN_POINT('Ctrl Pts',(-0.13333014615059,0.991871170579173,
2.12768221339602));
#18387=CARTESIAN_POINT('Ctrl Pts',(-0.184987608046235,0.98297944306662,
2.17252130019332));
#18388=CARTESIAN_POINT('Ctrl Pts',(-0.230530876255093,0.973454395083889,
2.2311541204646));
#18389=CARTESIAN_POINT('Ctrl Pts',(-0.255122284839583,0.966868905933786,
2.30756601931672));
#18390=CARTESIAN_POINT('Ctrl Pts',(-0.253875658998481,0.967246420818866,
2.38036927332879));
#18391=CARTESIAN_POINT('Ctrl Pts',(-0.237007380156922,0.971620587810882,
2.45580858562862));
#18392=CARTESIAN_POINT('Ctrl Pts',(-0.204967295321157,0.979117858283225,
2.50518732075992));
#18393=CARTESIAN_POINT('Ctrl Pts',(-0.173082478875929,0.984944804714717,
2.53735038518041));
#18394=CARTESIAN_POINT('Ctrl Pts',(-0.165770169783921,0.986201917446944,
2.54386940226406));
#18395=CARTESIAN_POINT('Ctrl Pts',(-0.157987843541269,0.987440871532657,
2.55001521460453));
#18396=CARTESIAN_POINT('Origin',(0.,0.,2.325));
#18397=CARTESIAN_POINT('',(0.157876674357314,0.987458837468112,2.54999999999916));
#18398=CARTESIAN_POINT('Ctrl Pts',(0.15787361447241,0.987459601094589,2.55002190145526));
#18399=CARTESIAN_POINT('Ctrl Pts',(0.159367603381274,0.987220783300611,
2.54883298459783));
#18400=CARTESIAN_POINT('Ctrl Pts',(0.16716148070395,0.985957317693993,2.54248953138653));
#18401=CARTESIAN_POINT('Ctrl Pts',(0.197782154055467,0.980628932028831,
2.51447081618292));
#18402=CARTESIAN_POINT('Ctrl Pts',(0.240862072091396,0.970821978192215,
2.45070211099161));
#18403=CARTESIAN_POINT('Ctrl Pts',(0.253753920072381,0.967257584978194,
2.38208598978509));
#18404=CARTESIAN_POINT('Ctrl Pts',(0.25377137321269,0.967257227319747,2.31770963275004));
#18405=CARTESIAN_POINT('Ctrl Pts',(0.247407872853293,0.96898626609141,2.28335835196792));
#18406=CARTESIAN_POINT('Ctrl Pts',(0.223542473616943,0.974765351154506,
2.22546113156583));
#18407=CARTESIAN_POINT('Ctrl Pts',(0.202625228604316,0.979486896662666,
2.19281789751093));
#18408=CARTESIAN_POINT('Ctrl Pts',(0.152664347670934,0.988739671565028,
2.14180432402534));
#18409=CARTESIAN_POINT('Ctrl Pts',(0.102949265500905,0.995581814195147,
2.11270476782457));
#18410=CARTESIAN_POINT('Ctrl Pts',(0.0581205001812461,0.998362457461274,
2.10152203482183));
#18411=CARTESIAN_POINT('Ctrl Pts',(0.0502611231985831,0.998755291180234,
2.09995263652274));
#18412=CARTESIAN_POINT('Origin',(0.,0.,2.55));
#18413=CARTESIAN_POINT('Origin',(0.705,0.,2.35));
#18414=CARTESIAN_POINT('',(0.501,-1.25526296912604E-17,2.145));
#18415=CARTESIAN_POINT('',(0.705,-2.51052593825207E-17,2.145));
#18416=CARTESIAN_POINT('',(0.457138928554548,-0.205,2.35));
#18417=CARTESIAN_POINT('Ctrl Pts',(0.457138928554548,-0.205,2.35));
#18418=CARTESIAN_POINT('Ctrl Pts',(0.457138928554548,-0.205,2.32390927987453));
#18419=CARTESIAN_POINT('Ctrl Pts',(0.459609069157102,-0.199722778787908,
2.29632432035936));
#18420=CARTESIAN_POINT('Ctrl Pts',(0.468177727272261,-0.178715671123715,
2.24592797085052));
#18421=CARTESIAN_POINT('Ctrl Pts',(0.474117890962221,-0.162998335554875,
2.22308455526839));
#18422=CARTESIAN_POINT('Ctrl Pts',(0.485018345626291,-0.126935588134045,
2.18702180784756));
#18423=CARTESIAN_POINT('Ctrl Pts',(0.490733376060334,-0.104084611878653,
2.17128923329376));
#18424=CARTESIAN_POINT('Ctrl Pts',(0.498772107838147,-0.0536585253249439,
2.1502704112139));
#18425=CARTESIAN_POINT('Ctrl Pts',(0.501,-0.0260615896504235,2.145));
#18426=CARTESIAN_POINT('Ctrl Pts',(0.501,-6.24500451351651E-17,2.145));
#18427=CARTESIAN_POINT('Ctrl Pts',(0.501,0.,2.145));
#18428=CARTESIAN_POINT('Ctrl Pts',(0.501,0.0260615896504235,2.145));
#18429=CARTESIAN_POINT('Ctrl Pts',(0.498772107838147,0.0536585253249438,
2.1502704112139));
#18430=CARTESIAN_POINT('Ctrl Pts',(0.490733376060334,0.104084611878653,
2.17128923329376));
#18431=CARTESIAN_POINT('Ctrl Pts',(0.485018345626291,0.126935588134045,
2.18702180784756));
#18432=CARTESIAN_POINT('Ctrl Pts',(0.474117890962221,0.162998335554875,
2.22308455526839));
#18433=CARTESIAN_POINT('Ctrl Pts',(0.468177727272261,0.178715671123715,
2.24592797085052));
#18434=CARTESIAN_POINT('Ctrl Pts',(0.459609069157102,0.199722778787908,
2.29632432035936));
#18435=CARTESIAN_POINT('Ctrl Pts',(0.457138928554548,0.205,2.32390927987453));
#18436=CARTESIAN_POINT('Ctrl Pts',(0.457138928554548,0.205,2.37609072012547));
#18437=CARTESIAN_POINT('Ctrl Pts',(0.459609069157102,0.199722778787908,
2.40367567964064));
#18438=CARTESIAN_POINT('Ctrl Pts',(0.468177727272261,0.178715671123715,
2.45407202914948));
#18439=CARTESIAN_POINT('Ctrl Pts',(0.474117890962221,0.162998335554875,
2.47691544473161));
#18440=CARTESIAN_POINT('Ctrl Pts',(0.485018345626291,0.126935588134045,
2.51297819215244));
#18441=CARTESIAN_POINT('Ctrl Pts',(0.490733376060334,0.104084611878653,
2.52871076670624));
#18442=CARTESIAN_POINT('Ctrl Pts',(0.498772107838147,0.0536585253249439,
2.5497295887861));
#18443=CARTESIAN_POINT('Ctrl Pts',(0.501,0.0260615896504235,2.555));
#18444=CARTESIAN_POINT('Ctrl Pts',(0.501,-0.0260615896504234,2.555));
#18445=CARTESIAN_POINT('Ctrl Pts',(0.498772107838147,-0.0536585253249438,
2.5497295887861));
#18446=CARTESIAN_POINT('Ctrl Pts',(0.490733376060334,-0.104084611878653,
2.52871076670624));
#18447=CARTESIAN_POINT('Ctrl Pts',(0.485018345626291,-0.126935588134045,
2.51297819215244));
#18448=CARTESIAN_POINT('Ctrl Pts',(0.474117890962222,-0.162998335554875,
2.47691544473161));
#18449=CARTESIAN_POINT('Ctrl Pts',(0.468177727272261,-0.178715671123715,
2.45407202914948));
#18450=CARTESIAN_POINT('Ctrl Pts',(0.459609069157102,-0.199722778787908,
2.40367567964064));
#18451=CARTESIAN_POINT('Ctrl Pts',(0.457138928554548,-0.205,2.37609072012547));
#18452=CARTESIAN_POINT('Ctrl Pts',(0.457138928554548,-0.205,2.35));
#18453=CARTESIAN_POINT('Ctrl Pts',(1.8740610339731E-6,0.999999999998244,
2.60499999999311));
#18454=CARTESIAN_POINT('Ctrl Pts',(-0.0335556196380034,1.00000006288704,
2.60500024661583));
#18455=CARTESIAN_POINT('Ctrl Pts',(-0.100756673071006,0.996441174833638,
2.59168345968582));
#18456=CARTESIAN_POINT('Ctrl Pts',(-0.157603488695687,0.98777358833807,
2.55296445525625));
#18457=CARTESIAN_POINT('Ctrl Pts',(-0.204967295321157,0.979117858283225,
2.50518732075992));
#18458=CARTESIAN_POINT('Ctrl Pts',(-0.237007380156922,0.971620587810882,
2.45580858562862));
#18459=CARTESIAN_POINT('Ctrl Pts',(-0.253875658998481,0.967246420818866,
2.38036927332879));
#18460=CARTESIAN_POINT('Ctrl Pts',(-0.255122284839583,0.966868905933786,
2.30756601931672));
#18461=CARTESIAN_POINT('Ctrl Pts',(-0.230530876255093,0.973454395083889,
2.2311541204646));
#18462=CARTESIAN_POINT('Ctrl Pts',(-0.184987608046235,0.98297944306662,
2.17252130019332));
#18463=CARTESIAN_POINT('Ctrl Pts',(-0.130000247114384,0.992444341497521,
2.12479183461179));
#18464=CARTESIAN_POINT('Ctrl Pts',(-0.0547900546441262,0.999800917250482,
2.09586490599377));
#18465=CARTESIAN_POINT('Ctrl Pts',(0.00901292386013043,1.00025490450459,
2.09401178448709));
#18466=CARTESIAN_POINT('Ctrl Pts',(0.0460479466138129,0.999088187246804,
2.09861314679373));
#18467=CARTESIAN_POINT('Ctrl Pts',(0.101662133244068,0.995758958476132,
2.11195137517568));
#18468=CARTESIAN_POINT('Ctrl Pts',(0.152664347670934,0.988739671565028,
2.14180432402534));
#18469=CARTESIAN_POINT('Ctrl Pts',(0.202625228604316,0.979486896662666,
2.19281789751093));
#18470=CARTESIAN_POINT('Ctrl Pts',(0.223542473616943,0.974765351154506,
2.22546113156583));
#18471=CARTESIAN_POINT('Ctrl Pts',(0.247407872853293,0.96898626609141,2.28335835196792));
#18472=CARTESIAN_POINT('Ctrl Pts',(0.25377137321269,0.967257227319747,2.31770963275004));
#18473=CARTESIAN_POINT('Ctrl Pts',(0.253753920072381,0.967257584978194,
2.38208598978509));
#18474=CARTESIAN_POINT('Ctrl Pts',(0.240862072091396,0.970821978192215,
2.45070211099161));
#18475=CARTESIAN_POINT('Ctrl Pts',(0.197782154055467,0.980628932028831,
2.51447081618292));
#18476=CARTESIAN_POINT('Ctrl Pts',(0.16267570908935,0.986737898868484,2.54659412947604));
#18477=CARTESIAN_POINT('Ctrl Pts',(0.136234199434897,0.990851168416345,
2.56664374352278));
#18478=CARTESIAN_POINT('Ctrl Pts',(0.0840473157184407,0.997329420352096,
2.59494454511583));
#18479=CARTESIAN_POINT('Ctrl Pts',(0.03365753814838,0.999999936925475,2.60499975264892));
#18480=CARTESIAN_POINT('Ctrl Pts',(1.8740610339731E-6,0.999999999998244,
2.60499999999311));
#18481=CARTESIAN_POINT('Ctrl Pts',(1.72646341657069E-6,0.983333333331803,
2.58833333332708));
#18482=CARTESIAN_POINT('Ctrl Pts',(-0.0309211194933883,0.983327802047045,
2.58831966882739));
#18483=CARTESIAN_POINT('Ctrl Pts',(-0.0928377960476621,0.98023976768212,
2.57629404074584));
#18484=CARTESIAN_POINT('Ctrl Pts',(-0.146048423576797,0.972626976944164,
2.54070953195264));
#18485=CARTESIAN_POINT('Ctrl Pts',(-0.190747496194426,0.964977664234015,
2.49636747507197));
#18486=CARTESIAN_POINT('Ctrl Pts',(-0.221374849129247,0.95831490086092,
2.45011538765543));
#18487=CARTESIAN_POINT('Ctrl Pts',(-0.237650481571607,0.954402200933291,
2.37878285196974));
#18488=CARTESIAN_POINT('Ctrl Pts',(-0.238858199349336,0.954071300725052,
2.30977107620483));
#18489=CARTESIAN_POINT('Ctrl Pts',(-0.215099921034606,0.959955138122488,
2.23759648199501));
#18490=CARTESIAN_POINT('Ctrl Pts',(-0.17183883952112,0.968399947196108,
2.18290355895676));
#18491=CARTESIAN_POINT('Ctrl Pts',(-0.120099054224975,0.976743248230922,
2.13876052168788));
#18492=CARTESIAN_POINT('Ctrl Pts',(-0.0504163434655785,0.983158893045571,
2.11245900795287));
#18493=CARTESIAN_POINT('Ctrl Pts',(0.00827833993718029,0.983561344274991,
2.1107555539468));
#18494=CARTESIAN_POINT('Ctrl Pts',(0.0424518621317906,0.982538668939213,
2.11495120932668));
#18495=CARTESIAN_POINT('Ctrl Pts',(0.0937720299455498,0.979640570051344,
2.12707976132422));
#18496=CARTESIAN_POINT('Ctrl Pts',(0.141360481904814,0.973477223378796,
2.15443787690997));
#18497=CARTESIAN_POINT('Ctrl Pts',(0.188538345234594,0.965310317630362,
2.20179163355866));
#18498=CARTESIAN_POINT('Ctrl Pts',(0.208490757001602,0.961105657569896,
2.23236164151278));
#18499=CARTESIAN_POINT('Ctrl Pts',(0.231400254955185,0.955964354544338,
2.28688145033855));
#18500=CARTESIAN_POINT('Ctrl Pts',(0.237544330067899,0.954413219989739,
2.31941255684048));
#18501=CARTESIAN_POINT('Ctrl Pts',(0.237537755869605,0.954418441564086,
2.38038851320367));
#18502=CARTESIAN_POINT('Ctrl Pts',(0.225032695661137,0.957606932779055,
2.44537253850971));
#18503=CARTESIAN_POINT('Ctrl Pts',(0.183910350012796,0.966318757498156,
2.50501316984723));
#18504=CARTESIAN_POINT('Ctrl Pts',(0.150857782836235,0.971711641804196,
2.53478061849988));
#18505=CARTESIAN_POINT('Ctrl Pts',(0.126062259734711,0.975331110231934,
2.55328561568025));
#18506=CARTESIAN_POINT('Ctrl Pts',(0.0774389729843563,0.981016367853088,
2.57924416260037));
#18507=CARTESIAN_POINT('Ctrl Pts',(0.0310095625324942,0.983324489370319,
2.58831441049439));
#18508=CARTESIAN_POINT('Ctrl Pts',(1.72646341657069E-6,0.983333333331803,
2.58833333332708));
#18509=CARTESIAN_POINT('Ctrl Pts',(1.57886579916828E-6,0.966666666665363,
2.57166666666104));
#18510=CARTESIAN_POINT('Ctrl Pts',(-0.028261782201734,0.966672299451083,
2.57168075671789));
#18511=CARTESIAN_POINT('Ctrl Pts',(-0.0849369725180309,0.964038061600584,
2.56088137505698));
#18512=CARTESIAN_POINT('Ctrl Pts',(-0.134467081311291,0.957489301980934,
2.52849464185));
#18513=CARTESIAN_POINT('Ctrl Pts',(-0.176493077367449,0.950850885491106,
2.48751717131812));
#18514=CARTESIAN_POINT('Ctrl Pts',(-0.205749279945383,0.945011607194673,
2.44443170330968));
#18515=CARTESIAN_POINT('Ctrl Pts',(-0.221405615759076,0.941576404880082,
2.37718285612148));
#18516=CARTESIAN_POINT('Ctrl Pts',(-0.222592256095046,0.941273043800734,
2.31198020634687));
#18517=CARTESIAN_POINT('Ctrl Pts',(-0.19967059846768,0.946452066132863,
2.24404982314633));
#18518=CARTESIAN_POINT('Ctrl Pts',(-0.158679713896286,0.953815819341673,
2.19329233666131));
#18519=CARTESIAN_POINT('Ctrl Pts',(-0.110198993644362,0.961036297799555,
2.15273846356872));
#18520=CARTESIAN_POINT('Ctrl Pts',(-0.046075343884759,0.966525769606431,
2.12903238312702));
#18521=CARTESIAN_POINT('Ctrl Pts',(0.00757919676247354,0.966850980745995,
2.12753983018364));
#18522=CARTESIAN_POINT('Ctrl Pts',(0.0388114474174279,0.965990205488828,
2.13128917659776));
#18523=CARTESIAN_POINT('Ctrl Pts',(0.0859427838572395,0.963505820548163,
2.14224095850635));
#18524=CARTESIAN_POINT('Ctrl Pts',(0.130095057847622,0.958228990545236,
2.16703937038342));
#18525=CARTESIAN_POINT('Ctrl Pts',(0.17448083867517,0.95111834103327,2.21079555546396));
#18526=CARTESIAN_POINT('Ctrl Pts',(0.193473476747956,0.947464227672504,
2.23924962741081));
#18527=CARTESIAN_POINT('Ctrl Pts',(0.215362766008526,0.942940862740997,
2.29040473546289));
#18528=CARTESIAN_POINT('Ctrl Pts',(0.221328116324425,0.941582271034106,
2.32111335094323));
#18529=CARTESIAN_POINT('Ctrl Pts',(0.221307475198179,0.941576462552143,
2.37869131092512));
#18530=CARTESIAN_POINT('Ctrl Pts',(0.209212867982546,0.944395419867102,
2.44004063866257));
#18531=CARTESIAN_POINT('Ctrl Pts',(0.170035598298793,0.952016482602868,
2.49557168347949));
#18532=CARTESIAN_POINT('Ctrl Pts',(0.139037988014577,0.956682144907831,
2.52295666497662));
#18533=CARTESIAN_POINT('Ctrl Pts',(0.115891644338605,0.959813980610051,
2.53993061096407));
#18534=CARTESIAN_POINT('Ctrl Pts',(0.0708540967431303,0.964686661475804,
2.56350215110508));
#18535=CARTESIAN_POINT('Ctrl Pts',(0.0283530954373026,0.96667540882895,
2.57168516269162));
#18536=CARTESIAN_POINT('Ctrl Pts',(1.57886579916828E-6,0.966666666665363,
2.57166666666104));
#18537=CARTESIAN_POINT('Ctrl Pts',(1.43126818176587E-6,0.949999999998922,
2.554999999995));
#18538=CARTESIAN_POINT('Ctrl Pts',(-0.0256272820571188,0.950000038611092,
2.55500017892945));
#18539=CARTESIAN_POINT('Ctrl Pts',(-0.0770180954946874,0.947836654449066,
2.545491956117));
#18540=CARTESIAN_POINT('Ctrl Pts',(-0.122912016192401,0.942342690587028,
2.51623971854639));
#18541=CARTESIAN_POINT('Ctrl Pts',(-0.162273278240718,0.936710691441896,
2.47869732563017));
#18542=CARTESIAN_POINT('Ctrl Pts',(-0.190116748917708,0.931705920244711,
2.43873850533649));
#18543=CARTESIAN_POINT('Ctrl Pts',(-0.205180438332203,0.928732184994508,
2.37559643476243));
#18544=CARTESIAN_POINT('Ctrl Pts',(-0.2063281706048,0.928475438592001,2.31418526323498));
#18545=CARTESIAN_POINT('Ctrl Pts',(-0.184239643247193,0.932952809171462,
2.25049218467674));
#18546=CARTESIAN_POINT('Ctrl Pts',(-0.14553094537117,0.939236323471161,
2.20367459542476));
#18547=CARTESIAN_POINT('Ctrl Pts',(-0.100297800754953,0.945335204532955,
2.16670715064481));
#18548=CARTESIAN_POINT('Ctrl Pts',(-0.0417016327062113,0.94988374540152,
2.14562648508612));
#18549=CARTESIAN_POINT('Ctrl Pts',(0.0068446128395234,0.950157420516395,
2.14428359964335));
#18550=CARTESIAN_POINT('Ctrl Pts',(0.0352153629354055,0.949440687181237,
2.14762723913071));
#18551=CARTESIAN_POINT('Ctrl Pts',(0.0780526805587212,0.947387432123376,
2.15736934465489));
#18552=CARTESIAN_POINT('Ctrl Pts',(0.118791192081503,0.942966542359005,
2.17967292326805));
#18553=CARTESIAN_POINT('Ctrl Pts',(0.160393955305448,0.936941762000965,
2.2197692915117));
#18554=CARTESIAN_POINT('Ctrl Pts',(0.178421760132616,0.933804534087895,
2.24615013735776));
#18555=CARTESIAN_POINT('Ctrl Pts',(0.199355148110418,0.929918951193924,
2.29392783383353));
#18556=CARTESIAN_POINT('Ctrl Pts',(0.205101073179634,0.928738263704097,
2.32281627503367));
#18557=CARTESIAN_POINT('Ctrl Pts',(0.205091310995403,0.928737319138035,
2.3769938343437));
#18558=CARTESIAN_POINT('Ctrl Pts',(0.193383491552286,0.931180374453942,
2.43471106618067));
#18559=CARTESIAN_POINT('Ctrl Pts',(0.156163794256122,0.937706308072193,
2.4861140371438));
#18560=CARTESIAN_POINT('Ctrl Pts',(0.127220061761462,0.941655887843543,
2.51114315400046));
#18561=CARTESIAN_POINT('Ctrl Pts',(0.105719704638418,0.944293922425639,
2.52657248312153));
#18562=CARTESIAN_POINT('Ctrl Pts',(0.0642457540090459,0.948373608976796,
2.54780176858962));
#18563=CARTESIAN_POINT('Ctrl Pts',(0.0257051198214169,0.949999961273794,
2.55499982053709));
#18564=CARTESIAN_POINT('Ctrl Pts',(1.43126818176587E-6,0.949999999998922,
2.554999999995));
#18565=CARTESIAN_POINT('',(1.63052496528509E-6,0.972500000001548,2.57749999999709));
#18566=CARTESIAN_POINT('Ctrl Pts',(-0.157876674355192,0.987458837468451,
2.55));
#18567=CARTESIAN_POINT('Ctrl Pts',(-0.14679428096426,0.985294697406766,
2.55388665064189));
#18568=CARTESIAN_POINT('Ctrl Pts',(-0.135549889588828,0.983354421647031,
2.55740912752908));
#18569=CARTESIAN_POINT('Ctrl Pts',(-0.0935709003424397,0.977055328631449,
2.56892572544489));
#18570=CARTESIAN_POINT('Ctrl Pts',(-0.062201374246487,0.974161715360584,
2.57437596695135));
#18571=CARTESIAN_POINT('Ctrl Pts',(-0.024619403298166,0.972834706545006,
2.57687004873351));
#18572=CARTESIAN_POINT('Ctrl Pts',(-0.0189840464089389,0.972691422895011,
2.57713968402705));
#18573=CARTESIAN_POINT('Ctrl Pts',(-0.0105124985263454,0.972559701868467,
2.57738760007473));
#18574=CARTESIAN_POINT('Ctrl Pts',(-0.00768142954473445,0.972529696233088,
2.5774440907214));
#18575=CARTESIAN_POINT('Ctrl Pts',(-0.0032326711402507,0.972504563213093,
2.57749140831944));
#18576=CARTESIAN_POINT('Ctrl Pts',(-0.0016155351650678,0.972499996930093,
2.57750000577993));
#18577=CARTESIAN_POINT('Ctrl Pts',(1.63052496528509E-6,0.972500000001548,
2.57749999999708));
#18578=CARTESIAN_POINT('',(1.43126818176587E-6,0.949999999998922,2.554999999995));
#18579=CARTESIAN_POINT('Ctrl Pts',(1.63052496528509E-6,0.972500000001548,
2.57749999999709));
#18580=CARTESIAN_POINT('Ctrl Pts',(1.56410603744535E-6,0.965000000000673,
2.56999999999639));
#18581=CARTESIAN_POINT('Ctrl Pts',(1.49768710960561E-6,0.957499999999797,
2.5624999999957));
#18582=CARTESIAN_POINT('Ctrl Pts',(1.43126818176587E-6,0.949999999998922,
2.554999999995));
#18583=CARTESIAN_POINT('',(-3.4869210388678E-5,0.950019014087066,2.14494180214374));
#18584=CARTESIAN_POINT('Ctrl Pts',(1.43126818176587E-6,0.949999999998922,
2.554999999995));
#18585=CARTESIAN_POINT('Ctrl Pts',(-0.0256272820571188,0.950000038611092,
2.55500017892945));
#18586=CARTESIAN_POINT('Ctrl Pts',(-0.0770180954946874,0.947836654449066,
2.545491956117));
#18587=CARTESIAN_POINT('Ctrl Pts',(-0.122912016192401,0.942342690587028,
2.51623971854639));
#18588=CARTESIAN_POINT('Ctrl Pts',(-0.162273278240718,0.936710691441896,
2.47869732563017));
#18589=CARTESIAN_POINT('Ctrl Pts',(-0.190116748917708,0.931705920244711,
2.43873850533649));
#18590=CARTESIAN_POINT('Ctrl Pts',(-0.205180438332203,0.928732184994508,
2.37559643476243));
#18591=CARTESIAN_POINT('Ctrl Pts',(-0.2063281706048,0.928475438592001,2.31418526323498));
#18592=CARTESIAN_POINT('Ctrl Pts',(-0.184239643247193,0.932952809171462,
2.25049218467674));
#18593=CARTESIAN_POINT('Ctrl Pts',(-0.14553094537117,0.939236323471161,
2.20367459542476));
#18594=CARTESIAN_POINT('Ctrl Pts',(-0.100297800754953,0.945335204532955,
2.16670715064481));
#18595=CARTESIAN_POINT('Ctrl Pts',(-0.0465835707283805,0.949504783852479,
2.14738282011878));
#18596=CARTESIAN_POINT('Ctrl Pts',(-0.00936425895417839,0.950027004161095,
2.14491207293051));
#18597=CARTESIAN_POINT('Ctrl Pts',(-3.48692103886768E-5,0.950019014087066,
2.14494180214374));
#18598=CARTESIAN_POINT('Ctrl Pts',(-3.48692103886768E-5,0.950019014087066,
2.14494180214374));
#18599=CARTESIAN_POINT('Ctrl Pts',(0.00462828401910463,0.950015020370377,
2.14495666183772));
#18600=CARTESIAN_POINT('Ctrl Pts',(0.0163025714633961,0.949918483082405,
2.14539826893541));
#18601=CARTESIAN_POINT('Ctrl Pts',(0.0352153629354055,0.949440687181237,
2.14762723913071));
#18602=CARTESIAN_POINT('Ctrl Pts',(0.0780526805587212,0.947387432123376,
2.15736934465489));
#18603=CARTESIAN_POINT('Ctrl Pts',(0.118791192081503,0.942966542359005,
2.17967292326805));
#18604=CARTESIAN_POINT('Ctrl Pts',(0.160393955305448,0.936941762000965,
2.2197692915117));
#18605=CARTESIAN_POINT('Ctrl Pts',(0.178421760132616,0.933804534087895,
2.24615013735776));
#18606=CARTESIAN_POINT('Ctrl Pts',(0.199355148110418,0.929918951193924,
2.29392783383353));
#18607=CARTESIAN_POINT('Ctrl Pts',(0.205101073179634,0.928738263704097,
2.32281627503367));
#18608=CARTESIAN_POINT('Ctrl Pts',(0.205091310995403,0.928737319138035,
2.3769938343437));
#18609=CARTESIAN_POINT('Ctrl Pts',(0.193383491552286,0.931180374453942,
2.43471106618067));
#18610=CARTESIAN_POINT('Ctrl Pts',(0.156163794256122,0.937706308072193,
2.4861140371438));
#18611=CARTESIAN_POINT('Ctrl Pts',(0.127220061761462,0.941655887843543,
2.51114315400046));
#18612=CARTESIAN_POINT('Ctrl Pts',(0.105719704638418,0.944293922425639,
2.52657248312153));
#18613=CARTESIAN_POINT('Ctrl Pts',(0.0642457540090459,0.948373608976796,
2.54780176858962));
#18614=CARTESIAN_POINT('Ctrl Pts',(0.0257051198214169,0.949999961273794,
2.55499982053709));
#18615=CARTESIAN_POINT('Ctrl Pts',(1.43126818176587E-6,0.949999999998922,
2.554999999995));
#18616=CARTESIAN_POINT('Ctrl Pts',(1.63052496528509E-6,0.972500000001548,
2.57749999999708));
#18617=CARTESIAN_POINT('Ctrl Pts',(0.000580473862567526,0.972500001100936,
2.57749999792719));
#18618=CARTESIAN_POINT('Ctrl Pts',(0.00115932100720228,0.972500587629742,
2.5774988936244));
#18619=CARTESIAN_POINT('Ctrl Pts',(0.00414265020169645,0.972506627935274,
2.57748752117621));
#18620=CARTESIAN_POINT('Ctrl Pts',(0.00654688441943462,0.972521597304209,
2.57745933671442));
#18621=CARTESIAN_POINT('Ctrl Pts',(0.0128156465435042,0.972586968658231,
2.57733627628346));
#18622=CARTESIAN_POINT('Ctrl Pts',(0.0166786361769429,0.972653363288268,
2.57721129835072));
#18623=CARTESIAN_POINT('Ctrl Pts',(0.0281987946478794,0.972929256482295,
2.57669227394828));
#18624=CARTESIAN_POINT('Ctrl Pts',(0.0358422720486675,0.973215079278776,
2.57615478699383));
#18625=CARTESIAN_POINT('Ctrl Pts',(0.0623401377173534,0.974562717145952,
2.57362665221117));
#18626=CARTESIAN_POINT('Ctrl Pts',(0.0810078079633459,0.976141626745025,
2.57067014303824));
#18627=CARTESIAN_POINT('Ctrl Pts',(0.119336271682641,0.980686505593142,
2.56227318576719));
#18628=CARTESIAN_POINT('Ctrl Pts',(0.138835225480719,0.983740474395769,
2.55667793110024));
#18629=CARTESIAN_POINT('Ctrl Pts',(0.157876674355193,0.987458837468451,
2.55));
#18630=CARTESIAN_POINT('Origin',(4.31687996699442E-17,0.705,2.35));
#18631=CARTESIAN_POINT('',(-0.205,0.457138928554548,2.35));
#18632=CARTESIAN_POINT('',(-1.45611632917078E-17,0.501,2.145));
#18633=CARTESIAN_POINT('Ctrl Pts',(-0.205,0.457138928554548,2.35));
#18634=CARTESIAN_POINT('Ctrl Pts',(-0.205,0.457138928554548,2.37609072012547));
#18635=CARTESIAN_POINT('Ctrl Pts',(-0.199722778787908,0.459609069157102,
2.40367567964064));
#18636=CARTESIAN_POINT('Ctrl Pts',(-0.178715671123715,0.468177727272261,
2.45407202914948));
#18637=CARTESIAN_POINT('Ctrl Pts',(-0.162998335554875,0.474117890962222,
2.47691544473161));
#18638=CARTESIAN_POINT('Ctrl Pts',(-0.126935588134045,0.485018345626291,
2.51297819215244));
#18639=CARTESIAN_POINT('Ctrl Pts',(-0.104084611878653,0.490733376060334,
2.52871076670624));
#18640=CARTESIAN_POINT('Ctrl Pts',(-0.0536585253249438,0.498772107838147,
2.5497295887861));
#18641=CARTESIAN_POINT('Ctrl Pts',(-0.0260615896504234,0.501,2.555));
#18642=CARTESIAN_POINT('Ctrl Pts',(0.0260615896504235,0.501,2.555));
#18643=CARTESIAN_POINT('Ctrl Pts',(0.0536585253249439,0.498772107838147,
2.5497295887861));
#18644=CARTESIAN_POINT('Ctrl Pts',(0.104084611878653,0.490733376060334,
2.52871076670624));
#18645=CARTESIAN_POINT('Ctrl Pts',(0.126935588134046,0.485018345626291,
2.51297819215244));
#18646=CARTESIAN_POINT('Ctrl Pts',(0.162998335554875,0.474117890962221,
2.47691544473161));
#18647=CARTESIAN_POINT('Ctrl Pts',(0.178715671123715,0.468177727272261,
2.45407202914948));
#18648=CARTESIAN_POINT('Ctrl Pts',(0.199722778787908,0.459609069157102,
2.40367567964064));
#18649=CARTESIAN_POINT('Ctrl Pts',(0.205,0.457138928554548,2.37609072012547));
#18650=CARTESIAN_POINT('Ctrl Pts',(0.205,0.457138928554548,2.32390927987453));
#18651=CARTESIAN_POINT('Ctrl Pts',(0.199722778787908,0.459609069157102,
2.29632432035936));
#18652=CARTESIAN_POINT('Ctrl Pts',(0.178715671123715,0.468177727272261,
2.24592797085052));
#18653=CARTESIAN_POINT('Ctrl Pts',(0.162998335554875,0.474117890962221,
2.22308455526839));
#18654=CARTESIAN_POINT('Ctrl Pts',(0.126935588134045,0.485018345626291,
2.18702180784756));
#18655=CARTESIAN_POINT('Ctrl Pts',(0.104084611878653,0.490733376060334,
2.17128923329376));
#18656=CARTESIAN_POINT('Ctrl Pts',(0.0536585253249439,0.498772107838147,
2.1502704112139));
#18657=CARTESIAN_POINT('Ctrl Pts',(0.0260615896504234,0.501,2.145));
#18658=CARTESIAN_POINT('Ctrl Pts',(-3.46944695195361E-17,0.501,2.145));
#18659=CARTESIAN_POINT('Ctrl Pts',(-3.46944695195361E-17,0.501,2.145));
#18660=CARTESIAN_POINT('Ctrl Pts',(-0.0260615896504235,0.501,2.145));
#18661=CARTESIAN_POINT('Ctrl Pts',(-0.0536585253249439,0.498772107838147,
2.1502704112139));
#18662=CARTESIAN_POINT('Ctrl Pts',(-0.104084611878653,0.490733376060334,
2.17128923329376));
#18663=CARTESIAN_POINT('Ctrl Pts',(-0.126935588134045,0.485018345626291,
2.18702180784756));
#18664=CARTESIAN_POINT('Ctrl Pts',(-0.162998335554875,0.474117890962221,
2.22308455526839));
#18665=CARTESIAN_POINT('Ctrl Pts',(-0.178715671123715,0.468177727272261,
2.24592797085052));
#18666=CARTESIAN_POINT('Ctrl Pts',(-0.199722778787908,0.459609069157102,
2.29632432035936));
#18667=CARTESIAN_POINT('Ctrl Pts',(-0.205,0.457138928554548,2.32390927987453));
#18668=CARTESIAN_POINT('Ctrl Pts',(-0.205,0.457138928554548,2.35));
#18669=CARTESIAN_POINT('',(1.80635402874235E-17,0.705,2.145));
#18670=CARTESIAN_POINT('Origin',(0.,0.,2.575));
#18671=CARTESIAN_POINT('',(-0.95,-1.16341445918999E-16,2.6));
#18672=CARTESIAN_POINT('Origin',(0.,0.,2.6));
#18673=CARTESIAN_POINT('',(-0.975,-1.19403062916867E-16,2.575));
#18674=CARTESIAN_POINT('Ctrl Pts',(1.03743092372925,-0.292083537906633,
1.28318517918604));
#18675=CARTESIAN_POINT('Ctrl Pts',(1.23979244918951,-0.398891247467648,
1.53750926858099));
#18676=CARTESIAN_POINT('Ctrl Pts',(1.33623488367509,-0.594491629104928,
1.74606924121326));
#18677=CARTESIAN_POINT('Ctrl Pts',(1.32675822718598,-0.878884682818471,
1.90886509708283));
#18678=CARTESIAN_POINT('Ctrl Pts',(1.05199356151554,-0.294610685989129,
1.26845681306972));
#18679=CARTESIAN_POINT('Ctrl Pts',(1.25726427409018,-0.402631406009323,
1.51984840181958));
#18680=CARTESIAN_POINT('Ctrl Pts',(1.35531508433345,-0.600652305106672,
1.72608377212012));
#18681=CARTESIAN_POINT('Ctrl Pts',(1.34605472186502,-0.888971417088906,
1.88700775532559));
#18682=CARTESIAN_POINT('Ctrl Pts',(1.07830248703538,-0.30261409250914,1.241120378339));
#18683=CARTESIAN_POINT('Ctrl Pts',(1.28869195855348,-0.413428941810942,
1.48709498232077));
#18684=CARTESIAN_POINT('Ctrl Pts',(1.38909450341186,-0.616606838701699,
1.68880599613843));
#18685=CARTESIAN_POINT('Ctrl Pts',(1.3795008682383,-0.912150767476977,1.84625490381855));
#18686=CARTESIAN_POINT('Ctrl Pts',(1.13234954650476,-0.339741650892321,
1.18057861631985));
#18687=CARTESIAN_POINT('Ctrl Pts',(1.35241043892922,-0.460769919763724,
1.41443334405943));
#18688=CARTESIAN_POINT('Ctrl Pts',(1.45460182159639,-0.677140712937715,
1.60624291768871));
#18689=CARTESIAN_POINT('Ctrl Pts',(1.4388862517722,-0.989017806729689,1.7559174048444));
#18690=CARTESIAN_POINT('Ctrl Pts',(1.17040376051196,-0.384106544865054,
1.1340877844534));
#18691=CARTESIAN_POINT('Ctrl Pts',(1.39633768248716,-0.51607374181577,1.35876508657129));
#18692=CARTESIAN_POINT('Ctrl Pts',(1.49702742698244,-0.744159155535334,
1.54303391436826));
#18693=CARTESIAN_POINT('Ctrl Pts',(1.4722721909128,-1.06856709212992,1.68683916414419));
#18694=CARTESIAN_POINT('Ctrl Pts',(1.19569665581665,-0.420763908606184,
1.10166698368801));
#18695=CARTESIAN_POINT('Ctrl Pts',(1.42522258493376,-0.561378116697244,
1.3199705116299));
#18696=CARTESIAN_POINT('Ctrl Pts',(1.52373714690788,-0.79825366200197,1.49898794576061));
#18697=CARTESIAN_POINT('Ctrl Pts',(1.491240341739,-1.13139054452036,1.63871928608014));
#18698=CARTESIAN_POINT('',(1.04067701160391,-0.293809324770207,1.28727233489076));
#18699=CARTESIAN_POINT('',(1.19131159212569,-0.414490807021284,1.10727038327973));
#18700=CARTESIAN_POINT('Ctrl Pts',(1.04067701160391,-0.293809324770207,
1.28727233489076));
#18701=CARTESIAN_POINT('Ctrl Pts',(1.07291073821506,-0.299434836228389,
1.2547227402422));
#18702=CARTESIAN_POINT('Ctrl Pts',(1.09698565606019,-0.312686039747329,
1.22803799031313));
#18703=CARTESIAN_POINT('Ctrl Pts',(1.14435511150659,-0.354129853275147,
1.17079203987136));
#18704=CARTESIAN_POINT('Ctrl Pts',(1.1680017368876,-0.38029714786499,1.14052203161155));
#18705=CARTESIAN_POINT('Ctrl Pts',(1.19131159212569,-0.414490807021284,
1.10727038327973));
#18706=CARTESIAN_POINT('Ctrl Pts',(1.04067701160391,-0.293809324770207,
1.28727233489076));
#18707=CARTESIAN_POINT('Ctrl Pts',(1.12993947443311,-0.341610972564375,
1.39987124007464));
#18708=CARTESIAN_POINT('Ctrl Pts',(1.19835965101752,-0.406884846288962,
1.50346488650363));
#18709=CARTESIAN_POINT('Ctrl Pts',(1.30500348982786,-0.592356746173702,
1.715480776583));
#18710=CARTESIAN_POINT('Ctrl Pts',(1.33194693676576,-0.722011051157661,
1.81902921434248));
#18711=CARTESIAN_POINT('Ctrl Pts',(1.32676788217082,-0.878593860895847,
1.90869858745619));
#18712=CARTESIAN_POINT('Ctrl Pts',(1.19131159212569,-0.414490807021284,
1.10727038327973));
#18713=CARTESIAN_POINT('Ctrl Pts',(1.26101451903381,-0.455811744539446,
1.17697999301248));
#18714=CARTESIAN_POINT('Ctrl Pts',(1.3231563905114,-0.510390409161008,1.24430717677952));
#18715=CARTESIAN_POINT('Ctrl Pts',(1.42696598762934,-0.655828360684346,
1.37795460947454));
#18716=CARTESIAN_POINT('Ctrl Pts',(1.46323512106126,-0.744250824847066,
1.43952296396723));
#18717=CARTESIAN_POINT('Ctrl Pts',(1.49770211069246,-0.926020771798772,
1.54471868724305));
#18718=CARTESIAN_POINT('Ctrl Pts',(1.50135379887057,-1.01770953159263,1.59041399531289));
#18719=CARTESIAN_POINT('Ctrl Pts',(1.4914400228729,-1.11782012388912,1.63615580822897));
#18720=CARTESIAN_POINT('Ctrl Pts',(1.26214138440836,-0.114046207919,1.10192461715937));
#18721=CARTESIAN_POINT('Ctrl Pts',(1.51915795367952,-0.193872070477571,
1.32030517702043));
#18722=CARTESIAN_POINT('Ctrl Pts',(1.67285198321398,-0.39921550360964,1.49938098964775));
#18723=CARTESIAN_POINT('Ctrl Pts',(1.72322347301172,-0.730076507315206,
1.63915205504133));
#18724=CARTESIAN_POINT('Ctrl Pts',(1.23350917110672,-0.131128471412264,
1.12620814253777));
#18725=CARTESIAN_POINT('Ctrl Pts',(1.48384440470435,-0.213229856531407,
1.3493730700966));
#18726=CARTESIAN_POINT('Ctrl Pts',(1.63116936194582,-0.416549152036911,
1.53236753871639));
#18727=CARTESIAN_POINT('Ctrl Pts',(1.67535851585319,-0.74115396361005,1.67519578767207));
#18728=CARTESIAN_POINT('Ctrl Pts',(1.18566161414104,-0.154321672329429,
1.16792358645355));
#18729=CARTESIAN_POINT('Ctrl Pts',(1.42508536822677,-0.239112514228603,
1.39930746388997));
#18730=CARTESIAN_POINT('Ctrl Pts',(1.56242925297242,-0.438352145622168,
1.58908978141842));
#18731=CARTESIAN_POINT('Ctrl Pts',(1.59768412386216,-0.752201465653598,
1.73717464481022));
#18732=CARTESIAN_POINT('Ctrl Pts',(1.11989042845005,-0.172598846101517,
1.2281493040678));
#18733=CARTESIAN_POINT('Ctrl Pts',(1.34476711329974,-0.258281860114562,
1.47154499595952));
#18734=CARTESIAN_POINT('Ctrl Pts',(1.47038505632135,-0.450170312236593,
1.67113613169256));
#18735=CARTESIAN_POINT('Ctrl Pts',(1.49675459841166,-0.748265815679371,
1.82691733765972));
#18736=CARTESIAN_POINT('Ctrl Pts',(1.08406383481182,-0.17018101435307,1.26357751389222));
#18737=CARTESIAN_POINT('Ctrl Pts',(1.30156053800083,-0.253820963688729,
1.51402822523202));
#18738=CARTESIAN_POINT('Ctrl Pts',(1.42264323155934,-0.439852505027485,
1.71951214242024));
#18739=CARTESIAN_POINT('Ctrl Pts',(1.44728013834437,-0.728627336389036,
1.87982452105687));
#18740=CARTESIAN_POINT('Ctrl Pts',(1.06503024353735,-0.165188454635723,
1.28318566992362));
#18741=CARTESIAN_POINT('Ctrl Pts',(1.27879462627691,-0.246892212254839,
1.5375404757467));
#18742=CARTESIAN_POINT('Ctrl Pts',(1.39806529952135,-0.42950771085669,1.74612008846831));
#18743=CARTESIAN_POINT('Ctrl Pts',(1.42284226327066,-0.713034950441276,
1.90892450808844));
#18744=CARTESIAN_POINT('',(1.25585067703094,-0.117749801015233,1.10727038327973));
#18745=CARTESIAN_POINT('',(1.06845992077163,-0.166511139289343,1.28727233489076));
#18746=CARTESIAN_POINT('Ctrl Pts',(1.25585067703094,-0.117749801015232,
1.10727038327973));
#18747=CARTESIAN_POINT('Ctrl Pts',(1.23367823136722,-0.131623884554202,
1.12805083925442));
#18748=CARTESIAN_POINT('Ctrl Pts',(1.20873355917046,-0.144946380875744,
1.15131250789248));
#18749=CARTESIAN_POINT('Ctrl Pts',(1.16557150946412,-0.161532774289013,
1.19194777349469));
#18750=CARTESIAN_POINT('Ctrl Pts',(1.14529581701501,-0.168037493511604,
1.21108489279932));
#18751=CARTESIAN_POINT('Ctrl Pts',(1.11004996015815,-0.172484956391328,
1.24526606650747));
#18752=CARTESIAN_POINT('Ctrl Pts',(1.09154853530975,-0.172587502434263,
1.26352342884154));
#18753=CARTESIAN_POINT('Ctrl Pts',(1.06845992077163,-0.166511139289343,
1.28727233489076));
#18754=CARTESIAN_POINT('Ctrl Pts',(1.71930883511106,-0.719647344681869,
1.63615580822897));
#18755=CARTESIAN_POINT('Ctrl Pts',(1.70798257074607,-0.634377380847188,
1.59808263051822));
#18756=CARTESIAN_POINT('Ctrl Pts',(1.68649822169668,-0.55237815462213,1.55687869031203));
#18757=CARTESIAN_POINT('Ctrl Pts',(1.61179111914083,-0.383878819109612,
1.4528510278119));
#18758=CARTESIAN_POINT('Ctrl Pts',(1.55475212125011,-0.306551362590219,
1.3904370872311));
#18759=CARTESIAN_POINT('Ctrl Pts',(1.41508721860523,-0.186091644383525,
1.25222975809873));
#18760=CARTESIAN_POINT('Ctrl Pts',(1.33721040532788,-0.145146699351923,
1.18062438818012));
#18761=CARTESIAN_POINT('Ctrl Pts',(1.25585067703094,-0.117749801015232,
1.10727038327973));
#18762=CARTESIAN_POINT('Ctrl Pts',(1.06845992077163,-0.166511139289343,
1.28727233489076));
#18763=CARTESIAN_POINT('Ctrl Pts',(1.16282366323453,-0.203229920731113,
1.39987124007464));
#18764=CARTESIAN_POINT('Ctrl Pts',(1.23859785430383,-0.259800859583567,
1.50346488650363));
#18765=CARTESIAN_POINT('Ctrl Pts',(1.36677481743678,-0.431100013478375,
1.715480776583));
#18766=CARTESIAN_POINT('Ctrl Pts',(1.40911659430225,-0.556572568507924,
1.81902921434248));
#18767=CARTESIAN_POINT('Ctrl Pts',(1.42280782457595,-0.712641620935351,
1.90869858745619));
#18768=CARTESIAN_POINT('Ctrl Pts',(1.06845992077163,-0.166511139289343,
1.28727233489076));
#18769=CARTESIAN_POINT('Ctrl Pts',(1.28063005644821,-0.24907069698643,1.54044293163017));
#18770=CARTESIAN_POINT('Ctrl Pts',(1.3988219960746,-0.431991468445895,1.74808806329354));
#18771=CARTESIAN_POINT('Ctrl Pts',(1.42303573965083,-0.715273453667736,
1.91020772988088));
#18772=CARTESIAN_POINT('Ctrl Pts',(1.05919895104906,-0.208943867782964,
1.28727233489076));
#18773=CARTESIAN_POINT('Ctrl Pts',(1.26754579908091,-0.299809769973181,
1.54044293163017));
#18774=CARTESIAN_POINT('Ctrl Pts',(1.37811826912839,-0.487026359393917,
1.74808806329354));
#18775=CARTESIAN_POINT('Ctrl Pts',(1.39091636119152,-0.770593636045173,
1.91020772988088));
#18776=CARTESIAN_POINT('Ctrl Pts',(1.04993798132648,-0.251376596276586,
1.28727233489076));
#18777=CARTESIAN_POINT('Ctrl Pts',(1.25446154171361,-0.350548842959932,
1.54044293163017));
#18778=CARTESIAN_POINT('Ctrl Pts',(1.35741454218218,-0.54206125034194,1.74808806329354));
#18779=CARTESIAN_POINT('Ctrl Pts',(1.35879698273221,-0.825913818422611,
1.91020772988088));
#18780=CARTESIAN_POINT('Ctrl Pts',(1.04067701160391,-0.293809324770207,
1.28727233489076));
#18781=CARTESIAN_POINT('Ctrl Pts',(1.24137728434631,-0.401287915946682,
1.54044293163017));
#18782=CARTESIAN_POINT('Ctrl Pts',(1.33671081523597,-0.597096141289963,
1.74808806329354));
#18783=CARTESIAN_POINT('Ctrl Pts',(1.3266776042729,-0.881234000800048,1.91020772988088));
#18784=CARTESIAN_POINT('Ctrl Pts',(1.06845992077163,-0.166511139289343,
1.28727233489076));
#18785=CARTESIAN_POINT('Ctrl Pts',(1.06442058969234,-0.187915337510243,
1.28796759655004));
#18786=CARTESIAN_POINT('Ctrl Pts',(1.06007279171241,-0.209261745030532,
1.2883190755065));
#18787=CARTESIAN_POINT('Ctrl Pts',(1.05542181279351,-0.230552888394581,
1.288319084765));
#18788=CARTESIAN_POINT('Ctrl Pts',(1.05079951139633,-0.251712752465176,
1.28831909396641));
#18789=CARTESIAN_POINT('Ctrl Pts',(1.0458824320276,-0.272796801398346,1.28797193184368));
#18790=CARTESIAN_POINT('Ctrl Pts',(1.04067701160391,-0.293809324770207,
1.28727233489076));
#18791=CARTESIAN_POINT('Origin',(0.,0.,1.37171309575435));
#18792=CARTESIAN_POINT('',(1.26108935601086,-0.0260686553993152,1.10727038327973));
#18793=CARTESIAN_POINT('Origin',(0.,0.,1.10727038327973));
#18794=CARTESIAN_POINT('Ctrl Pts',(1.26108935601086,-0.0260686553993151,
1.10727038327973));
#18795=CARTESIAN_POINT('Ctrl Pts',(1.34014965076829,-0.0438278133131022,
1.17697999301248));
#18796=CARTESIAN_POINT('Ctrl Pts',(1.41611581747018,-0.0765323136032893,
1.24430717677952));
#18797=CARTESIAN_POINT('Ctrl Pts',(1.55978740991095,-0.182773095427518,
1.37795460947453));
#18798=CARTESIAN_POINT('Ctrl Pts',(1.62160544971255,-0.255660077554628,
1.43952296396723));
#18799=CARTESIAN_POINT('Ctrl Pts',(1.71055550747305,-0.417882684528603,
1.54471868724299));
#18800=CARTESIAN_POINT('Ctrl Pts',(1.74236185427981,-0.503955443296344,
1.59041399531284));
#18801=CARTESIAN_POINT('Ctrl Pts',(1.76386916735271,-0.602229799711921,
1.63615580822897));
#18802=CARTESIAN_POINT('Origin',(0.,0.,1.37171309575435));
#18803=CARTESIAN_POINT('',(1.15799828028598,-0.500065917147839,1.10727038327973));
#18804=CARTESIAN_POINT('Ctrl Pts',(1.4127766116927,-1.21572094522251,1.63615580822897));
#18805=CARTESIAN_POINT('Ctrl Pts',(1.42835456209775,-1.13112438230172,1.59808263051822));
#18806=CARTESIAN_POINT('Ctrl Pts',(1.4332608863651,-1.04649945489987,1.55687869031203));
#18807=CARTESIAN_POINT('Ctrl Pts',(1.41427936788009,-0.863161299579018,
1.4528510278119));
#18808=CARTESIAN_POINT('Ctrl Pts',(1.38392755544946,-0.77199249847737,1.3904370872311));
#18809=CARTESIAN_POINT('Ctrl Pts',(1.2883224397548,-0.614269670090824,1.25222975809873));
#18810=CARTESIAN_POINT('Ctrl Pts',(1.22690987286759,-0.551263454538704,
1.18062438818012));
#18811=CARTESIAN_POINT('Ctrl Pts',(1.15799828028598,-0.500065917147839,
1.10727038327973));
#18812=CARTESIAN_POINT('Origin',(0.,0.,1.10727038327973));
#18813=CARTESIAN_POINT('Ctrl Pts',(0.896396663228496,-0.598371737951084,
1.28318517918604));
#18814=CARTESIAN_POINT('Ctrl Pts',(1.05584851328029,-0.762485056494508,
1.537509268581));
#18815=CARTESIAN_POINT('Ctrl Pts',(1.08712687701302,-0.9783144252754,1.74606924121326));
#18816=CARTESIAN_POINT('Ctrl Pts',(0.99023175442669,-1.24585984429376,1.90886509708284));
#18817=CARTESIAN_POINT('Ctrl Pts',(0.909465623084801,-0.605275301161475,
1.26845681306972));
#18818=CARTESIAN_POINT('Ctrl Pts',(1.0713094336526,-0.771441249464594,1.51984840181958));
#18819=CARTESIAN_POINT('Ctrl Pts',(1.1033694726,-0.990069682591163,1.72608377212012));
#18820=CARTESIAN_POINT('Ctrl Pts',(1.00546683912554,-1.26141584343748,1.88700775532559));
#18821=CARTESIAN_POINT('Ctrl Pts',(0.932013737380385,-0.621016981690702,
1.24112031232197));
#18822=CARTESIAN_POINT('Ctrl Pts',(1.09786234356421,-0.791422088358105,
1.48709491630374));
#18823=CARTESIAN_POINT('Ctrl Pts',(1.13056538342229,-1.01568188386468,1.68880590632088));
#18824=CARTESIAN_POINT('Ctrl Pts',(1.03011319759961,-1.29379626687142,1.846254814001));
#18825=CARTESIAN_POINT('Ctrl Pts',(0.971942506168048,-0.673028944353636,
1.180578495595));
#18826=CARTESIAN_POINT('Ctrl Pts',(1.14383306000902,-0.856136223676185,
1.41443322333459));
#18827=CARTESIAN_POINT('Ctrl Pts',(1.17416051125987,-1.09349602729722,1.60624275382305));
#18828=CARTESIAN_POINT('Ctrl Pts',(1.06283879403329,-1.38525239147931,1.75591724097875));
#18829=CARTESIAN_POINT('Ctrl Pts',(0.994424673117317,-0.726981684724075,
1.13408778445339));
#18830=CARTESIAN_POINT('Ctrl Pts',(1.16852049530615,-0.922307368817382,
1.35876508657128));
#18831=CARTESIAN_POINT('Ctrl Pts',(1.19379986392408,-1.17034433001556,1.54303391436826));
#18832=CARTESIAN_POINT('Ctrl Pts',(1.07000866982979,-1.47122482340642,1.68683916414419));
#18833=CARTESIAN_POINT('Ctrl Pts',(1.00715189764781,-0.769660843866376,
1.101666983688));
#18834=CARTESIAN_POINT('Ctrl Pts',(1.18199184824263,-0.974320315501954,
1.31997051162989));
#18835=CARTESIAN_POINT('Ctrl Pts',(1.20248619530708,-1.23004502025839,1.4989879457606));
#18836=CARTESIAN_POINT('Ctrl Pts',(1.06863493884117,-1.53683495813569,1.63871928608013));
#18837=CARTESIAN_POINT('',(0.89895057878464,-0.601016155111926,1.28727233489076));
#18838=CARTESIAN_POINT('',(1.00491994924733,-0.762339710524743,1.10727038327973));
#18839=CARTESIAN_POINT('Ctrl Pts',(0.89895057878464,-0.601016155111926,
1.28727233489076));
#18840=CARTESIAN_POINT('Ctrl Pts',(0.927868295879504,-0.616327103756327,
1.25472274024279));
#18841=CARTESIAN_POINT('Ctrl Pts',(0.946670056291831,-0.636369305963266,
1.22803799031441));
#18842=CARTESIAN_POINT('Ctrl Pts',(0.978914242877883,-0.690422681629505,
1.17079203986898));
#18843=CARTESIAN_POINT('Ctrl Pts',(0.993317381309374,-0.722616466766505,
1.14052203160877));
#18844=CARTESIAN_POINT('Ctrl Pts',(1.00491994924733,-0.762339710524744,
1.10727038327973));
#18845=CARTESIAN_POINT('Ctrl Pts',(0.89895057878464,-0.601016155111926,
1.28727233489076));
#18846=CARTESIAN_POINT('Ctrl Pts',(0.969072704191387,-0.674061841710201,
1.39987124007464));
#18847=CARTESIAN_POINT('Ctrl Pts',(1.01397342270847,-0.757283981982513,
1.50346488650363));
#18848=CARTESIAN_POINT('Ctrl Pts',(1.05808377148838,-0.966632999495317,
1.715480776583));
#18849=CARTESIAN_POINT('Ctrl Pts',(1.04364312863621,-1.09826755410688,1.81902921434248));
#18850=CARTESIAN_POINT('Ctrl Pts',(0.990330805779365,-1.24558623976355,
1.90869858745619));
#18851=CARTESIAN_POINT('Ctrl Pts',(1.00491994924733,-0.762339710524743,
1.10727038327973));
#18852=CARTESIAN_POINT('Ctrl Pts',(1.05844250017153,-0.823177646383102,
1.17697999301248));
#18853=CARTESIAN_POINT('Ctrl Pts',(1.10067719707671,-0.894287935370966,
1.24430717677952));
#18854=CARTESIAN_POINT('Ctrl Pts',(1.1544631922219,-1.06468657657251,1.37795460947453));
#18855=CARTESIAN_POINT('Ctrl Pts',(1.16163314380192,-1.15998911590305,1.43952296396722));
#18856=CARTESIAN_POINT('Ctrl Pts',(1.13824319621308,-1.3435134939588,1.54471868724288));
#18857=CARTESIAN_POINT('Ctrl Pts',(1.113382773081,-1.43184312013692,1.59041399531273));
#18858=CARTESIAN_POINT('Ctrl Pts',(1.07301833748062,-1.52399042602929,1.63615580822897));
#18859=CARTESIAN_POINT('Ctrl Pts',(1.16512557173636,-0.498487526286222,
1.10192461715937));
#18860=CARTESIAN_POINT('Ctrl Pts',(1.38489530661629,-0.653828920782168,
1.32030517702043));
#18861=CARTESIAN_POINT('Ctrl Pts',(1.46761240439959,-0.89661619800095,1.49938098964775));
#18862=CARTESIAN_POINT('Ctrl Pts',(1.41327686508625,-1.22684935794257,1.63915205504132));
#18863=CARTESIAN_POINT('Ctrl Pts',(1.13261600897807,-0.505885883797788,
1.12620814253776));
#18864=CARTESIAN_POINT('Ctrl Pts',(1.34532824088583,-0.661326782584696,
1.3493730700966));
#18865=CARTESIAN_POINT('Ctrl Pts',(1.4226134838877,-0.90022083894692,1.53236753871639));
#18866=CARTESIAN_POINT('Ctrl Pts',(1.36433146342889,-1.22259355973874,1.67519578767206));
#18867=CARTESIAN_POINT('Ctrl Pts',(1.07994282031223,-0.513157335393556,
1.16792434557146));
#18868=CARTESIAN_POINT('Ctrl Pts',(1.28144653067711,-0.667784226973456,
1.39930822300789));
#18869=CARTESIAN_POINT('Ctrl Pts',(1.35050022373304,-0.899713500733374,
1.58909081893483));
#18870=CARTESIAN_POINT('Ctrl Pts',(1.28704482486114,-1.20909629592349,1.73717568232663));
#18871=CARTESIAN_POINT('Ctrl Pts',(1.01174252544333,-0.5102156806996,1.22815018770195));
#18872=CARTESIAN_POINT('Ctrl Pts',(1.19913545447318,-0.661195786769768,
1.47154587959366));
#18873=CARTESIAN_POINT('Ctrl Pts',(1.25930861084253,-0.882510125799204,
1.6711373385863));
#18874=CARTESIAN_POINT('Ctrl Pts',(1.19227095916867,-1.17416443346653,1.82691854455345));
#18875=CARTESIAN_POINT('Ctrl Pts',(0.978417148622633,-0.496845910594336,
1.26357751389222));
#18876=CARTESIAN_POINT('Ctrl Pts',(1.15942263970987,-0.643602406938538,
1.51402822523202));
#18877=CARTESIAN_POINT('Ctrl Pts',(1.21709221666582,-0.857945526599466,
1.71951214242024));
#18878=CARTESIAN_POINT('Ctrl Pts',(1.15128697696661,-1.14019993459331,1.87982452105687));
#18879=CARTESIAN_POINT('Ctrl Pts',(0.961857913410637,-0.486216000974361,
1.28318566992362));
#18880=CARTESIAN_POINT('Ctrl Pts',(1.13991207295831,-0.629977719122415,
1.5375404757467));
#18881=CARTESIAN_POINT('Ctrl Pts',(1.19691393144611,-0.840512044007265,
1.74612008846831));
#18882=CARTESIAN_POINT('Ctrl Pts',(1.13286348887405,-1.11781897562891,1.90892450808844));
#18883=CARTESIAN_POINT('',(0.964710998256926,-0.488533777383804,1.28727233489076));
#18884=CARTESIAN_POINT('Ctrl Pts',(1.15799828028598,-0.500065917147839,
1.10727038327973));
#18885=CARTESIAN_POINT('Ctrl Pts',(1.13262370376014,-0.506409292188322,
1.12805083925462));
#18886=CARTESIAN_POINT('Ctrl Pts',(1.10478303294976,-0.51137141150027,1.15131250789266));
#18887=CARTESIAN_POINT('Ctrl Pts',(1.0586080068788,-0.513808202166539,1.19194777349574));
#18888=CARTESIAN_POINT('Ctrl Pts',(1.03731460866957,-0.513729024230128,
1.21108489280018));
#18889=CARTESIAN_POINT('Ctrl Pts',(1.00241946522287,-0.507067244033001,
1.24526606650725));
#18890=CARTESIAN_POINT('Ctrl Pts',(0.984791876090065,-0.501447516417141,
1.2635234288413));
#18891=CARTESIAN_POINT('Ctrl Pts',(0.964710998256925,-0.488533777383804,
1.28727233489076));
#18892=CARTESIAN_POINT('Ctrl Pts',(0.964710998256926,-0.488533777383804,
1.28727233489076));
#18893=CARTESIAN_POINT('Ctrl Pts',(1.04310952295002,-0.552615413818275,
1.39987124007464));
#18894=CARTESIAN_POINT('Ctrl Pts',(1.09769367964031,-0.629833086622262,
1.50346488650363));
#18895=CARTESIAN_POINT('Ctrl Pts',(1.16666286599128,-0.832357123065218,
1.715480776583));
#18896=CARTESIAN_POINT('Ctrl Pts',(1.16815913695893,-0.964772942765737,
1.81902921434248));
#18897=CARTESIAN_POINT('Ctrl Pts',(1.13295228123076,-1.11743425489732,1.90869858745619));
#18898=CARTESIAN_POINT('Ctrl Pts',(0.964710998256925,-0.488533777383804,
1.28727233489076));
#18899=CARTESIAN_POINT('Ctrl Pts',(1.14098448197888,-0.632616760336964,
1.54044293163017));
#18900=CARTESIAN_POINT('Ctrl Pts',(1.19686606932897,-0.843108069941918,
1.74808806329354));
#18901=CARTESIAN_POINT('Ctrl Pts',(1.13235576030722,-1.12000770619867,1.91020772988088));
#18902=CARTESIAN_POINT('Ctrl Pts',(0.94279085843283,-0.526027903293178,
1.28727233489076));
#18903=CARTESIAN_POINT('Ctrl Pts',(1.11286137791709,-0.676829228446517,
1.54044293163017));
#18904=CARTESIAN_POINT('Ctrl Pts',(1.16016893831867,-0.889051558128351,
1.74808806329354));
#18905=CARTESIAN_POINT('Ctrl Pts',(1.08471353963759,-1.16269489233868,1.91020772988088));
#18906=CARTESIAN_POINT('Ctrl Pts',(0.920870718608735,-0.563522029202552,
1.28727233489076));
#18907=CARTESIAN_POINT('Ctrl Pts',(1.0847382738553,-0.72104169655607,1.54044293163017));
#18908=CARTESIAN_POINT('Ctrl Pts',(1.12347180730837,-0.934995046314783,
1.74808806329354));
#18909=CARTESIAN_POINT('Ctrl Pts',(1.03707131896797,-1.20538207847869,1.91020772988088));
#18910=CARTESIAN_POINT('Ctrl Pts',(0.89895057878464,-0.601016155111926,
1.28727233489076));
#18911=CARTESIAN_POINT('Ctrl Pts',(1.05661516979351,-0.765254164665624,
1.54044293163017));
#18912=CARTESIAN_POINT('Ctrl Pts',(1.08677467629807,-0.980938534501216,
1.74808806329354));
#18913=CARTESIAN_POINT('Ctrl Pts',(0.989429098298345,-1.2480692646187,1.91020772988088));
#18914=CARTESIAN_POINT('Ctrl Pts',(0.964710998256926,-0.488533777383804,
1.28727233489076));
#18915=CARTESIAN_POINT('Ctrl Pts',(0.954255105111264,-0.507642157628455,
1.28796759655004));
#18916=CARTESIAN_POINT('Ctrl Pts',(0.943523700818291,-0.52660025413621,
1.2883190755065));
#18917=CARTESIAN_POINT('Ctrl Pts',(0.932521031881151,-0.545412103245543,
1.288319084765));
#18918=CARTESIAN_POINT('Ctrl Pts',(0.921586204420597,-0.564107960168963,
1.28831909396641));
#18919=CARTESIAN_POINT('Ctrl Pts',(0.910394454615237,-0.582640621209125,
1.28797193184368));
#18920=CARTESIAN_POINT('Ctrl Pts',(0.89895057878464,-0.601016155111926,
1.28727233489076));
#18921=CARTESIAN_POINT('Origin',(0.,0.,1.37171309575435));
#18922=CARTESIAN_POINT('',(0.946792943618188,-0.833432097145897,1.10727038327973));
#18923=CARTESIAN_POINT('Ctrl Pts',(0.967951970128402,-1.59279130921887,
1.63615580822897));
#18924=CARTESIAN_POINT('Ctrl Pts',(1.00890925697988,-1.51714904820957,1.59808263051822));
#18925=CARTESIAN_POINT('Ctrl Pts',(1.03972598936032,-1.43818209714157,1.55687869031203));
#18926=CARTESIAN_POINT('Ctrl Pts',(1.07832809822747,-1.25795153804723,1.4528510278119));
#18927=CARTESIAN_POINT('Ctrl Pts',(1.07763451813115,-1.16186562982554,1.3904370872311));
#18928=CARTESIAN_POINT('Ctrl Pts',(1.03544768423091,-0.982318700621181,
1.25222975809873));
#18929=CARTESIAN_POINT('Ctrl Pts',(0.996510853667277,-0.903418701916906,
1.18062438818012));
#18930=CARTESIAN_POINT('Ctrl Pts',(0.946792943618189,-0.833432097145897,
1.10727038327973));
#18931=CARTESIAN_POINT('Origin',(0.,0.,1.10727038327973));
#18932=CARTESIAN_POINT('Ctrl Pts',(0.667616851768136,-0.846087143183836,
1.28318517918604));
#18933=CARTESIAN_POINT('Ctrl Pts',(0.76855076836202,-1.05144151564591,1.53750926858099));
#18934=CARTESIAN_POINT('Ctrl Pts',(0.731603317170575,-1.26637298918249,
1.74606924121325));
#18935=CARTESIAN_POINT('Ctrl Pts',(0.5567744981938,-1.4908815637936,1.90886509708283));
#18936=CARTESIAN_POINT('Ctrl Pts',(0.677912852846922,-0.856691352655136,
1.26845681306972));
#18937=CARTESIAN_POINT('Ctrl Pts',(0.780487361597373,-1.06473704847503,
1.51984840181957));
#18938=CARTESIAN_POINT('Ctrl Pts',(0.743418369261301,-1.28257214132251,
1.72608377212011));
#18939=CARTESIAN_POINT('Ctrl Pts',(0.566456856673054,-1.5103840982294,1.88700775532558));
#18940=CARTESIAN_POINT('Ctrl Pts',(0.694492950134683,-0.878631748253098,
1.24111924840996));
#18941=CARTESIAN_POINT('Ctrl Pts',(0.799566273875774,-1.0919466731633,1.48709385239173));
#18942=CARTESIAN_POINT('Ctrl Pts',(0.761367941758637,-1.31533666464121,
1.68880445881715));
#18943=CARTESIAN_POINT('Ctrl Pts',(0.579890165126716,-1.54879772833385,
1.84625336649728));
#18944=CARTESIAN_POINT('Ctrl Pts',(0.716394511678361,-0.940438249469774,
1.18057655035131));
#18945=CARTESIAN_POINT('Ctrl Pts',(0.82328888189397,-1.16770072295994,1.4144312780909));
#18946=CARTESIAN_POINT('Ctrl Pts',(0.778782224872496,-1.40281580396029,
1.60624011348192));
#18947=CARTESIAN_POINT('Ctrl Pts',(0.582751305549686,-1.64589229282023,
1.75591460063762));
#18948=CARTESIAN_POINT('Ctrl Pts',(0.721104370153831,-0.998694792103054,
1.1340877844534));
#18949=CARTESIAN_POINT('Ctrl Pts',(0.826320380483539,-1.23825912446582,
1.35876508657128));
#18950=CARTESIAN_POINT('Ctrl Pts',(0.7737148524921,-1.48196804720541,1.54303391436826));
#18951=CARTESIAN_POINT('Ctrl Pts',(0.56300524495508,-1.72986881834178,1.68683916414418));
#18952=CARTESIAN_POINT('Ctrl Pts',(0.720020094497306,-1.04321801318649,
1.10166698368801));
#18953=CARTESIAN_POINT('Ctrl Pts',(0.823059514024041,-1.29188925333649,
1.31997051162989));
#18954=CARTESIAN_POINT('Ctrl Pts',(0.763527516695654,-1.54143100170428,
1.4989879457606));
#18955=CARTESIAN_POINT('Ctrl Pts',(0.541424102512144,-1.79184325828986,
1.63871928608013));
#18956=CARTESIAN_POINT('',(0.669228599956957,-0.849391336665505,1.28727233489076));
#18957=CARTESIAN_POINT('',(0.720159740047643,-1.03556549162895,1.10727038327973));
#18958=CARTESIAN_POINT('Ctrl Pts',(0.669228599956957,-0.849391336665505,
1.28727233489076));
#18959=CARTESIAN_POINT('Ctrl Pts',(0.691999639905454,-0.872888980165437,
1.25472274024255));
#18960=CARTESIAN_POINT('Ctrl Pts',(0.70368779557681,-0.897760310667366,
1.22803799031372));
#18961=CARTESIAN_POINT('Ctrl Pts',(0.717650427656666,-0.959132127442248,
1.17079203987312));
#18962=CARTESIAN_POINT('Ctrl Pts',(0.721400199597647,-0.994201051127665,
1.14052203161312));
#18963=CARTESIAN_POINT('Ctrl Pts',(0.720159740047643,-1.03556549162895,
1.10727038327973));
#18964=CARTESIAN_POINT('Ctrl Pts',(0.669228599956957,-0.849391336665505,
1.28727233489076));
#18965=CARTESIAN_POINT('Ctrl Pts',(0.713346345736856,-0.940530841324424,
1.39987124007464));
#18966=CARTESIAN_POINT('Ctrl Pts',(0.730332411016459,-1.03355488521186,
1.50346488650363));
#18967=CARTESIAN_POINT('Ctrl Pts',(0.707591441492496,-1.2462884798982,1.715480776583));
#18968=CARTESIAN_POINT('Ctrl Pts',(0.653180259586497,-1.36701797678012,
1.81902921434248));
#18969=CARTESIAN_POINT('Ctrl Pts',(0.556953250077769,-1.49065195897357,
1.90869858745619));
#18970=CARTESIAN_POINT('Ctrl Pts',(0.720159740047643,-1.03556549162895,
1.10727038327973));
#18971=CARTESIAN_POINT('Ctrl Pts',(0.752262754789917,-1.10996518478287,
1.17697999301248));
#18972=CARTESIAN_POINT('Ctrl Pts',(0.770456050723178,-1.19064632759639,
1.24430717677952));
#18973=CARTESIAN_POINT('Ctrl Pts',(0.768953495941756,-1.36932585223819,
1.37795460947453));
#18974=CARTESIAN_POINT('Ctrl Pts',(0.746322420853231,-1.46217959017504,
1.43952296396723));
#18975=CARTESIAN_POINT('Ctrl Pts',(0.667365107081636,-1.62949375452171,
1.54471868724302));
#18976=CARTESIAN_POINT('Ctrl Pts',(0.616426084068086,-1.70581792784517,
1.59041399531287));
#18977=CARTESIAN_POINT('Ctrl Pts',(0.549562141057364,-1.78098192700405,
1.63615580822897));
#18978=CARTESIAN_POINT('Ctrl Pts',(0.954059150195613,-0.834133412413726,
1.10192461715937));
#18979=CARTESIAN_POINT('Ctrl Pts',(1.11506945780848,-1.04978444082665,1.32030517702044));
#18980=CARTESIAN_POINT('Ctrl Pts',(1.11871269798568,-1.30624985183955,1.49938098964776));
#18981=CARTESIAN_POINT('Ctrl Pts',(0.96498887072721,-1.60352964545243,1.63915205504134));
#18982=CARTESIAN_POINT('Ctrl Pts',(0.909786283922669,-0.830120410746054,
1.13430265099723));
#18983=CARTESIAN_POINT('Ctrl Pts',(1.06188151028184,-1.04296293472434,1.35904945381842));
#18984=CARTESIAN_POINT('Ctrl Pts',(1.06009689157698,-1.29220976330375,1.54337045304296));
#18985=CARTESIAN_POINT('Ctrl Pts',(0.904675898434802,-1.5779663580892,1.68721036521566));
#18986=CARTESIAN_POINT('Ctrl Pts',(0.852548363463457,-0.818798046722487,
1.18072883129925));
#18987=CARTESIAN_POINT('Ctrl Pts',(0.993250080255865,-1.02679776283204,
1.41464170568302));
#18988=CARTESIAN_POINT('Ctrl Pts',(0.985477438725562,-1.26592128430496,
1.60649360709678));
#18989=CARTESIAN_POINT('Ctrl Pts',(0.829299566756361,-1.53630097399698,
1.75619511453864));
#18990=CARTESIAN_POINT('Ctrl Pts',(0.79375614980161,-0.790019116961202,
1.24117993109554));
#18991=CARTESIAN_POINT('Ctrl Pts',(0.923395339954023,-0.989381722131547,
1.48719616792706));
#18992=CARTESIAN_POINT('Ctrl Pts',(0.911933272667177,-1.21574497056749,
1.68893589783145));
#18993=CARTESIAN_POINT('Ctrl Pts',(0.759379860065507,-1.46910775939894,
1.84640075134781));
#18994=CARTESIAN_POINT('Ctrl Pts',(0.773880188435137,-0.771069384901099,
1.26847955290007));
#18995=CARTESIAN_POINT('Ctrl Pts',(0.900255846614141,-0.96560832231481,
1.51990601315848));
#18996=CARTESIAN_POINT('Ctrl Pts',(0.888894517998789,-1.18631348684325,
1.72616419407532));
#18997=CARTESIAN_POINT('Ctrl Pts',(0.739946404362065,-1.43341713701446,
1.88709951781478));
#18998=CARTESIAN_POINT('Ctrl Pts',(0.764532229061142,-0.75964933747155,
1.28318566992362));
#18999=CARTESIAN_POINT('Ctrl Pts',(0.889446983704125,-0.951396617529428,
1.53754047574671));
#19000=CARTESIAN_POINT('Ctrl Pts',(0.878600288371208,-1.16924120209866,
1.74612008846832));
#19001=CARTESIAN_POINT('Ctrl Pts',(0.731992143062391,-1.41318309117925,
1.90892450808845));
#19002=CARTESIAN_POINT('',(0.766529441696069,-0.762735325532963,1.28727233489076));
#19003=CARTESIAN_POINT('Ctrl Pts',(0.946792943618188,-0.833432097145897,
1.10727038327973));
#19004=CARTESIAN_POINT('Ctrl Pts',(0.920700076576133,-0.831623829941914,
1.12805083925439));
#19005=CARTESIAN_POINT('Ctrl Pts',(0.892688645988321,-0.827739845433019,
1.15131250789245));
#19006=CARTESIAN_POINT('Ctrl Pts',(0.848020576826707,-0.815788503303615,
1.19194777349474));
#19007=CARTESIAN_POINT('Ctrl Pts',(0.827793819033383,-0.809133178696747,
1.2110848927993));
#19008=CARTESIAN_POINT('Ctrl Pts',(0.796665168763682,-0.792014256883214,
1.24526606650786));
#19009=CARTESIAN_POINT('Ctrl Pts',(0.781636926589614,-0.781222353702314,
1.26352342884187));
#19010=CARTESIAN_POINT('Ctrl Pts',(0.766529441696069,-0.762735325532963,
1.28727233489076));
#19011=CARTESIAN_POINT('Ctrl Pts',(0.766529441696069,-0.762735325532963,
1.28727233489076));
#19012=CARTESIAN_POINT('Ctrl Pts',(0.821288554787752,-0.847907059902912,
1.39987124007464));
#19013=CARTESIAN_POINT('Ctrl Pts',(0.849339599532016,-0.938212862837218,
1.50346488650363));
#19014=CARTESIAN_POINT('Ctrl Pts',(0.852349824604395,-1.15213731807335,
1.715480776583));
#19015=CARTESIAN_POINT('Ctrl Pts',(0.812854124246772,-1.27853461941729,
1.81902921434248));
#19016=CARTESIAN_POINT('Ctrl Pts',(0.732195474855992,-1.41284463836769,
1.90869858745619));
#19017=CARTESIAN_POINT('Ctrl Pts',(0.766529441696069,-0.762735325532963,
1.28727233489076));
#19018=CARTESIAN_POINT('Ctrl Pts',(0.889651396707116,-0.954237887485568,
1.54044293163017));
#19019=CARTESIAN_POINT('Ctrl Pts',(0.877752552661174,-1.17169537927269,
1.74808806329354));
#19020=CARTESIAN_POINT('Ctrl Pts',(0.730832909558242,-1.41510780089433,
1.91020772988088));
#19021=CARTESIAN_POINT('Ctrl Pts',(0.734095827783031,-0.791620662577143,
1.28727233489076));
#19022=CARTESIAN_POINT('Ctrl Pts',(0.849242331321591,-0.987595926292982,
1.54044293163017));
#19023=CARTESIAN_POINT('Ctrl Pts',(0.828654188454018,-1.20405019596674,
1.74808806329354));
#19024=CARTESIAN_POINT('Ctrl Pts',(0.672331399180314,-1.44098347159841,
1.91020772988088));
#19025=CARTESIAN_POINT('Ctrl Pts',(0.701662213869994,-0.820505999621324,
1.28727233489076));
#19026=CARTESIAN_POINT('Ctrl Pts',(0.808833265936067,-1.0209539651004,1.54044293163017));
#19027=CARTESIAN_POINT('Ctrl Pts',(0.779555824246863,-1.23640501266079,
1.74808806329354));
#19028=CARTESIAN_POINT('Ctrl Pts',(0.613829888802385,-1.4668591423025,1.91020772988088));
#19029=CARTESIAN_POINT('Ctrl Pts',(0.669228599956957,-0.849391336665505,
1.28727233489076));
#19030=CARTESIAN_POINT('Ctrl Pts',(0.768424200550542,-1.05431200390781,
1.54044293163017));
#19031=CARTESIAN_POINT('Ctrl Pts',(0.730457460039708,-1.26875982935484,
1.74808806329354));
#19032=CARTESIAN_POINT('Ctrl Pts',(0.555328378424456,-1.49273481300659,
1.91020772988088));
#19033=CARTESIAN_POINT('Ctrl Pts',(0.766529441696069,-0.762735325532963,
1.28727233489076));
#19034=CARTESIAN_POINT('Ctrl Pts',(0.750680482155633,-0.777677426407099,
1.28796759655004));
#19035=CARTESIAN_POINT('Ctrl Pts',(0.734615936171903,-0.792391461327318,
1.2883190755065));
#19036=CARTESIAN_POINT('Ctrl Pts',(0.718338595112193,-0.806882581321257,
1.288319084765));
#19037=CARTESIAN_POINT('Ctrl Pts',(0.702161618687534,-0.821284350360125,
1.28831909396641));
#19038=CARTESIAN_POINT('Ctrl Pts',(0.685790724894005,-0.835451517520009,
1.28797193184368));
#19039=CARTESIAN_POINT('Ctrl Pts',(0.669228599956957,-0.849391336665505,
1.28727233489076));
#19040=CARTESIAN_POINT('Origin',(0.,0.,1.37171309575435));
#19041=CARTESIAN_POINT('',(0.642908916934714,-1.08521613661244,1.10727038327973));
#19042=CARTESIAN_POINT('Ctrl Pts',(0.428377445609996,-1.81394816223928,
1.63615580822897));
#19043=CARTESIAN_POINT('Ctrl Pts',(0.490704884304682,-1.75466459467969,
1.59808263051822));
#19044=CARTESIAN_POINT('Ctrl Pts',(0.544415468320011,-1.68908545531116,
1.55687869031203));
#19045=CARTESIAN_POINT('Ctrl Pts',(0.636822561166698,-1.52960471530762,
1.4528510278119));
#19046=CARTESIAN_POINT('Ctrl Pts',(0.665855105856972,-1.43800725813253,
1.39043708723109));
#19047=CARTESIAN_POINT('Ctrl Pts',(0.681216094986276,-1.25421153251789,
1.25222975809872));
#19048=CARTESIAN_POINT('Ctrl Pts',(0.668566409010631,-1.16714103226326,
1.18062438818012));
#19049=CARTESIAN_POINT('Ctrl Pts',(0.642908916934714,-1.08521613661244,
1.10727038327973));
#19050=CARTESIAN_POINT('Origin',(0.,0.,1.10727038327973));
#19051=CARTESIAN_POINT('Ctrl Pts',(0.373486051296586,-1.01098164380599,
1.28318517918604));
#19052=CARTESIAN_POINT('Ctrl Pts',(0.40602191942841,-1.23747555342209,1.537509268581));
#19053=CARTESIAN_POINT('Ctrl Pts',(0.304465327263429,-1.43047014156898,
1.74606924121326));
#19054=CARTESIAN_POINT('Ctrl Pts',(0.0688162748016435,-1.58996540824669,
1.90886509708284));
#19055=CARTESIAN_POINT('Ctrl Pts',(0.379996173302724,-1.02423814947078,
1.26846828789983));
#19056=CARTESIAN_POINT('Ctrl Pts',(0.413260018127926,-1.25379621584498,
1.51986220127974));
#19057=CARTESIAN_POINT('Ctrl Pts',(0.310691453231357,-1.44951276533331,
1.72609931925976));
#19058=CARTESIAN_POINT('Ctrl Pts',(0.0719956513773653,-1.61148865224617,
1.88702478432129));
#19059=CARTESIAN_POINT('Ctrl Pts',(0.388981181049686,-1.05021098685512,
1.24114793592828));
#19060=CARTESIAN_POINT('Ctrl Pts',(0.422993564147048,-1.28554831174898,
1.48712868773117));
#19061=CARTESIAN_POINT('Ctrl Pts',(0.317635541875722,-1.48619594640544,
1.68884366634831));
#19062=CARTESIAN_POINT('Ctrl Pts',(0.072903703454065,-1.65214688300286,
1.84629652534568));
#19063=CARTESIAN_POINT('Ctrl Pts',(0.390726670926086,-1.11570416593892,
1.18065052582665));
#19064=CARTESIAN_POINT('Ctrl Pts',(0.422167036078159,-1.36485769647199,
1.41452066958594));
#19065=CARTESIAN_POINT('Ctrl Pts',(0.307195656373209,-1.57470193347747,
1.6063408569219));
#19066=CARTESIAN_POINT('Ctrl Pts',(0.0456677490292576,-1.74530108095235,
1.75602521756879));
#19067=CARTESIAN_POINT('Ctrl Pts',(0.377231702026725,-1.17251250338939,
1.13419834492992));
#19068=CARTESIAN_POINT('Ctrl Pts',(0.40328175100029,-1.43283860087531,1.35889748756926));
#19069=CARTESIAN_POINT('Ctrl Pts',(0.277966085037659,-1.64835039139677,
1.54318426643097));
#19070=CARTESIAN_POINT('Ctrl Pts',(0.00100075866861844,-1.81900536712134,
1.68700348817738));
#19071=CARTESIAN_POINT('Ctrl Pts',(0.362468171451202,-1.21448591285885,
1.10179959977345));
#19072=CARTESIAN_POINT('Ctrl Pts',(0.383640993960513,-1.48279448162749,
1.32012924726704));
#19073=CARTESIAN_POINT('Ctrl Pts',(0.249943984819035,-1.7017123916886,1.49916808705051));
#19074=CARTESIAN_POINT('Ctrl Pts',(-0.0386228559732302,-1.87123964304219,
1.63891611912388));
#19075=CARTESIAN_POINT('',(0.373997862975653,-1.01462217612883,1.28727233489076));
#19076=CARTESIAN_POINT('',(0.364905277844141,-1.20742290720348,1.10727038327973));
#19077=CARTESIAN_POINT('Ctrl Pts',(0.373997862975653,-1.01462217612883,
1.28727233489076));
#19078=CARTESIAN_POINT('Ctrl Pts',(0.388393237732386,-1.04400640142099,
1.25472274024223));
#19079=CARTESIAN_POINT('Ctrl Pts',(0.39182367054918,-1.07127228109936,1.22803799031322));
#19080=CARTESIAN_POINT('Ctrl Pts',(0.38613798841402,-1.13395503795985,1.17079203987176));
#19081=CARTESIAN_POINT('Ctrl Pts',(0.3788673400596,-1.16846630960495,1.14052203161198));
#19082=CARTESIAN_POINT('Ctrl Pts',(0.364905277844141,-1.20742290720348,
1.10727038327973));
#19083=CARTESIAN_POINT('Ctrl Pts',(0.373997862975653,-1.01462217612883,
1.28727233489076));
#19084=CARTESIAN_POINT('Ctrl Pts',(0.387792676785358,-1.11493412912611,
1.39987124007464));
#19085=CARTESIAN_POINT('Ctrl Pts',(0.375201374409042,-1.20865423507634,
1.50346488650363));
#19086=CARTESIAN_POINT('Ctrl Pts',(0.287835131123855,-1.40394856048621,
1.715480776583));
#19087=CARTESIAN_POINT('Ctrl Pts',(0.198779555753984,-1.50195515531182,
1.81902921434248));
#19088=CARTESIAN_POINT('Ctrl Pts',(0.0690572297370875,-1.58980227845634,
1.90869858745619));
#19089=CARTESIAN_POINT('Ctrl Pts',(0.364905277844141,-1.20742290720348,
1.10727038327973));
#19090=CARTESIAN_POINT('Ctrl Pts',(0.372446289646659,-1.2881015973139,1.17697999301248));
#19091=CARTESIAN_POINT('Ctrl Pts',(0.364817298041905,-1.3704559615559,1.24430717677952));
#19092=CARTESIAN_POINT('Ctrl Pts',(0.30817327386479,-1.53992597283257,1.37795460947453));
#19093=CARTESIAN_POINT('Ctrl Pts',(0.257956459417354,-1.62124173855645,
1.43952296396723));
#19094=CARTESIAN_POINT('Ctrl Pts',(0.127450637982166,-1.75990988600071,
1.54779670475201));
#19095=CARTESIAN_POINT('Ctrl Pts',(0.0535283678677317,-1.81609416413933,
1.5933649555937));
#19096=CARTESIAN_POINT('Ctrl Pts',(-0.02768902675717,-1.86363850813291,
1.63615580822897));
#19097=CARTESIAN_POINT('Ctrl Pts',(0.649602771712747,-1.08812850838495,
1.10192461715937));
#19098=CARTESIAN_POINT('Ctrl Pts',(0.736092841324625,-1.34297974552473,
1.32030517702044));
#19099=CARTESIAN_POINT('Ctrl Pts',(0.660305598163236,-1.58801866900221,
1.49938098964776));
#19100=CARTESIAN_POINT('Ctrl Pts',(0.422241042228578,-1.82324527881739,
1.63915205504134));
#19101=CARTESIAN_POINT('Ctrl Pts',(0.618953337525113,-1.07500526379447,
1.12620814253776));
#19102=CARTESIAN_POINT('Ctrl Pts',(0.699675280139884,-1.3257887054316,1.34937307009661));
#19103=CARTESIAN_POINT('Ctrl Pts',(0.621781951952735,-1.56448518294015,
1.5323675387164));
#19104=CARTESIAN_POINT('Ctrl Pts',(0.385144875912206,-1.79103288048414,
1.67519578767208));
#19105=CARTESIAN_POINT('Ctrl Pts',(0.57206528258633,-1.04992951600932,1.16792267552994));
#19106=CARTESIAN_POINT('Ctrl Pts',(0.644197802222636,-1.29346620831953,
1.39930655296637));
#19107=CARTESIAN_POINT('Ctrl Pts',(0.563737612015952,-1.52169008642819,
1.58908853641613));
#19108=CARTESIAN_POINT('Ctrl Pts',(0.330550471617951,-1.73468787786898,
1.73717339980793));
#19109=CARTESIAN_POINT('Ctrl Pts',(0.518619720423095,-1.00746259753274,
1.2281482344299));
#19110=CARTESIAN_POINT('Ctrl Pts',(0.581479904896343,-1.23975486922368,
1.47154392632162));
#19111=CARTESIAN_POINT('Ctrl Pts',(0.500074721257065,-1.45417148278635,
1.67113467075223));
#19112=CARTESIAN_POINT('Ctrl Pts',(0.274410020975479,-1.65072103116967,
1.82691587671939));
#19113=CARTESIAN_POINT('Ctrl Pts',(0.499517401914415,-0.977055955806949,
1.26357751389222));
#19114=CARTESIAN_POINT('Ctrl Pts',(0.559692616049942,-1.20217681362938,
1.51402822523203));
#19115=CARTESIAN_POINT('Ctrl Pts',(0.480360559198655,-1.40948136690307,
1.71951214242025));
#19116=CARTESIAN_POINT('Ctrl Pts',(0.261218023549733,-1.59915063028856,
1.87982452105689));
#19117=CARTESIAN_POINT('Ctrl Pts',(0.49236880332188,-0.958722904028868,
1.28318566992362));
#19118=CARTESIAN_POINT('Ctrl Pts',(0.551916626543442,-1.17968618624264,
1.53754047574671));
#19119=CARTESIAN_POINT('Ctrl Pts',(0.47428312750236,-1.38351688474614,1.74612008846832));
#19120=CARTESIAN_POINT('Ctrl Pts',(0.259468306198631,-1.57021499953937,
1.90892450808845));
#19121=CARTESIAN_POINT('',(0.493314642657339,-0.962275025729455,1.28727233489076));
#19122=CARTESIAN_POINT('Ctrl Pts',(0.642908916934714,-1.08521613661244,
1.10727038327973));
#19123=CARTESIAN_POINT('Ctrl Pts',(0.618651911002038,-1.07543323295697,
1.12805083925432));
#19124=CARTESIAN_POINT('Ctrl Pts',(0.593211674629804,-1.06308333609217,
1.15131250789245));
#19125=CARTESIAN_POINT('Ctrl Pts',(0.554422984205302,-1.03791374180364,
1.19194777349641));
#19126=CARTESIAN_POINT('Ctrl Pts',(0.537242802809869,-1.0253337400692,1.21108489280038));
#19127=CARTESIAN_POINT('Ctrl Pts',(0.512927734894523,-0.999433395982646,
1.24526606650702));
#19128=CARTESIAN_POINT('Ctrl Pts',(0.501969908730686,-0.984525703912059,
1.26352342884097));
#19129=CARTESIAN_POINT('Ctrl Pts',(0.493314642657339,-0.962275025729455,
1.28727233489076));
#19130=CARTESIAN_POINT('Ctrl Pts',(0.493314642657339,-0.962275025729455,
1.28727233489076));
#19131=CARTESIAN_POINT('Ctrl Pts',(0.519074140629024,-1.06019965524839,
1.39987124007464));
#19132=CARTESIAN_POINT('Ctrl Pts',(0.517846241724568,-1.15475382712427,
1.50346488650363));
#19133=CARTESIAN_POINT('Ctrl Pts',(0.454602843714801,-1.35913828497575,
1.715480776583));
#19134=CARTESIAN_POINT('Ctrl Pts',(0.377981286365636,-1.46714441944577,
1.81902921434248));
#19135=CARTESIAN_POINT('Ctrl Pts',(0.259766273896473,-1.5699559447672,1.90869858745619));
#19136=CARTESIAN_POINT('Ctrl Pts',(0.493314642657339,-0.962275025729455,
1.28727233489076));
#19137=CARTESIAN_POINT('Ctrl Pts',(0.551233034159898,-1.18245156164078,
1.54044293163017));
#19138=CARTESIAN_POINT('Ctrl Pts',(0.472718500477254,-1.38558898119851,
1.74808806329354));
#19139=CARTESIAN_POINT('Ctrl Pts',(0.257771041609407,-1.57168728440264,
1.91020772988088));
#19140=CARTESIAN_POINT('Ctrl Pts',(0.453542382763444,-0.979724075862581,
1.28727233489076));
#19141=CARTESIAN_POINT('Ctrl Pts',(0.502493528317088,-1.20168985388846,
1.54044293163017));
#19142=CARTESIAN_POINT('Ctrl Pts',(0.416024993050258,-1.4011880115129,1.74808806329354));
#19143=CARTESIAN_POINT('Ctrl Pts',(0.194136776962956,-1.57821854873589,
1.91020772988088));
#19144=CARTESIAN_POINT('Ctrl Pts',(0.413770122869548,-0.997173125995706,
1.28727233489076));
#19145=CARTESIAN_POINT('Ctrl Pts',(0.453754022474278,-1.22092814613614,
1.54044293163017));
#19146=CARTESIAN_POINT('Ctrl Pts',(0.359331485623264,-1.41678704182728,
1.74808806329354));
#19147=CARTESIAN_POINT('Ctrl Pts',(0.130502512316506,-1.58474981306913,
1.91020772988088));
#19148=CARTESIAN_POINT('Ctrl Pts',(0.373997862975653,-1.01462217612883,
1.28727233489076));
#19149=CARTESIAN_POINT('Ctrl Pts',(0.405014516631467,-1.24016643838382,
1.54044293163017));
#19150=CARTESIAN_POINT('Ctrl Pts',(0.302637978196268,-1.43238607214167,
1.74808806329354));
#19151=CARTESIAN_POINT('Ctrl Pts',(0.0668682476700559,-1.59128107740238,
1.91020772988088));
#19152=CARTESIAN_POINT('Ctrl Pts',(0.493314642657339,-0.962275025729455,
1.28727233489076));
#19153=CARTESIAN_POINT('Ctrl Pts',(0.473624023308131,-0.971588210291789,
1.28796759655004));
#19154=CARTESIAN_POINT('Ctrl Pts',(0.45379884532281,-0.980617871367766,
1.2883190755065));
#19155=CARTESIAN_POINT('Ctrl Pts',(0.433840171694363,-0.989369770455727,
1.288319084765));
#19156=CARTESIAN_POINT('Ctrl Pts',(0.414004561469677,-0.998067706113493,
1.28831909396641));
#19157=CARTESIAN_POINT('Ctrl Pts',(0.394057020835224,-1.00648259836303,
1.28797193184368));
#19158=CARTESIAN_POINT('Ctrl Pts',(0.373997862975653,-1.01462217612883,
1.28727233489076));
#19159=CARTESIAN_POINT('Origin',(0.,0.,1.37171309575435));
#19160=CARTESIAN_POINT('',(0.27609248605185,-1.23077165948193,1.10727038327973));
#19161=CARTESIAN_POINT('Ctrl Pts',(-0.153129647965883,-1.85754313061971,
1.63615580822897));
#19162=CARTESIAN_POINT('Ctrl Pts',(-0.0607713534907783,-1.81335940151627,
1.59083969670469));
#19163=CARTESIAN_POINT('Ctrl Pts',(0.0223614442500381,-1.75708539039456,
1.54129005514746));
#19164=CARTESIAN_POINT('Ctrl Pts',(0.159600739735624,-1.61733286423933,
1.42521036359322));
#19165=CARTESIAN_POINT('Ctrl Pts',(0.208550308549108,-1.53789592166465,
1.36183966503053));
#19166=CARTESIAN_POINT('Ctrl Pts',(0.264206681902337,-1.37907079095174,
1.23219371736399));
#19167=CARTESIAN_POINT('Ctrl Pts',(0.275306576910198,-1.30454791379682,
1.17031259812849));
#19168=CARTESIAN_POINT('Ctrl Pts',(0.27609248605185,-1.23077165948193,1.10727038327973));
#19169=CARTESIAN_POINT('Origin',(0.,0.,1.10727038327973));
#19170=CARTESIAN_POINT('Ctrl Pts',(0.0427958338937929,-1.07691421720911,
1.28318517918604));
#19171=CARTESIAN_POINT('Ctrl Pts',(0.00374881610008805,-1.30237686203014,
1.53750926858099));
#19172=CARTESIAN_POINT('Ctrl Pts',(-0.15247585021093,-1.45454290982716,
1.74606924121326));
#19173=CARTESIAN_POINT('Ctrl Pts',(-0.42587816503926,-1.53341236060018,
1.90886509708283));
#19174=CARTESIAN_POINT('Ctrl Pts',(0.044892475801183,-1.091545040475,1.26845681306972));
#19175=CARTESIAN_POINT('Ctrl Pts',(0.00559080476410136,-1.32014932750452,
1.51984840181958));
#19176=CARTESIAN_POINT('Ctrl Pts',(-0.152438895007653,-1.4745930125769,
1.72608377212011));
#19177=CARTESIAN_POINT('Ctrl Pts',(-0.429508274607606,-1.55488138991364,
1.88700775532559));
#19178=CARTESIAN_POINT('Ctrl Pts',(0.0454099470705952,-1.11904054473513,
1.24111941924412));
#19179=CARTESIAN_POINT('Ctrl Pts',(0.00503268467650687,-1.35337649424567,
1.4870940232259));
#19180=CARTESIAN_POINT('Ctrl Pts',(-0.157175625948469,-1.51165038249934,
1.68880469124906));
#19181=CARTESIAN_POINT('Ctrl Pts',(-0.441219201568131,-1.59385438982847,
1.84625359892918));
#19182=CARTESIAN_POINT('Ctrl Pts',(0.0267999250011405,-1.18191630764682,
1.1805768626608));
#19183=CARTESIAN_POINT('Ctrl Pts',(-0.0203022432084527,-1.42860644524988,
1.41443159040039));
#19184=CARTESIAN_POINT('Ctrl Pts',(-0.194505783955952,-1.59265822923791,
1.60624053738541));
#19185=CARTESIAN_POINT('Ctrl Pts',(-0.495974904441967,-1.67408715628731,
1.7559150245411));
#19186=CARTESIAN_POINT('Ctrl Pts',(-0.00363238016698598,-1.23181557314521,
1.1340877844534));
#19187=CARTESIAN_POINT('Ctrl Pts',(-0.0593232212680527,-1.48747160844963,
1.35876508657128));
#19188=CARTESIAN_POINT('Ctrl Pts',(-0.245130498049611,-1.65371551508435,
1.54303391436825));
#19189=CARTESIAN_POINT('Ctrl Pts',(-0.561310568731037,-1.73041945202573,
1.68683916414418));
#19190=CARTESIAN_POINT('Ctrl Pts',(-0.0306796703370996,-1.26719829440569,
1.101666983688));
#19191=CARTESIAN_POINT('Ctrl Pts',(-0.0934843164788986,-1.52894260490194,
1.31997051162989));
#19192=CARTESIAN_POINT('Ctrl Pts',(-0.288323673548522,-1.69583409006838,
1.4989879457606));
#19193=CARTESIAN_POINT('Ctrl Pts',(-0.61519774154597,-1.76787274990501,
1.63871928608013));
#19194=CARTESIAN_POINT('',(0.0421576093699568,-1.08053472770428,1.28727233489076));
#19195=CARTESIAN_POINT('',(-0.0260686553993151,-1.26108935601086,1.10727038327973));
#19196=CARTESIAN_POINT('Ctrl Pts',(0.0421576093699568,-1.08053472770428,
1.28727233489076));
#19197=CARTESIAN_POINT('Ctrl Pts',(0.0467681993550376,-1.11292920208489,
1.25472274024224));
#19198=CARTESIAN_POINT('Ctrl Pts',(0.0416051146519907,-1.13992065666392,
1.22803799031328));
#19199=CARTESIAN_POINT('Ctrl Pts',(0.0168276724834171,-1.19777852863149,
1.17079203987139));
#19200=CARTESIAN_POINT('Ctrl Pts',(-0.000751694447691145,-1.22835394451355,
1.14052203161161));
#19201=CARTESIAN_POINT('Ctrl Pts',(-0.0260686553993153,-1.26108935601086,
1.10727038327973));
#19202=CARTESIAN_POINT('Ctrl Pts',(0.0421576093699568,-1.08053472770428,
1.28727233489076));
#19203=CARTESIAN_POINT('Ctrl Pts',(0.0242791587196548,-1.18019989616608,
1.39987124007464));
#19204=CARTESIAN_POINT('Ctrl Pts',(-0.0166569869072259,-1.26544208722232,
1.50346488650363));
#19205=CARTESIAN_POINT('Ctrl Pts',(-0.160096487344471,-1.42418037408903,
1.715480776583));
#19206=CARTESIAN_POINT('Ctrl Pts',(-0.275079075974333,-1.48987049850469,
1.81902921434248));
#19207=CARTESIAN_POINT('Ctrl Pts',(-0.425598593400272,-1.53333167412,1.90869858745619));
#19208=CARTESIAN_POINT('Ctrl Pts',(-0.0260686553993153,-1.26108935601086,
1.10727038327973));
#19209=CARTESIAN_POINT('Ctrl Pts',(-0.0438278133131018,-1.34014965076829,
1.17697999301248));
#19210=CARTESIAN_POINT('Ctrl Pts',(-0.0765323136032887,-1.41611581747018,
1.24430717677952));
#19211=CARTESIAN_POINT('Ctrl Pts',(-0.182773095427517,-1.55978740991095,
1.37795460947453));
#19212=CARTESIAN_POINT('Ctrl Pts',(-0.255660077554626,-1.62160544971255,
1.43952296396722));
#19213=CARTESIAN_POINT('Ctrl Pts',(-0.417882684528454,-1.71055550747297,
1.54471868724289));
#19214=CARTESIAN_POINT('Ctrl Pts',(-0.503955443296138,-1.74236185427976,
1.59041399531274));
#19215=CARTESIAN_POINT('Ctrl Pts',(-0.602229799711922,-1.76386916735271,
1.63615580822897));
#19216=CARTESIAN_POINT('Ctrl Pts',(0.281756991007075,-1.23578335387376,
1.1017328493151));
#19217=CARTESIAN_POINT('Ctrl Pts',(0.285293785520307,-1.50493278576873,
1.32007563441911));
#19218=CARTESIAN_POINT('Ctrl Pts',(0.137495264840177,-1.71461214828354,
1.4991204904476));
#19219=CARTESIAN_POINT('Ctrl Pts',(-0.161638571033313,-1.86482144141821,
1.63886741740056));
#19220=CARTESIAN_POINT('Ctrl Pts',(0.2566193137444,-1.21381148288727,1.12604029619216));
#19221=CARTESIAN_POINT('Ctrl Pts',(0.25591920404824,-1.47730375097777,1.34917212439386));
#19222=CARTESIAN_POINT('Ctrl Pts',(0.108074844008921,-1.68029140190124,
1.5321393304303));
#19223=CARTESIAN_POINT('Ctrl Pts',(-0.187017052056851,-1.82267525691206,
1.67494641070563));
#19224=CARTESIAN_POINT('Ctrl Pts',(0.219711749650112,-1.17543855297397,
1.16779612397805));
#19225=CARTESIAN_POINT('Ctrl Pts',(0.21307065152042,-1.42937433465483,1.39915507862236));
#19226=CARTESIAN_POINT('Ctrl Pts',(0.0660178837300413,-1.62159457256362,
1.58891631513415));
#19227=CARTESIAN_POINT('Ctrl Pts',(-0.221600535375876,-1.7521395453745,
1.73698522631426));
#19228=CARTESIAN_POINT('Ctrl Pts',(0.181934739915364,-1.11847368101377,
1.22808906223353));
#19229=CARTESIAN_POINT('Ctrl Pts',(0.169938151077974,-1.35883455739468,
1.47147297599239));
#19230=CARTESIAN_POINT('Ctrl Pts',(0.0262526925971304,-1.53761229859012,
1.67105384595181));
#19231=CARTESIAN_POINT('Ctrl Pts',(-0.249117593166629,-1.65481713073797,
1.82682748557709));
#19232=CARTESIAN_POINT('Ctrl Pts',(0.173143664137204,-1.08361696356336,
1.26355539141207));
#19233=CARTESIAN_POINT('Ctrl Pts',(0.160806376565823,-1.31631931390947,
1.51400180025811));
#19234=CARTESIAN_POINT('Ctrl Pts',(0.0212938283898079,-1.48896648444243,
1.71948206324579));
#19235=CARTESIAN_POINT('Ctrl Pts',(-0.245739828560967,-1.6016350942056,
1.87979168962264));
#19236=CARTESIAN_POINT('Ctrl Pts',(0.172008888578299,-1.06394999292458,
1.28318566992362));
#19237=CARTESIAN_POINT('Ctrl Pts',(0.160360824547434,-1.29249985168946,
1.53754047574671));
#19238=CARTESIAN_POINT('Ctrl Pts',(0.0235398295887214,-1.46236429518572,
1.74612008846832));
#19239=CARTESIAN_POINT('Ctrl Pts',(-0.238454096297838,-1.57354332341337,
1.90892450808845));
#19240=CARTESIAN_POINT('',(0.171810769270086,-1.06762054184321,1.28727233489076));
#19241=CARTESIAN_POINT('Ctrl Pts',(0.27609248605185,-1.23077165948193,1.10727038327973));
#19242=CARTESIAN_POINT('Ctrl Pts',(0.256045785977557,-1.21397173814618,
1.12805083925441));
#19243=CARTESIAN_POINT('Ctrl Pts',(0.235667011409714,-1.19436482287745,
1.15131250789248));
#19244=CARTESIAN_POINT('Ctrl Pts',(0.206554607000121,-1.15844075168674,
1.19194777349574));
#19245=CARTESIAN_POINT('Ctrl Pts',(0.194102717857772,-1.14116749104435,
1.21108489279997));
#19246=CARTESIAN_POINT('Ctrl Pts',(0.178981360555582,-1.10902103082124,
1.2452660665067));
#19247=CARTESIAN_POINT('Ctrl Pts',(0.173166578774629,-1.09145681862846,
1.26352342884077));
#19248=CARTESIAN_POINT('Ctrl Pts',(0.171810769270086,-1.06762054184321,
1.28727233489076));
#19249=CARTESIAN_POINT('Ctrl Pts',(0.171810769270086,-1.06762054184321,
1.28727233489076));
#19250=CARTESIAN_POINT('Ctrl Pts',(0.166049132983329,-1.16871252149279,
1.39987124007464));
#19251=CARTESIAN_POINT('Ctrl Pts',(0.135662485730195,-1.25825944116939,
1.50346488650363));
#19252=CARTESIAN_POINT('Ctrl Pts',(0.0123561690781436,-1.43309732687145,
1.715480776583));
#19253=CARTESIAN_POINT('Ctrl Pts',(-0.0938909933754473,-1.51213990150266,
1.81902921434248));
#19254=CARTESIAN_POINT('Ctrl Pts',(-0.238090659850088,-1.57338902476662,
1.90869858745619));
#19255=CARTESIAN_POINT('Ctrl Pts',(0.171810769270086,-1.06762054184321,
1.28727233489076));
#19256=CARTESIAN_POINT('Ctrl Pts',(0.158856141562724,-1.29491863831812,
1.54044293163017));
#19257=CARTESIAN_POINT('Ctrl Pts',(0.0214114678431581,-1.46385147967852,
1.74808806329354));
#19258=CARTESIAN_POINT('Ctrl Pts',(-0.240523251888612,-1.5744190659244,
1.91020772988088));
#19259=CARTESIAN_POINT('Ctrl Pts',(0.128593049303376,-1.07192527046357,
1.28727233489076));
#19260=CARTESIAN_POINT('Ctrl Pts',(0.106557157682628,-1.2981540059198,1.54044293163017));
#19261=CARTESIAN_POINT('Ctrl Pts',(-0.0373276272898297,-1.46116778184124,
1.74808806329354));
#19262=CARTESIAN_POINT('Ctrl Pts',(-0.303061305613997,-1.56096659822788,
1.91020772988088));
#19263=CARTESIAN_POINT('Ctrl Pts',(0.0853753293366665,-1.07622999908393,
1.28727233489076));
#19264=CARTESIAN_POINT('Ctrl Pts',(0.054258173802532,-1.30138937352148,
1.54044293163017));
#19265=CARTESIAN_POINT('Ctrl Pts',(-0.0960667224228173,-1.45848408400396,
1.74808806329354));
#19266=CARTESIAN_POINT('Ctrl Pts',(-0.365599359339382,-1.54751413053135,
1.91020772988088));
#19267=CARTESIAN_POINT('Ctrl Pts',(0.0421576093699568,-1.08053472770428,
1.28727233489076));
#19268=CARTESIAN_POINT('Ctrl Pts',(0.00195918992243604,-1.30462474112317,
1.54044293163017));
#19269=CARTESIAN_POINT('Ctrl Pts',(-0.154805817555805,-1.45580038616668,
1.74808806329354));
#19270=CARTESIAN_POINT('Ctrl Pts',(-0.428137413064767,-1.53406166283483,
1.91020772988088));
#19271=CARTESIAN_POINT('Ctrl Pts',(0.171810769270086,-1.06762054184321,
1.28727233489076));
#19272=CARTESIAN_POINT('Ctrl Pts',(0.150205945126601,-1.0703931707,1.28796759655004));
#19273=CARTESIAN_POINT('Ctrl Pts',(0.128560761691038,-1.07285457179227,
1.2883190755065));
#19274=CARTESIAN_POINT('Ctrl Pts',(0.106874449528872,-1.07501055311346,
1.288319084765));
#19275=CARTESIAN_POINT('Ctrl Pts',(0.0853218532357676,-1.07715324084587,
1.28831909396641));
#19276=CARTESIAN_POINT('Ctrl Pts',(0.0637502700203705,-1.07899214990168,
1.28797193184368));
#19277=CARTESIAN_POINT('Ctrl Pts',(0.0421576093699568,-1.08053472770428,
1.28727233489076));
#19278=CARTESIAN_POINT('Origin',(0.,0.,1.37171309575435));
#19279=CARTESIAN_POINT('',(-0.117749801015232,-1.25585067703094,1.10727038327973));
#19280=CARTESIAN_POINT('Ctrl Pts',(-0.719647344681869,-1.71930883511106,
1.63615580822897));
#19281=CARTESIAN_POINT('Ctrl Pts',(-0.634377380847188,-1.70798257074607,
1.59808263051822));
#19282=CARTESIAN_POINT('Ctrl Pts',(-0.552378154622127,-1.68649822169668,
1.55687869031203));
#19283=CARTESIAN_POINT('Ctrl Pts',(-0.383878819109611,-1.61179111914083,
1.4528510278119));
#19284=CARTESIAN_POINT('Ctrl Pts',(-0.306551362590219,-1.55475212125011,
1.3904370872311));
#19285=CARTESIAN_POINT('Ctrl Pts',(-0.186091644383524,-1.41508721860523,
1.25222975809872));
#19286=CARTESIAN_POINT('Ctrl Pts',(-0.145146699351922,-1.33721040532788,
1.18062438818012));
#19287=CARTESIAN_POINT('Ctrl Pts',(-0.117749801015232,-1.25585067703094,
1.10727038327973));
#19288=CARTESIAN_POINT('Origin',(0.,0.,1.10727038327973));
#19289=CARTESIAN_POINT('Ctrl Pts',(-0.292083537906633,-1.03743092372925,
1.28318517918604));
#19290=CARTESIAN_POINT('Ctrl Pts',(-0.398891247467646,-1.23979244918951,
1.53750926858099));
#19291=CARTESIAN_POINT('Ctrl Pts',(-0.594491629104921,-1.33623488367509,
1.74606924121325));
#19292=CARTESIAN_POINT('Ctrl Pts',(-0.878884682818457,-1.32675822718598,
1.90886509708283));
#19293=CARTESIAN_POINT('Ctrl Pts',(-0.294610685989129,-1.05199356151554,
1.26845681306972));
#19294=CARTESIAN_POINT('Ctrl Pts',(-0.402631406009321,-1.25726427409018,
1.51984840181957));
#19295=CARTESIAN_POINT('Ctrl Pts',(-0.600652305106666,-1.35531508433345,
1.72608377212011));
#19296=CARTESIAN_POINT('Ctrl Pts',(-0.888971417088892,-1.34605472186502,
1.88700775532558));
#19297=CARTESIAN_POINT('Ctrl Pts',(-0.302614092509142,-1.07830248703538,
1.241120378339));
#19298=CARTESIAN_POINT('Ctrl Pts',(-0.413428941810942,-1.28869195855348,
1.48709498232077));
#19299=CARTESIAN_POINT('Ctrl Pts',(-0.616606838701694,-1.38909450341185,
1.68880599613841));
#19300=CARTESIAN_POINT('Ctrl Pts',(-0.912150767476964,-1.3795008682383,
1.84625490381854));
#19301=CARTESIAN_POINT('Ctrl Pts',(-0.339741650892325,-1.13234954650477,
1.18057861631985));
#19302=CARTESIAN_POINT('Ctrl Pts',(-0.460769919763727,-1.35241043892923,
1.41443334405943));
#19303=CARTESIAN_POINT('Ctrl Pts',(-0.677140712937712,-1.4546018215964,
1.6062429176887));
#19304=CARTESIAN_POINT('Ctrl Pts',(-0.98901780672968,-1.43888625177221,
1.75591740484439));
#19305=CARTESIAN_POINT('Ctrl Pts',(-0.384106544865062,-1.17040376051197,
1.13408778445339));
#19306=CARTESIAN_POINT('Ctrl Pts',(-0.516073741815779,-1.39633768248717,
1.35876508657127));
#19307=CARTESIAN_POINT('Ctrl Pts',(-0.744159155535337,-1.49702742698244,
1.54303391436825));
#19308=CARTESIAN_POINT('Ctrl Pts',(-1.06856709212991,-1.4722721909128,1.68683916414418));
#19309=CARTESIAN_POINT('Ctrl Pts',(-0.420763908606196,-1.19569665581666,
1.101666983688));
#19310=CARTESIAN_POINT('Ctrl Pts',(-0.561378116697257,-1.42522258493377,
1.31997051162988));
#19311=CARTESIAN_POINT('Ctrl Pts',(-0.798253662001981,-1.52373714690789,
1.49898794576059));
#19312=CARTESIAN_POINT('Ctrl Pts',(-1.13139054452037,-1.49124034173901,
1.63871928608012));
#19313=CARTESIAN_POINT('',(-0.293809324770207,-1.04067701160391,1.28727233489076));
#19314=CARTESIAN_POINT('',(-0.414490807021284,-1.19131159212569,1.10727038327973));
#19315=CARTESIAN_POINT('Ctrl Pts',(-0.293809324770207,-1.04067701160391,
1.28727233489076));
#19316=CARTESIAN_POINT('Ctrl Pts',(-0.299434836228388,-1.07291073821506,
1.25472274024221));
#19317=CARTESIAN_POINT('Ctrl Pts',(-0.312686039747241,-1.09698565606009,
1.22803799031324));
#19318=CARTESIAN_POINT('Ctrl Pts',(-0.354129853274886,-1.14435511150628,
1.17079203987172));
#19319=CARTESIAN_POINT('Ctrl Pts',(-0.380297147864532,-1.16800173688728,
1.14052203161199));
#19320=CARTESIAN_POINT('Ctrl Pts',(-0.414490807021284,-1.19131159212569,
1.10727038327973));
#19321=CARTESIAN_POINT('Ctrl Pts',(-0.293809324770207,-1.04067701160391,
1.28727233489076));
#19322=CARTESIAN_POINT('Ctrl Pts',(-0.341610972564375,-1.12993947443311,
1.39987124007464));
#19323=CARTESIAN_POINT('Ctrl Pts',(-0.406884846288962,-1.19835965101752,
1.50346488650363));
#19324=CARTESIAN_POINT('Ctrl Pts',(-0.592356746173702,-1.30500348982786,
1.715480776583));
#19325=CARTESIAN_POINT('Ctrl Pts',(-0.722011051157661,-1.33194693676576,
1.81902921434248));
#19326=CARTESIAN_POINT('Ctrl Pts',(-0.878593860895847,-1.32676788217082,
1.90869858745619));
#19327=CARTESIAN_POINT('Ctrl Pts',(-0.414490807021284,-1.19131159212569,
1.10727038327973));
#19328=CARTESIAN_POINT('Ctrl Pts',(-0.455811744539447,-1.26101451903382,
1.17697999301248));
#19329=CARTESIAN_POINT('Ctrl Pts',(-0.510390409161016,-1.32315639051141,
1.24430717677953));
#19330=CARTESIAN_POINT('Ctrl Pts',(-0.655828360684357,-1.42696598762934,
1.37795460947454));
#19331=CARTESIAN_POINT('Ctrl Pts',(-0.744250824847073,-1.46323512106126,
1.43952296396723));
#19332=CARTESIAN_POINT('Ctrl Pts',(-0.926020771798391,-1.49770211069239,
1.54471868724282));
#19333=CARTESIAN_POINT('Ctrl Pts',(-1.01770953159214,-1.50135379887062,
1.59041399531267));
#19334=CARTESIAN_POINT('Ctrl Pts',(-1.11782012388912,-1.4914400228729,1.63615580822897));
#19335=CARTESIAN_POINT('Ctrl Pts',(-0.114046207919,-1.26214138440836,1.10192461715937));
#19336=CARTESIAN_POINT('Ctrl Pts',(-0.193872070477574,-1.51915795367953,
1.32030517702044));
#19337=CARTESIAN_POINT('Ctrl Pts',(-0.399215503609652,-1.67285198321399,
1.49938098964776));
#19338=CARTESIAN_POINT('Ctrl Pts',(-0.730076507315236,-1.72322347301172,
1.63915205504134));
#19339=CARTESIAN_POINT('Ctrl Pts',(-0.131128471412264,-1.23350917110671,
1.12620814253777));
#19340=CARTESIAN_POINT('Ctrl Pts',(-0.213229856531409,-1.48384440470435,
1.34937307009661));
#19341=CARTESIAN_POINT('Ctrl Pts',(-0.416549152036926,-1.63116936194583,
1.5323675387164));
#19342=CARTESIAN_POINT('Ctrl Pts',(-0.741153963610082,-1.67535851585319,
1.67519578767208));
#19343=CARTESIAN_POINT('Ctrl Pts',(-0.15432167232943,-1.18566161414104,
1.16792358645355));
#19344=CARTESIAN_POINT('Ctrl Pts',(-0.239112514228606,-1.42508536822678,
1.39930746388998));
#19345=CARTESIAN_POINT('Ctrl Pts',(-0.43835214562218,-1.56242925297243,
1.58908978141843));
#19346=CARTESIAN_POINT('Ctrl Pts',(-0.752201465653627,-1.59768412386216,
1.73717464481023));
#19347=CARTESIAN_POINT('Ctrl Pts',(-0.172598846101517,-1.11989042845005,
1.2281493040678));
#19348=CARTESIAN_POINT('Ctrl Pts',(-0.258281860114565,-1.34476711329974,
1.47154499595952));
#19349=CARTESIAN_POINT('Ctrl Pts',(-0.450170312236607,-1.47038505632136,
1.67113613169257));
#19350=CARTESIAN_POINT('Ctrl Pts',(-0.7482658156794,-1.49675459841166,1.82691733765973));
#19351=CARTESIAN_POINT('Ctrl Pts',(-0.17018101435307,-1.08406383481182,
1.26357751389222));
#19352=CARTESIAN_POINT('Ctrl Pts',(-0.253820963688731,-1.30156053800084,
1.51402822523203));
#19353=CARTESIAN_POINT('Ctrl Pts',(-0.439852505027495,-1.42264323155935,
1.71951214242026));
#19354=CARTESIAN_POINT('Ctrl Pts',(-0.728627336389063,-1.44728013834437,
1.87982452105689));
#19355=CARTESIAN_POINT('Ctrl Pts',(-0.165188454635723,-1.06503024353735,
1.28318566992362));
#19356=CARTESIAN_POINT('Ctrl Pts',(-0.246892212254841,-1.27879462627692,
1.53754047574671));
#19357=CARTESIAN_POINT('Ctrl Pts',(-0.429507710856701,-1.39806529952135,
1.74612008846832));
#19358=CARTESIAN_POINT('Ctrl Pts',(-0.713034950441302,-1.42284226327066,
1.90892450808846));
#19359=CARTESIAN_POINT('',(-0.166511139289342,-1.06845992077163,1.28727233489076));
#19360=CARTESIAN_POINT('Ctrl Pts',(-0.117749801015232,-1.25585067703094,
1.10727038327973));
#19361=CARTESIAN_POINT('Ctrl Pts',(-0.13162388455418,-1.23367823136726,
1.12805083925438));
#19362=CARTESIAN_POINT('Ctrl Pts',(-0.144946380875744,-1.20873355917046,
1.15131250789249));
#19363=CARTESIAN_POINT('Ctrl Pts',(-0.161532774289153,-1.16557150946376,
1.19194777349503));
#19364=CARTESIAN_POINT('Ctrl Pts',(-0.168037493511636,-1.14529581701476,
1.21108489279957));
#19365=CARTESIAN_POINT('Ctrl Pts',(-0.1724849563913,-1.11004996015836,1.24526606650726));
#19366=CARTESIAN_POINT('Ctrl Pts',(-0.172587502434316,-1.09154853530996,
1.26352342884133));
#19367=CARTESIAN_POINT('Ctrl Pts',(-0.166511139289342,-1.06845992077163,
1.28727233489076));
#19368=CARTESIAN_POINT('Ctrl Pts',(-0.166511139289342,-1.06845992077163,
1.28727233489076));
#19369=CARTESIAN_POINT('Ctrl Pts',(-0.203229920731113,-1.16282366323453,
1.39987124007464));
#19370=CARTESIAN_POINT('Ctrl Pts',(-0.259800859583567,-1.23859785430383,
1.50346488650363));
#19371=CARTESIAN_POINT('Ctrl Pts',(-0.431100013478375,-1.36677481743678,
1.715480776583));
#19372=CARTESIAN_POINT('Ctrl Pts',(-0.556572568507924,-1.40911659430225,
1.81902921434248));
#19373=CARTESIAN_POINT('Ctrl Pts',(-0.712641620935351,-1.42280782457595,
1.90869858745619));
#19374=CARTESIAN_POINT('Ctrl Pts',(-0.166511139289342,-1.06845992077163,
1.28727233489076));
#19375=CARTESIAN_POINT('Ctrl Pts',(-0.24907069698643,-1.28063005644821,
1.54044293163017));
#19376=CARTESIAN_POINT('Ctrl Pts',(-0.431991468445894,-1.3988219960746,
1.74808806329354));
#19377=CARTESIAN_POINT('Ctrl Pts',(-0.715273453667736,-1.42303573965083,
1.91020772988088));
#19378=CARTESIAN_POINT('Ctrl Pts',(-0.208943867782964,-1.05919895104906,
1.28727233489076));
#19379=CARTESIAN_POINT('Ctrl Pts',(-0.299809769973181,-1.26754579908091,
1.54044293163017));
#19380=CARTESIAN_POINT('Ctrl Pts',(-0.487026359393918,-1.37811826912839,
1.74808806329354));
#19381=CARTESIAN_POINT('Ctrl Pts',(-0.770593636045173,-1.39091636119152,
1.91020772988088));
#19382=CARTESIAN_POINT('Ctrl Pts',(-0.251376596276585,-1.04993798132648,
1.28727233489076));
#19383=CARTESIAN_POINT('Ctrl Pts',(-0.350548842959931,-1.25446154171361,
1.54044293163017));
#19384=CARTESIAN_POINT('Ctrl Pts',(-0.542061250341939,-1.35741454218218,
1.74808806329354));
#19385=CARTESIAN_POINT('Ctrl Pts',(-0.825913818422611,-1.35879698273221,
1.91020772988088));
#19386=CARTESIAN_POINT('Ctrl Pts',(-0.293809324770207,-1.04067701160391,
1.28727233489076));
#19387=CARTESIAN_POINT('Ctrl Pts',(-0.401287915946682,-1.24137728434631,
1.54044293163017));
#19388=CARTESIAN_POINT('Ctrl Pts',(-0.597096141289962,-1.33671081523597,
1.74808806329354));
#19389=CARTESIAN_POINT('Ctrl Pts',(-0.881234000800048,-1.3266776042729,
1.91020772988088));
#19390=CARTESIAN_POINT('Ctrl Pts',(-0.166511139289342,-1.06845992077163,
1.28727233489076));
#19391=CARTESIAN_POINT('Ctrl Pts',(-0.187915337510229,-1.06442058969234,
1.28796759655004));
#19392=CARTESIAN_POINT('Ctrl Pts',(-0.209261745030525,-1.06007279171241,
1.2883190755065));
#19393=CARTESIAN_POINT('Ctrl Pts',(-0.230552888394581,-1.05542181279351,
1.288319084765));
#19394=CARTESIAN_POINT('Ctrl Pts',(-0.251712752465177,-1.05079951139633,
1.28831909396641));
#19395=CARTESIAN_POINT('Ctrl Pts',(-0.272796801398346,-1.0458824320276,
1.28797193184368));
#19396=CARTESIAN_POINT('Ctrl Pts',(-0.293809324770207,-1.04067701160391,
1.28727233489076));
#19397=CARTESIAN_POINT('Origin',(0.,0.,1.37171309575435));
#19398=CARTESIAN_POINT('',(-0.500065917147839,-1.15799828028598,1.10727038327973));
#19399=CARTESIAN_POINT('Ctrl Pts',(-1.21572094522251,-1.4127766116927,1.63615580822897));
#19400=CARTESIAN_POINT('Ctrl Pts',(-1.13112438230172,-1.42835456209775,
1.59808263051822));
#19401=CARTESIAN_POINT('Ctrl Pts',(-1.04649945489987,-1.4332608863651,1.55687869031203));
#19402=CARTESIAN_POINT('Ctrl Pts',(-0.863161299579022,-1.41427936788009,
1.4528510278119));
#19403=CARTESIAN_POINT('Ctrl Pts',(-0.771992498477375,-1.38392755544946,
1.3904370872311));
#19404=CARTESIAN_POINT('Ctrl Pts',(-0.614269670090826,-1.2883224397548,
1.25222975809873));
#19405=CARTESIAN_POINT('Ctrl Pts',(-0.551263454538706,-1.22690987286759,
1.18062438818012));
#19406=CARTESIAN_POINT('Ctrl Pts',(-0.500065917147839,-1.15799828028598,
1.10727038327973));
#19407=CARTESIAN_POINT('Origin',(0.,0.,1.10727038327973));
#19408=CARTESIAN_POINT('Ctrl Pts',(-0.598371737951084,-0.896396663228496,
1.28318517918604));
#19409=CARTESIAN_POINT('Ctrl Pts',(-0.762485056494505,-1.05584851328028,
1.53750926858099));
#19410=CARTESIAN_POINT('Ctrl Pts',(-0.978314425275391,-1.08712687701302,
1.74606924121326));
#19411=CARTESIAN_POINT('Ctrl Pts',(-1.24585984429374,-0.990231754426695,
1.90886509708283));
#19412=CARTESIAN_POINT('Ctrl Pts',(-0.605275301161474,-0.9094656230848,
1.26845681306972));
#19413=CARTESIAN_POINT('Ctrl Pts',(-0.771441249464591,-1.0713094336526,
1.51984840181957));
#19414=CARTESIAN_POINT('Ctrl Pts',(-0.990069682591154,-1.1033694726,1.72608377212011));
#19415=CARTESIAN_POINT('Ctrl Pts',(-1.26141584343747,-1.00546683912554,
1.88700775532558));
#19416=CARTESIAN_POINT('Ctrl Pts',(-0.621016981690699,-0.932013737380383,
1.24112031232197));
#19417=CARTESIAN_POINT('Ctrl Pts',(-0.791422088358097,-1.09786234356421,
1.48709491630373));
#19418=CARTESIAN_POINT('Ctrl Pts',(-1.01568188386468,-1.13056538342228,
1.68880590632087));
#19419=CARTESIAN_POINT('Ctrl Pts',(-1.29379626687141,-1.03011319759961,
1.84625481400099));
#19420=CARTESIAN_POINT('Ctrl Pts',(-0.673028944353633,-0.971942506168048,
1.180578495595));
#19421=CARTESIAN_POINT('Ctrl Pts',(-0.856136223676178,-1.14383306000902,
1.41443322333459));
#19422=CARTESIAN_POINT('Ctrl Pts',(-1.0934960272972,-1.17416051125987,1.60624275382304));
#19423=CARTESIAN_POINT('Ctrl Pts',(-1.38525239147929,-1.0628387940333,1.75591724097873));
#19424=CARTESIAN_POINT('Ctrl Pts',(-0.726981684724073,-0.994424673117314,
1.1340877844534));
#19425=CARTESIAN_POINT('Ctrl Pts',(-0.922307368817375,-1.16852049530615,
1.35876508657128));
#19426=CARTESIAN_POINT('Ctrl Pts',(-1.17034433001555,-1.19379986392408,
1.54303391436826));
#19427=CARTESIAN_POINT('Ctrl Pts',(-1.4712248234064,-1.07000866982979,1.68683916414419));
#19428=CARTESIAN_POINT('Ctrl Pts',(-0.769660843866369,-1.00715189764781,
1.10166698368801));
#19429=CARTESIAN_POINT('Ctrl Pts',(-0.974320315501941,-1.18199184824263,
1.31997051162989));
#19430=CARTESIAN_POINT('Ctrl Pts',(-1.23004502025837,-1.20248619530708,
1.4989879457606));
#19431=CARTESIAN_POINT('Ctrl Pts',(-1.53683495813566,-1.06863493884117,
1.63871928608013));
#19432=CARTESIAN_POINT('',(-0.601016155111926,-0.89895057878464,1.28727233489076));
#19433=CARTESIAN_POINT('',(-0.762339710524743,-1.00491994924733,1.10727038327973));
#19434=CARTESIAN_POINT('Ctrl Pts',(-0.601016155111926,-0.89895057878464,
1.28727233489076));
#19435=CARTESIAN_POINT('Ctrl Pts',(-0.616327103756389,-0.927868295879621,
1.25472274024266));
#19436=CARTESIAN_POINT('Ctrl Pts',(-0.636369305963692,-0.946670056292108,
1.22803799031394));
#19437=CARTESIAN_POINT('Ctrl Pts',(-0.690422681628619,-0.978914242877335,
1.17079203986993));
#19438=CARTESIAN_POINT('Ctrl Pts',(-0.722616466765382,-0.993317381309037,
1.14052203160971));
#19439=CARTESIAN_POINT('Ctrl Pts',(-0.762339710524743,-1.00491994924733,
1.10727038327973));
#19440=CARTESIAN_POINT('Ctrl Pts',(-0.601016155111926,-0.89895057878464,
1.28727233489076));
#19441=CARTESIAN_POINT('Ctrl Pts',(-0.674061841710201,-0.969072704191387,
1.39987124007464));
#19442=CARTESIAN_POINT('Ctrl Pts',(-0.757283981982513,-1.01397342270847,
1.50346488650363));
#19443=CARTESIAN_POINT('Ctrl Pts',(-0.966632999495317,-1.05808377148838,
1.715480776583));
#19444=CARTESIAN_POINT('Ctrl Pts',(-1.09826755410688,-1.04364312863621,
1.81902921434248));
#19445=CARTESIAN_POINT('Ctrl Pts',(-1.24558623976355,-0.990330805779365,
1.90869858745619));
#19446=CARTESIAN_POINT('Ctrl Pts',(-0.762339710524744,-1.00491994924733,
1.10727038327973));
#19447=CARTESIAN_POINT('Ctrl Pts',(-0.823177646383102,-1.05844250017153,
1.17697999301248));
#19448=CARTESIAN_POINT('Ctrl Pts',(-0.894287935370968,-1.10067719707671,
1.24430717677952));
#19449=CARTESIAN_POINT('Ctrl Pts',(-1.06468657657252,-1.15446319222191,
1.37795460947454));
#19450=CARTESIAN_POINT('Ctrl Pts',(-1.15998911590306,-1.16163314380192,
1.43952296396723));
#19451=CARTESIAN_POINT('Ctrl Pts',(-1.343513493959,-1.13824319621306,1.544718687243));
#19452=CARTESIAN_POINT('Ctrl Pts',(-1.43184312013715,-1.1133827730809,1.59041399531284));
#19453=CARTESIAN_POINT('Ctrl Pts',(-1.5239904260293,-1.07301833748062,1.63615580822897));
#19454=CARTESIAN_POINT('Ctrl Pts',(-0.498487526286222,-1.16512557173636,
1.10192461715937));
#19455=CARTESIAN_POINT('Ctrl Pts',(-0.653828920782166,-1.38489530661629,
1.32030517702043));
#19456=CARTESIAN_POINT('Ctrl Pts',(-0.896616198000942,-1.46761240439959,
1.49938098964774));
#19457=CARTESIAN_POINT('Ctrl Pts',(-1.22684935794255,-1.41327686508626,
1.63915205504132));
#19458=CARTESIAN_POINT('Ctrl Pts',(-0.50588588379779,-1.13261600897808,
1.12620814253777));
#19459=CARTESIAN_POINT('Ctrl Pts',(-0.661326782584696,-1.34532824088583,
1.3493730700966));
#19460=CARTESIAN_POINT('Ctrl Pts',(-0.900220838946918,-1.42261348388769,
1.53236753871639));
#19461=CARTESIAN_POINT('Ctrl Pts',(-1.22259355973873,-1.3643314634289,1.67519578767207));
#19462=CARTESIAN_POINT('Ctrl Pts',(-0.513157335393553,-1.07994282031223,
1.16792434557146));
#19463=CARTESIAN_POINT('Ctrl Pts',(-0.667784226973451,-1.2814465306771,
1.39930822300788));
#19464=CARTESIAN_POINT('Ctrl Pts',(-0.89971350073337,-1.35050022373304,
1.58909081893482));
#19465=CARTESIAN_POINT('Ctrl Pts',(-1.20909629592348,-1.28704482486114,
1.73717568232662));
#19466=CARTESIAN_POINT('Ctrl Pts',(-0.5102156806996,-1.01174252544333,1.22815018770195));
#19467=CARTESIAN_POINT('Ctrl Pts',(-0.661195786769765,-1.19913545447318,
1.47154587959366));
#19468=CARTESIAN_POINT('Ctrl Pts',(-0.882510125799198,-1.25930861084253,
1.67113733858628));
#19469=CARTESIAN_POINT('Ctrl Pts',(-1.17416443346652,-1.19227095916867,
1.82691854455344));
#19470=CARTESIAN_POINT('Ctrl Pts',(-0.496845910594337,-0.978417148622633,
1.26357751389222));
#19471=CARTESIAN_POINT('Ctrl Pts',(-0.643602406938536,-1.15942263970987,
1.51402822523202));
#19472=CARTESIAN_POINT('Ctrl Pts',(-0.857945526599457,-1.21709221666582,
1.71951214242024));
#19473=CARTESIAN_POINT('Ctrl Pts',(-1.1401999345933,-1.15128697696661,1.87982452105687));
#19474=CARTESIAN_POINT('Ctrl Pts',(-0.486216000974361,-0.961857913410637,
1.28318566992362));
#19475=CARTESIAN_POINT('Ctrl Pts',(-0.629977719122413,-1.13991207295831,
1.5375404757467));
#19476=CARTESIAN_POINT('Ctrl Pts',(-0.840512044007258,-1.19691393144611,
1.7461200884683));
#19477=CARTESIAN_POINT('Ctrl Pts',(-1.1178189756289,-1.13286348887406,1.90892450808843));
#19478=CARTESIAN_POINT('',(-0.488533777383804,-0.964710998256926,1.28727233489076));
#19479=CARTESIAN_POINT('Ctrl Pts',(-0.500065917147839,-1.15799828028598,
1.10727038327973));
#19480=CARTESIAN_POINT('Ctrl Pts',(-0.506409292188217,-1.13262370376054,
1.12805083925429));
#19481=CARTESIAN_POINT('Ctrl Pts',(-0.511371411500259,-1.10478303295006,
1.15131250789239));
#19482=CARTESIAN_POINT('Ctrl Pts',(-0.513808202166494,-1.05860800687958,
1.19194777349505));
#19483=CARTESIAN_POINT('Ctrl Pts',(-0.513729024230272,-1.03731460867033,
1.21108489279944));
#19484=CARTESIAN_POINT('Ctrl Pts',(-0.507067244033084,-1.00241946522331,
1.24526606650682));
#19485=CARTESIAN_POINT('Ctrl Pts',(-0.501447516417348,-0.984791876090384,
1.26352342884092));
#19486=CARTESIAN_POINT('Ctrl Pts',(-0.488533777383804,-0.964710998256926,
1.28727233489076));
#19487=CARTESIAN_POINT('Ctrl Pts',(-0.488533777383804,-0.964710998256925,
1.28727233489076));
#19488=CARTESIAN_POINT('Ctrl Pts',(-0.552615413818275,-1.04310952295002,
1.39987124007464));
#19489=CARTESIAN_POINT('Ctrl Pts',(-0.629833086622262,-1.09769367964031,
1.50346488650363));
#19490=CARTESIAN_POINT('Ctrl Pts',(-0.832357123065218,-1.16666286599128,
1.715480776583));
#19491=CARTESIAN_POINT('Ctrl Pts',(-0.964772942765737,-1.16815913695893,
1.81902921434248));
#19492=CARTESIAN_POINT('Ctrl Pts',(-1.11743425489732,-1.13295228123076,
1.90869858745619));
#19493=CARTESIAN_POINT('Ctrl Pts',(-0.488533777383804,-0.964710998256926,
1.28727233489076));
#19494=CARTESIAN_POINT('Ctrl Pts',(-0.632616760336964,-1.14098448197888,
1.54044293163017));
#19495=CARTESIAN_POINT('Ctrl Pts',(-0.843108069941918,-1.19686606932897,
1.74808806329354));
#19496=CARTESIAN_POINT('Ctrl Pts',(-1.12000770619867,-1.13235576030722,
1.91020772988088));
#19497=CARTESIAN_POINT('Ctrl Pts',(-0.526027903293178,-0.94279085843283,
1.28727233489076));
#19498=CARTESIAN_POINT('Ctrl Pts',(-0.676829228446517,-1.11286137791709,
1.54044293163017));
#19499=CARTESIAN_POINT('Ctrl Pts',(-0.889051558128351,-1.16016893831867,
1.74808806329354));
#19500=CARTESIAN_POINT('Ctrl Pts',(-1.16269489233868,-1.08471353963759,
1.91020772988088));
#19501=CARTESIAN_POINT('Ctrl Pts',(-0.563522029202552,-0.920870718608735,
1.28727233489076));
#19502=CARTESIAN_POINT('Ctrl Pts',(-0.721041696556071,-1.0847382738553,
1.54044293163017));
#19503=CARTESIAN_POINT('Ctrl Pts',(-0.934995046314783,-1.12347180730837,
1.74808806329354));
#19504=CARTESIAN_POINT('Ctrl Pts',(-1.20538207847869,-1.03707131896797,
1.91020772988088));
#19505=CARTESIAN_POINT('Ctrl Pts',(-0.601016155111926,-0.89895057878464,
1.28727233489076));
#19506=CARTESIAN_POINT('Ctrl Pts',(-0.765254164665624,-1.05661516979351,
1.54044293163017));
#19507=CARTESIAN_POINT('Ctrl Pts',(-0.980938534501216,-1.08677467629807,
1.74808806329354));
#19508=CARTESIAN_POINT('Ctrl Pts',(-1.2480692646187,-0.989429098298345,
1.91020772988088));
#19509=CARTESIAN_POINT('Ctrl Pts',(-0.488533777383804,-0.964710998256926,
1.28727233489076));
#19510=CARTESIAN_POINT('Ctrl Pts',(-0.507642157628474,-0.954255105111254,
1.28796759655004));
#19511=CARTESIAN_POINT('Ctrl Pts',(-0.526600254136219,-0.943523700818285,
1.2883190755065));
#19512=CARTESIAN_POINT('Ctrl Pts',(-0.545412103245543,-0.932521031881151,
1.288319084765));
#19513=CARTESIAN_POINT('Ctrl Pts',(-0.564107960168956,-0.921586204420602,
1.28831909396641));
#19514=CARTESIAN_POINT('Ctrl Pts',(-0.58264062120911,-0.910394454615247,
1.28797193184368));
#19515=CARTESIAN_POINT('Ctrl Pts',(-0.601016155111926,-0.89895057878464,
1.28727233489076));
#19516=CARTESIAN_POINT('Origin',(0.,0.,1.37171309575435));
#19517=CARTESIAN_POINT('',(-0.833432097145896,-0.946792943618189,1.10727038327973));
#19518=CARTESIAN_POINT('Ctrl Pts',(-1.59279130921887,-0.967951970128403,
1.63615580822897));
#19519=CARTESIAN_POINT('Ctrl Pts',(-1.51714904820957,-1.00890925697988,
1.59808263051822));
#19520=CARTESIAN_POINT('Ctrl Pts',(-1.43818209714157,-1.03972598936032,
1.55687869031203));
#19521=CARTESIAN_POINT('Ctrl Pts',(-1.25795153804723,-1.07832809822747,
1.4528510278119));
#19522=CARTESIAN_POINT('Ctrl Pts',(-1.16186562982554,-1.07763451813115,
1.3904370872311));
#19523=CARTESIAN_POINT('Ctrl Pts',(-0.982318700621179,-1.03544768423091,
1.25222975809873));
#19524=CARTESIAN_POINT('Ctrl Pts',(-0.903418701916908,-0.996510853667279,
1.18062438818012));
#19525=CARTESIAN_POINT('Ctrl Pts',(-0.833432097145896,-0.946792943618189,
1.10727038327973));
#19526=CARTESIAN_POINT('Origin',(0.,0.,1.10727038327973));
#19527=CARTESIAN_POINT('Ctrl Pts',(-0.846087143183836,-0.667616851768136,
1.28318517918604));
#19528=CARTESIAN_POINT('Ctrl Pts',(-1.05144151564591,-0.768550768362021,
1.53750926858099));
#19529=CARTESIAN_POINT('Ctrl Pts',(-1.26637298918249,-0.731603317170575,
1.74606924121326));
#19530=CARTESIAN_POINT('Ctrl Pts',(-1.4908815637936,-0.556774498193799,
1.90886509708283));
#19531=CARTESIAN_POINT('Ctrl Pts',(-0.856691352655136,-0.677912852846922,
1.26845681306972));
#19532=CARTESIAN_POINT('Ctrl Pts',(-1.06473704847503,-0.780487361597375,
1.51984840181957));
#19533=CARTESIAN_POINT('Ctrl Pts',(-1.28257214132251,-0.743418369261301,
1.72608377212011));
#19534=CARTESIAN_POINT('Ctrl Pts',(-1.5103840982294,-0.566456856673053,
1.88700775532558));
#19535=CARTESIAN_POINT('Ctrl Pts',(-0.878631748253101,-0.694492950134682,
1.24111924840996));
#19536=CARTESIAN_POINT('Ctrl Pts',(-1.0919466731633,-0.799566273875773,
1.48709385239173));
#19537=CARTESIAN_POINT('Ctrl Pts',(-1.31533666464121,-0.761367941758639,
1.68880445881716));
#19538=CARTESIAN_POINT('Ctrl Pts',(-1.54879772833386,-0.579890165126717,
1.84625336649729));
#19539=CARTESIAN_POINT('Ctrl Pts',(-0.940438249469776,-0.716394511678365,
1.18057655035132));
#19540=CARTESIAN_POINT('Ctrl Pts',(-1.16770072295994,-0.823288881893975,
1.4144312780909));
#19541=CARTESIAN_POINT('Ctrl Pts',(-1.4028158039603,-0.778782224872495,
1.60624011348192));
#19542=CARTESIAN_POINT('Ctrl Pts',(-1.64589229282025,-0.582751305549683,
1.75591460063762));
#19543=CARTESIAN_POINT('Ctrl Pts',(-0.998694792103063,-0.721104370153831,
1.1340877844534));
#19544=CARTESIAN_POINT('Ctrl Pts',(-1.23825912446583,-0.826320380483539,
1.35876508657128));
#19545=CARTESIAN_POINT('Ctrl Pts',(-1.48196804720542,-0.773714852492101,
1.54303391436825));
#19546=CARTESIAN_POINT('Ctrl Pts',(-1.72986881834179,-0.563005244955079,
1.68683916414418));
#19547=CARTESIAN_POINT('Ctrl Pts',(-1.04321801318649,-0.720020094497307,
1.10166698368801));
#19548=CARTESIAN_POINT('Ctrl Pts',(-1.2918892533365,-0.823059514024041,
1.31997051162989));
#19549=CARTESIAN_POINT('Ctrl Pts',(-1.5414310017043,-0.763527516695652,
1.4989879457606));
#19550=CARTESIAN_POINT('Ctrl Pts',(-1.79184325828987,-0.541424102512139,
1.63871928608013));
#19551=CARTESIAN_POINT('',(-0.849391336665505,-0.669228599956957,1.28727233489076));
#19552=CARTESIAN_POINT('',(-1.03556549162895,-0.720159740047643,1.10727038327973));
#19553=CARTESIAN_POINT('Ctrl Pts',(-0.849391336665505,-0.669228599956957,
1.28727233489076));
#19554=CARTESIAN_POINT('Ctrl Pts',(-0.872888980165412,-0.69199963990543,
1.25472274024258));
#19555=CARTESIAN_POINT('Ctrl Pts',(-0.897760310667151,-0.70368779557676,
1.22803799031392));
#19556=CARTESIAN_POINT('Ctrl Pts',(-0.959132127442685,-0.717650427656767,
1.17079203987271));
#19557=CARTESIAN_POINT('Ctrl Pts',(-0.994201051128119,-0.721400199597632,
1.14052203161276));
#19558=CARTESIAN_POINT('Ctrl Pts',(-1.03556549162895,-0.720159740047643,
1.10727038327973));
#19559=CARTESIAN_POINT('Ctrl Pts',(-0.849391336665505,-0.669228599956957,
1.28727233489076));
#19560=CARTESIAN_POINT('Ctrl Pts',(-0.940530841324424,-0.713346345736856,
1.39987124007464));
#19561=CARTESIAN_POINT('Ctrl Pts',(-1.03355488521186,-0.73033241101646,
1.50346488650363));
#19562=CARTESIAN_POINT('Ctrl Pts',(-1.2462884798982,-0.707591441492497,
1.715480776583));
#19563=CARTESIAN_POINT('Ctrl Pts',(-1.36701797678012,-0.653180259586497,
1.81902921434248));
#19564=CARTESIAN_POINT('Ctrl Pts',(-1.49065195897357,-0.55695325007777,
1.90869858745619));
#19565=CARTESIAN_POINT('Ctrl Pts',(-1.03556549162895,-0.720159740047643,
1.10727038327973));
#19566=CARTESIAN_POINT('Ctrl Pts',(-1.10996518478287,-0.752262754789918,
1.17697999301248));
#19567=CARTESIAN_POINT('Ctrl Pts',(-1.19064632759639,-0.770456050723179,
1.24430717677953));
#19568=CARTESIAN_POINT('Ctrl Pts',(-1.36932585223819,-0.768953495941756,
1.37795460947454));
#19569=CARTESIAN_POINT('Ctrl Pts',(-1.46217959017504,-0.746322420853231,
1.43952296396723));
#19570=CARTESIAN_POINT('Ctrl Pts',(-1.62949375452151,-0.667365107081731,
1.5447186872429));
#19571=CARTESIAN_POINT('Ctrl Pts',(-1.70581792784496,-0.616426084068271,
1.59041399531275));
#19572=CARTESIAN_POINT('Ctrl Pts',(-1.78098192700405,-0.549562141057365,
1.63615580822897));
#19573=CARTESIAN_POINT('Ctrl Pts',(-0.834133412413726,-0.954059150195613,
1.10192461715937));
#19574=CARTESIAN_POINT('Ctrl Pts',(-1.04978444082665,-1.11506945780848,
1.32030517702043));
#19575=CARTESIAN_POINT('Ctrl Pts',(-1.30624985183955,-1.11871269798568,
1.49938098964775));
#19576=CARTESIAN_POINT('Ctrl Pts',(-1.60352964545242,-0.964988870727218,
1.63915205504133));
#19577=CARTESIAN_POINT('Ctrl Pts',(-0.830120410746055,-0.909786283922666,
1.13430265099723));
#19578=CARTESIAN_POINT('Ctrl Pts',(-1.04296293472434,-1.06188151028183,
1.35904945381841));
#19579=CARTESIAN_POINT('Ctrl Pts',(-1.29220976330374,-1.06009689157698,
1.54337045304295));
#19580=CARTESIAN_POINT('Ctrl Pts',(-1.57796635808919,-0.904675898434815,
1.68721036521564));
#19581=CARTESIAN_POINT('Ctrl Pts',(-0.818798046722494,-0.852548363463462,
1.18072883129925));
#19582=CARTESIAN_POINT('Ctrl Pts',(-1.02679776283204,-0.993250080255868,
1.41464170568302));
#19583=CARTESIAN_POINT('Ctrl Pts',(-1.26592128430496,-0.985477438725565,
1.60649360709678));
#19584=CARTESIAN_POINT('Ctrl Pts',(-1.53630097399697,-0.82929956675637,
1.75619511453864));
#19585=CARTESIAN_POINT('Ctrl Pts',(-0.790019116961201,-0.793756149801608,
1.24117993109554));
#19586=CARTESIAN_POINT('Ctrl Pts',(-0.989381722131543,-0.923395339954019,
1.48719616792706));
#19587=CARTESIAN_POINT('Ctrl Pts',(-1.21574497056748,-0.911933272667178,
1.68893589783144));
#19588=CARTESIAN_POINT('Ctrl Pts',(-1.46910775939892,-0.759379860065515,
1.84640075134779));
#19589=CARTESIAN_POINT('Ctrl Pts',(-0.771069384901098,-0.773880188435137,
1.26847955290007));
#19590=CARTESIAN_POINT('Ctrl Pts',(-0.965608322314806,-0.900255846614139,
1.51990601315847));
#19591=CARTESIAN_POINT('Ctrl Pts',(-1.18631348684325,-0.88889451799879,
1.72616419407531));
#19592=CARTESIAN_POINT('Ctrl Pts',(-1.43341713701445,-0.739946404362073,
1.88709951781477));
#19593=CARTESIAN_POINT('Ctrl Pts',(-0.75964933747155,-0.764532229061142,
1.28318566992362));
#19594=CARTESIAN_POINT('Ctrl Pts',(-0.951396617529425,-0.889446983704123,
1.5375404757467));
#19595=CARTESIAN_POINT('Ctrl Pts',(-1.16924120209865,-0.878600288371209,
1.74612008846831));
#19596=CARTESIAN_POINT('Ctrl Pts',(-1.41318309117923,-0.731992143062398,
1.90892450808844));
#19597=CARTESIAN_POINT('',(-0.762735325532963,-0.766529441696069,1.28727233489076));
#19598=CARTESIAN_POINT('Ctrl Pts',(-0.833432097145896,-0.946792943618189,
1.10727038327973));
#19599=CARTESIAN_POINT('Ctrl Pts',(-0.831623829941906,-0.920700076575993,
1.12805083925451));
#19600=CARTESIAN_POINT('Ctrl Pts',(-0.827739845432993,-0.892688645988233,
1.15131250789253));
#19601=CARTESIAN_POINT('Ctrl Pts',(-0.815788503303453,-0.848020576826098,
1.19194777349529));
#19602=CARTESIAN_POINT('Ctrl Pts',(-0.809133178696535,-0.827793819032994,
1.21108489279973));
#19603=CARTESIAN_POINT('Ctrl Pts',(-0.792014256883054,-0.796665168763393,
1.24526606650818));
#19604=CARTESIAN_POINT('Ctrl Pts',(-0.781222353702122,-0.781636926589459,
1.26352342884212));
#19605=CARTESIAN_POINT('Ctrl Pts',(-0.762735325532963,-0.766529441696069,
1.28727233489076));
#19606=CARTESIAN_POINT('Ctrl Pts',(-0.762735325532963,-0.766529441696069,
1.28727233489076));
#19607=CARTESIAN_POINT('Ctrl Pts',(-0.847907059902912,-0.821288554787752,
1.39987124007464));
#19608=CARTESIAN_POINT('Ctrl Pts',(-0.938212862837218,-0.849339599532016,
1.50346488650363));
#19609=CARTESIAN_POINT('Ctrl Pts',(-1.15213731807335,-0.852349824604395,
1.715480776583));
#19610=CARTESIAN_POINT('Ctrl Pts',(-1.27853461941729,-0.812854124246773,
1.81902921434248));
#19611=CARTESIAN_POINT('Ctrl Pts',(-1.41284463836769,-0.732195474855993,
1.90869858745619));
#19612=CARTESIAN_POINT('Ctrl Pts',(-0.762735325532963,-0.766529441696069,
1.28727233489076));
#19613=CARTESIAN_POINT('Ctrl Pts',(-0.954237887485567,-0.889651396707116,
1.54044293163017));
#19614=CARTESIAN_POINT('Ctrl Pts',(-1.17169537927269,-0.877752552661174,
1.74808806329354));
#19615=CARTESIAN_POINT('Ctrl Pts',(-1.41510780089433,-0.730832909558243,
1.91020772988088));
#19616=CARTESIAN_POINT('Ctrl Pts',(-0.791620662577143,-0.734095827783031,
1.28727233489076));
#19617=CARTESIAN_POINT('Ctrl Pts',(-0.987595926292982,-0.849242331321591,
1.54044293163017));
#19618=CARTESIAN_POINT('Ctrl Pts',(-1.20405019596674,-0.828654188454019,
1.74808806329354));
#19619=CARTESIAN_POINT('Ctrl Pts',(-1.44098347159841,-0.672331399180314,
1.91020772988088));
#19620=CARTESIAN_POINT('Ctrl Pts',(-0.820505999621324,-0.701662213869994,
1.28727233489076));
#19621=CARTESIAN_POINT('Ctrl Pts',(-1.0209539651004,-0.808833265936067,
1.54044293163017));
#19622=CARTESIAN_POINT('Ctrl Pts',(-1.23640501266079,-0.779555824246864,
1.74808806329354));
#19623=CARTESIAN_POINT('Ctrl Pts',(-1.4668591423025,-0.613829888802386,
1.91020772988088));
#19624=CARTESIAN_POINT('Ctrl Pts',(-0.849391336665505,-0.669228599956957,
1.28727233489076));
#19625=CARTESIAN_POINT('Ctrl Pts',(-1.05431200390781,-0.768424200550542,
1.54044293163017));
#19626=CARTESIAN_POINT('Ctrl Pts',(-1.26875982935484,-0.730457460039709,
1.74808806329354));
#19627=CARTESIAN_POINT('Ctrl Pts',(-1.49273481300659,-0.555328378424457,
1.91020772988088));
#19628=CARTESIAN_POINT('Ctrl Pts',(-0.762735325532963,-0.766529441696069,
1.28727233489076));
#19629=CARTESIAN_POINT('Ctrl Pts',(-0.777677426407099,-0.750680482155632,
1.28796759655004));
#19630=CARTESIAN_POINT('Ctrl Pts',(-0.792391461327318,-0.734615936171903,
1.2883190755065));
#19631=CARTESIAN_POINT('Ctrl Pts',(-0.806882581321256,-0.718338595112193,
1.288319084765));
#19632=CARTESIAN_POINT('Ctrl Pts',(-0.821284350360119,-0.70216161868754,
1.28831909396641));
#19633=CARTESIAN_POINT('Ctrl Pts',(-0.835451517519998,-0.685790724894018,
1.28797193184368));
#19634=CARTESIAN_POINT('Ctrl Pts',(-0.849391336665505,-0.669228599956957,
1.28727233489076));
#19635=CARTESIAN_POINT('Origin',(0.,0.,1.37171309575435));
#19636=CARTESIAN_POINT('',(-1.08521613661244,-0.642908916934714,1.10727038327973));
#19637=CARTESIAN_POINT('Ctrl Pts',(-1.81394816223928,-0.428377445609996,
1.63615580822897));
#19638=CARTESIAN_POINT('Ctrl Pts',(-1.75466459467969,-0.490704884304682,
1.59808263051822));
#19639=CARTESIAN_POINT('Ctrl Pts',(-1.68908545531116,-0.54441546832001,
1.55687869031203));
#19640=CARTESIAN_POINT('Ctrl Pts',(-1.52960471530763,-0.636822561166696,
1.4528510278119));
#19641=CARTESIAN_POINT('Ctrl Pts',(-1.43800725813254,-0.665855105856971,
1.3904370872311));
#19642=CARTESIAN_POINT('Ctrl Pts',(-1.2542115325179,-0.681216094986277,
1.25222975809873));
#19643=CARTESIAN_POINT('Ctrl Pts',(-1.16714103226326,-0.668566409010631,
1.18062438818012));
#19644=CARTESIAN_POINT('Ctrl Pts',(-1.08521613661244,-0.642908916934714,
1.10727038327973));
#19645=CARTESIAN_POINT('Origin',(0.,0.,1.10727038327973));
#19646=CARTESIAN_POINT('Ctrl Pts',(-1.01098164380599,-0.373486051296586,
1.28318517918604));
#19647=CARTESIAN_POINT('Ctrl Pts',(-1.23747555342208,-0.40602191942841,
1.537509268581));
#19648=CARTESIAN_POINT('Ctrl Pts',(-1.43047014156898,-0.30446532726343,
1.74606924121326));
#19649=CARTESIAN_POINT('Ctrl Pts',(-1.58996540824668,-0.0688162748016467,
1.90886509708284));
#19650=CARTESIAN_POINT('Ctrl Pts',(-1.02423814947078,-0.379996173302724,
1.26846828789983));
#19651=CARTESIAN_POINT('Ctrl Pts',(-1.25379621584498,-0.413260018127925,
1.51986220127974));
#19652=CARTESIAN_POINT('Ctrl Pts',(-1.4495127653333,-0.310691453231357,
1.72609931925976));
#19653=CARTESIAN_POINT('Ctrl Pts',(-1.61148865224617,-0.0719956513773679,
1.88702478432129));
#19654=CARTESIAN_POINT('Ctrl Pts',(-1.05021098685512,-0.388981181049685,
1.24114793592827));
#19655=CARTESIAN_POINT('Ctrl Pts',(-1.28554831174898,-0.422993564147046,
1.48712868773117));
#19656=CARTESIAN_POINT('Ctrl Pts',(-1.48619594640544,-0.317635541875723,
1.68884366634831));
#19657=CARTESIAN_POINT('Ctrl Pts',(-1.65214688300285,-0.0729037034540686,
1.84629652534568));
#19658=CARTESIAN_POINT('Ctrl Pts',(-1.11570416593891,-0.390726670926085,
1.18065052582665));
#19659=CARTESIAN_POINT('Ctrl Pts',(-1.36485769647198,-0.422167036078157,
1.41452066958594));
#19660=CARTESIAN_POINT('Ctrl Pts',(-1.57470193347746,-0.307195656373209,
1.60634085692189));
#19661=CARTESIAN_POINT('Ctrl Pts',(-1.74530108095234,-0.04566774902926,
1.75602521756878));
#19662=CARTESIAN_POINT('Ctrl Pts',(-1.1725125033894,-0.377231702026724,
1.13419834492991));
#19663=CARTESIAN_POINT('Ctrl Pts',(-1.43283860087532,-0.40328175100029,
1.35889748756925));
#19664=CARTESIAN_POINT('Ctrl Pts',(-1.64835039139676,-0.277966085037659,
1.54318426643096));
#19665=CARTESIAN_POINT('Ctrl Pts',(-1.81900536712132,-0.00100075866862149,
1.68700348817737));
#19666=CARTESIAN_POINT('Ctrl Pts',(-1.21448591285885,-0.362468171451202,
1.10179959977345));
#19667=CARTESIAN_POINT('Ctrl Pts',(-1.48279448162749,-0.383640993960513,
1.32012924726704));
#19668=CARTESIAN_POINT('Ctrl Pts',(-1.7017123916886,-0.249943984819037,
1.49916808705051));
#19669=CARTESIAN_POINT('Ctrl Pts',(-1.87123964304219,0.0386228559732266,
1.63891611912387));
#19670=CARTESIAN_POINT('',(-1.01462217612883,-0.373997862975653,1.28727233489076));
#19671=CARTESIAN_POINT('',(-1.20742290720348,-0.364905277844141,1.10727038327973));
#19672=CARTESIAN_POINT('Ctrl Pts',(-1.01462217612883,-0.373997862975653,
1.28727233489076));
#19673=CARTESIAN_POINT('Ctrl Pts',(-1.0440064014209,-0.388393237732341,
1.25472274024233));
#19674=CARTESIAN_POINT('Ctrl Pts',(-1.07127228109916,-0.391823670549174,
1.22803799031341));
#19675=CARTESIAN_POINT('Ctrl Pts',(-1.13395503796153,-0.386137988413888,
1.17079203987022));
#19676=CARTESIAN_POINT('Ctrl Pts',(-1.16846630960692,-0.378867340058898,
1.1405220316103));
#19677=CARTESIAN_POINT('Ctrl Pts',(-1.20742290720348,-0.364905277844141,
1.10727038327973));
#19678=CARTESIAN_POINT('Ctrl Pts',(-1.01462217612883,-0.373997862975653,
1.28727233489076));
#19679=CARTESIAN_POINT('Ctrl Pts',(-1.11493412912611,-0.387792676785358,
1.39987124007464));
#19680=CARTESIAN_POINT('Ctrl Pts',(-1.20865423507634,-0.375201374409042,
1.50346488650363));
#19681=CARTESIAN_POINT('Ctrl Pts',(-1.40394856048621,-0.287835131123856,
1.715480776583));
#19682=CARTESIAN_POINT('Ctrl Pts',(-1.50195515531182,-0.198779555753984,
1.81902921434248));
#19683=CARTESIAN_POINT('Ctrl Pts',(-1.58980227845634,-0.0690572297370878,
1.90869858745619));
#19684=CARTESIAN_POINT('Ctrl Pts',(-1.20742290720348,-0.364905277844141,
1.10727038327973));
#19685=CARTESIAN_POINT('Ctrl Pts',(-1.2881015973139,-0.372446289646659,
1.17697999301248));
#19686=CARTESIAN_POINT('Ctrl Pts',(-1.3704559615559,-0.364817298041905,
1.24430717677952));
#19687=CARTESIAN_POINT('Ctrl Pts',(-1.53992597283257,-0.308173273864792,
1.37795460947453));
#19688=CARTESIAN_POINT('Ctrl Pts',(-1.62124173855645,-0.257956459417358,
1.43952296396722));
#19689=CARTESIAN_POINT('Ctrl Pts',(-1.75990988600071,-0.127450637982168,
1.54779670475201));
#19690=CARTESIAN_POINT('Ctrl Pts',(-1.81609416413933,-0.0535283678677387,
1.59336495559369));
#19691=CARTESIAN_POINT('Ctrl Pts',(-1.86363850813291,0.0276890267571704,
1.63615580822897));
#19692=CARTESIAN_POINT('Ctrl Pts',(-1.08812850838495,-0.649602771712747,
1.10192461715937));
#19693=CARTESIAN_POINT('Ctrl Pts',(-1.34297974552473,-0.736092841324624,
1.32030517702043));
#19694=CARTESIAN_POINT('Ctrl Pts',(-1.58801866900221,-0.660305598163237,
1.49938098964776));
#19695=CARTESIAN_POINT('Ctrl Pts',(-1.82324527881738,-0.422241042228586,
1.63915205504133));
#19696=CARTESIAN_POINT('Ctrl Pts',(-1.07063084893098,-0.608736859462563,
1.13430265099724));
#19697=CARTESIAN_POINT('Ctrl Pts',(-1.32005612801352,-0.687616058553888,
1.35904945381843));
#19698=CARTESIAN_POINT('Ctrl Pts',(-1.55655247099159,-0.608897279480437,
1.54337045304296));
#19699=CARTESIAN_POINT('Ctrl Pts',(-1.78029541437304,-0.372779487140093,
1.68721036521565));
#19700=CARTESIAN_POINT('Ctrl Pts',(-1.04217626136028,-0.5578027141241,1.18072639205177));
#19701=CARTESIAN_POINT('Ctrl Pts',(-1.2834749683804,-0.627342551630417,
1.41463926643554));
#19702=CARTESIAN_POINT('Ctrl Pts',(-1.50849481334978,-0.546058002751383,
1.60649029622179));
#19703=CARTESIAN_POINT('Ctrl Pts',(-1.71737956252144,-0.313972100865309,
1.75619180366366));
#19704=CARTESIAN_POINT('Ctrl Pts',(-0.996637718803132,-0.510779237881579,
1.24117859886916));
#19705=CARTESIAN_POINT('Ctrl Pts',(-1.22630353645006,-0.572467001402757,
1.48719483570068));
#19706=CARTESIAN_POINT('Ctrl Pts',(-1.43804667102143,-0.491616133252193,
1.68893408523069));
#19707=CARTESIAN_POINT('Ctrl Pts',(-1.63186740528248,-0.26823580862317,
1.84639893874704));
#19708=CARTESIAN_POINT('Ctrl Pts',(-0.972472692862429,-0.497730252266281,
1.26847955290007));
#19709=CARTESIAN_POINT('Ctrl Pts',(-1.1965424430155,-0.55780480775003,1.51990601315848));
#19710=CARTESIAN_POINT('Ctrl Pts',(-1.40293468429945,-0.478797895551023,
1.72616419407532));
#19711=CARTESIAN_POINT('Ctrl Pts',(-1.59191672260126,-0.260780594211966,
1.88709951781477));
#19712=CARTESIAN_POINT('Ctrl Pts',(-0.958722904028868,-0.49236880332188,
1.28318566992362));
#19713=CARTESIAN_POINT('Ctrl Pts',(-1.17968618624264,-0.551916626543442,
1.53754047574671));
#19714=CARTESIAN_POINT('Ctrl Pts',(-1.38351688474614,-0.474283127502362,
1.74612008846831));
#19715=CARTESIAN_POINT('Ctrl Pts',(-1.57021499953936,-0.259468306198639,
1.90892450808845));
#19716=CARTESIAN_POINT('',(-0.962275025729455,-0.493314642657339,1.28727233489076));
#19717=CARTESIAN_POINT('Ctrl Pts',(-1.08521613661244,-0.642908916934714,
1.10727038327973));
#19718=CARTESIAN_POINT('Ctrl Pts',(-1.0754332329569,-0.618651911001871,
1.12805083925446));
#19719=CARTESIAN_POINT('Ctrl Pts',(-1.06308333609212,-0.593211674629724,
1.15131250789253));
#19720=CARTESIAN_POINT('Ctrl Pts',(-1.03791374180393,-0.554422984205748,
1.19194777349594));
#19721=CARTESIAN_POINT('Ctrl Pts',(-1.02533374006937,-0.537242802810029,
1.21108489280015));
#19722=CARTESIAN_POINT('Ctrl Pts',(-0.999433395982659,-0.512927734894534,
1.245266066507));
#19723=CARTESIAN_POINT('Ctrl Pts',(-0.98452570391201,-0.501969908730666,
1.26352342884102));
#19724=CARTESIAN_POINT('Ctrl Pts',(-0.962275025729455,-0.493314642657339,
1.28727233489076));
#19725=CARTESIAN_POINT('Ctrl Pts',(-0.962275025729455,-0.493314642657339,
1.28727233489076));
#19726=CARTESIAN_POINT('Ctrl Pts',(-1.06019965524839,-0.519074140629024,
1.39987124007464));
#19727=CARTESIAN_POINT('Ctrl Pts',(-1.15475382712427,-0.517846241724568,
1.50346488650363));
#19728=CARTESIAN_POINT('Ctrl Pts',(-1.35913828497575,-0.454602843714802,
1.715480776583));
#19729=CARTESIAN_POINT('Ctrl Pts',(-1.46714441944577,-0.377981286365636,
1.81902921434248));
#19730=CARTESIAN_POINT('Ctrl Pts',(-1.5699559447672,-0.259766273896473,
1.90869858745619));
#19731=CARTESIAN_POINT('Ctrl Pts',(-0.962275025729455,-0.493314642657339,
1.28727233489076));
#19732=CARTESIAN_POINT('Ctrl Pts',(-1.18245156164078,-0.551233034159898,
1.54044293163017));
#19733=CARTESIAN_POINT('Ctrl Pts',(-1.38558898119851,-0.472718500477254,
1.74808806329354));
#19734=CARTESIAN_POINT('Ctrl Pts',(-1.57168728440264,-0.257771041609407,
1.91020772988088));
#19735=CARTESIAN_POINT('Ctrl Pts',(-0.979724075862581,-0.453542382763444,
1.28727233489076));
#19736=CARTESIAN_POINT('Ctrl Pts',(-1.20168985388846,-0.502493528317088,
1.54044293163017));
#19737=CARTESIAN_POINT('Ctrl Pts',(-1.4011880115129,-0.416024993050259,
1.74808806329354));
#19738=CARTESIAN_POINT('Ctrl Pts',(-1.57821854873589,-0.194136776962957,
1.91020772988088));
#19739=CARTESIAN_POINT('Ctrl Pts',(-0.997173125995706,-0.413770122869549,
1.28727233489076));
#19740=CARTESIAN_POINT('Ctrl Pts',(-1.22092814613614,-0.453754022474278,
1.54044293163017));
#19741=CARTESIAN_POINT('Ctrl Pts',(-1.41678704182728,-0.359331485623264,
1.74808806329354));
#19742=CARTESIAN_POINT('Ctrl Pts',(-1.58474981306913,-0.130502512316506,
1.91020772988088));
#19743=CARTESIAN_POINT('Ctrl Pts',(-1.01462217612883,-0.373997862975653,
1.28727233489076));
#19744=CARTESIAN_POINT('Ctrl Pts',(-1.24016643838382,-0.405014516631467,
1.54044293163017));
#19745=CARTESIAN_POINT('Ctrl Pts',(-1.43238607214167,-0.302637978196268,
1.74808806329354));
#19746=CARTESIAN_POINT('Ctrl Pts',(-1.59128107740238,-0.0668682476700562,
1.91020772988088));
#19747=CARTESIAN_POINT('Ctrl Pts',(-0.962275025729455,-0.493314642657339,
1.28727233489076));
#19748=CARTESIAN_POINT('Ctrl Pts',(-0.971588210291795,-0.473624023308118,
1.28796759655004));
#19749=CARTESIAN_POINT('Ctrl Pts',(-0.980617871367769,-0.453798845322803,
1.2883190755065));
#19750=CARTESIAN_POINT('Ctrl Pts',(-0.989369770455727,-0.433840171694363,
1.288319084765));
#19751=CARTESIAN_POINT('Ctrl Pts',(-0.998067706113495,-0.414004561469673,
1.28831909396641));
#19752=CARTESIAN_POINT('Ctrl Pts',(-1.00648259836303,-0.394057020835215,
1.28797193184368));
#19753=CARTESIAN_POINT('Ctrl Pts',(-1.01462217612883,-0.373997862975653,
1.28727233489076));
#19754=CARTESIAN_POINT('Origin',(0.,0.,1.37171309575435));
#19755=CARTESIAN_POINT('',(-1.23077165948193,-0.27609248605185,1.10727038327973));
#19756=CARTESIAN_POINT('Ctrl Pts',(-1.85754313061971,0.153129647965883,
1.63615580822897));
#19757=CARTESIAN_POINT('Ctrl Pts',(-1.81335940151627,0.0607713534907818,
1.59083969670469));
#19758=CARTESIAN_POINT('Ctrl Pts',(-1.75708539039456,-0.0223614442500404,
1.54129005514746));
#19759=CARTESIAN_POINT('Ctrl Pts',(-1.61733286423933,-0.159600739735627,
1.42521036359321));
#19760=CARTESIAN_POINT('Ctrl Pts',(-1.53789592166465,-0.208550308549111,
1.36183966503053));
#19761=CARTESIAN_POINT('Ctrl Pts',(-1.37907079095174,-0.264206681902337,
1.23219371736399));
#19762=CARTESIAN_POINT('Ctrl Pts',(-1.30454791379682,-0.275306576910198,
1.17031259812848));
#19763=CARTESIAN_POINT('Ctrl Pts',(-1.23077165948193,-0.27609248605185,
1.10727038327973));
#19764=CARTESIAN_POINT('Origin',(0.,0.,1.10727038327973));
#19765=CARTESIAN_POINT('Ctrl Pts',(-1.07691421720911,-0.042795833893793,
1.28318517918604));
#19766=CARTESIAN_POINT('Ctrl Pts',(-1.30237686203014,-0.00374881610008784,
1.537509268581));
#19767=CARTESIAN_POINT('Ctrl Pts',(-1.45454290982716,0.152475850210932,
1.74606924121326));
#19768=CARTESIAN_POINT('Ctrl Pts',(-1.53341236060018,0.425878165039266,
1.90886509708284));
#19769=CARTESIAN_POINT('Ctrl Pts',(-1.091545040475,-0.0448924758011831,
1.26845681306972));
#19770=CARTESIAN_POINT('Ctrl Pts',(-1.32014932750452,-0.00559080476410112,
1.51984840181958));
#19771=CARTESIAN_POINT('Ctrl Pts',(-1.4745930125769,0.152438895007655,1.72608377212012));
#19772=CARTESIAN_POINT('Ctrl Pts',(-1.55488138991364,0.429508274607612,
1.88700775532559));
#19773=CARTESIAN_POINT('Ctrl Pts',(-1.11904054473513,-0.0454099470705951,
1.24111941924412));
#19774=CARTESIAN_POINT('Ctrl Pts',(-1.35337649424567,-0.00503268467650647,
1.48709402322589));
#19775=CARTESIAN_POINT('Ctrl Pts',(-1.51165038249935,0.15717562594847,1.68880469124906));
#19776=CARTESIAN_POINT('Ctrl Pts',(-1.59385438982847,0.441219201568136,
1.84625359892919));
#19777=CARTESIAN_POINT('Ctrl Pts',(-1.18191630764682,-0.0267999250011405,
1.1805768626608));
#19778=CARTESIAN_POINT('Ctrl Pts',(-1.42860644524989,0.0203022432084532,
1.41443159040039));
#19779=CARTESIAN_POINT('Ctrl Pts',(-1.59265822923791,0.194505783955957,
1.60624053738541));
#19780=CARTESIAN_POINT('Ctrl Pts',(-1.67408715628731,0.495974904441976,
1.7559150245411));
#19781=CARTESIAN_POINT('Ctrl Pts',(-1.23181557314521,0.0036323801669868,
1.1340877844534));
#19782=CARTESIAN_POINT('Ctrl Pts',(-1.48747160844964,0.059323221268054,
1.35876508657128));
#19783=CARTESIAN_POINT('Ctrl Pts',(-1.65371551508435,0.245130498049616,
1.54303391436826));
#19784=CARTESIAN_POINT('Ctrl Pts',(-1.73041945202573,0.561310568731046,
1.68683916414419));
#19785=CARTESIAN_POINT('Ctrl Pts',(-1.26719829440569,0.0306796703371001,
1.101666983688));
#19786=CARTESIAN_POINT('Ctrl Pts',(-1.52894260490194,0.0934843164788996,
1.31997051162989));
#19787=CARTESIAN_POINT('Ctrl Pts',(-1.69583409006838,0.288323673548526,
1.4989879457606));
#19788=CARTESIAN_POINT('Ctrl Pts',(-1.76787274990502,0.615197741545978,
1.63871928608013));
#19789=CARTESIAN_POINT('',(-1.08053472770428,-0.0421576093699569,1.28727233489076));
#19790=CARTESIAN_POINT('',(-1.22409607968053,1.1943445105165E-9,1.144533070421));
#19791=CARTESIAN_POINT('Ctrl Pts',(-1.08053472770428,-0.0421576093699569,
1.28727233489076));
#19792=CARTESIAN_POINT('Ctrl Pts',(-1.11292920208489,-0.0467681993550381,
1.25472274024224));
#19793=CARTESIAN_POINT('Ctrl Pts',(-1.13992065666394,-0.0416051146519816,
1.22803799031326));
#19794=CARTESIAN_POINT('Ctrl Pts',(-1.18752803009125,-0.0212174145555454,
1.18093412618539));
#19795=CARTESIAN_POINT('Ctrl Pts',(-1.20526565550415,-0.0119731083046825,
1.16336349462073));
#19796=CARTESIAN_POINT('Ctrl Pts',(-1.22409607968053,2.38868920650337E-9,
1.144533070421));
#19797=CARTESIAN_POINT('Ctrl Pts',(-1.08053472770428,-0.0421576093699569,
1.28727233489076));
#19798=CARTESIAN_POINT('Ctrl Pts',(-1.18019989616608,-0.0242791587196548,
1.39987124007464));
#19799=CARTESIAN_POINT('Ctrl Pts',(-1.26544208722232,0.0166569869072258,
1.50346488650363));
#19800=CARTESIAN_POINT('Ctrl Pts',(-1.42418037408903,0.160096487344471,
1.715480776583));
#19801=CARTESIAN_POINT('Ctrl Pts',(-1.48987049850469,0.275079075974333,
1.81902921434248));
#19802=CARTESIAN_POINT('Ctrl Pts',(-1.53333167412,0.425598593400271,1.90869858745619));
#19803=CARTESIAN_POINT('',(-1.26108935601086,0.0260686553993156,1.10727038327973));
#19804=CARTESIAN_POINT('Ctrl Pts',(-1.26108935601086,0.0260686553993152,
1.10727038327973));
#19805=CARTESIAN_POINT('Ctrl Pts',(-1.34014965076829,0.0438278133131024,
1.17697999301248));
#19806=CARTESIAN_POINT('Ctrl Pts',(-1.41611581747019,0.0765323136032917,
1.24430717677953));
#19807=CARTESIAN_POINT('Ctrl Pts',(-1.55978740991096,0.182773095427525,
1.37795460947454));
#19808=CARTESIAN_POINT('Ctrl Pts',(-1.62160544971256,0.255660077554636,
1.43952296396723));
#19809=CARTESIAN_POINT('Ctrl Pts',(-1.71055550747296,0.417882684528441,
1.54471868724288));
#19810=CARTESIAN_POINT('Ctrl Pts',(-1.74236185427976,0.503955443296111,
1.59041399531273));
#19811=CARTESIAN_POINT('Ctrl Pts',(-1.76386916735271,0.602229799711921,
1.63615580822897));
#19812=CARTESIAN_POINT('Ctrl Pts',(-1.22409607968053,2.38868920650337E-9,
1.144533070421));
#19813=CARTESIAN_POINT('Ctrl Pts',(-1.23602443718504,0.00758451261819888,
1.13260471290168));
#19814=CARTESIAN_POINT('Ctrl Pts',(-1.24839445491079,0.0162506540138241,
1.12016548273562));
#19815=CARTESIAN_POINT('Ctrl Pts',(-1.26108935601086,0.0260686553993153,
1.10727038327973));
#19816=CARTESIAN_POINT('Ctrl Pts',(-1.23578335387376,-0.281756991007075,
1.1017328493151));
#19817=CARTESIAN_POINT('Ctrl Pts',(-1.50493278576872,-0.285293785520307,
1.32007563441911));
#19818=CARTESIAN_POINT('Ctrl Pts',(-1.71461214828354,-0.137495264840182,
1.49912049044759));
#19819=CARTESIAN_POINT('Ctrl Pts',(-1.8648214414182,0.1616385710333,1.63886741740055));
#19820=CARTESIAN_POINT('Ctrl Pts',(-1.21381148288727,-0.256619313744399,
1.12604029619216));
#19821=CARTESIAN_POINT('Ctrl Pts',(-1.47730375097777,-0.255919204048238,
1.34917212439386));
#19822=CARTESIAN_POINT('Ctrl Pts',(-1.68029140190123,-0.108074844008926,
1.53213933043029));
#19823=CARTESIAN_POINT('Ctrl Pts',(-1.82267525691205,0.187017052056837,
1.67494641070563));
#19824=CARTESIAN_POINT('Ctrl Pts',(-1.17543855297398,-0.219711749650113,
1.16779612397806));
#19825=CARTESIAN_POINT('Ctrl Pts',(-1.42937433465483,-0.213070651520421,
1.39915507862237));
#19826=CARTESIAN_POINT('Ctrl Pts',(-1.62159457256361,-0.0660178837300448,
1.58891631513415));
#19827=CARTESIAN_POINT('Ctrl Pts',(-1.75213954537449,0.221600535375864,
1.73698522631427));
#19828=CARTESIAN_POINT('Ctrl Pts',(-1.11847368101377,-0.181934739915363,
1.22808906223352));
#19829=CARTESIAN_POINT('Ctrl Pts',(-1.35883455739468,-0.169938151077974,
1.47147297599238));
#19830=CARTESIAN_POINT('Ctrl Pts',(-1.53761229859012,-0.0262526925971351,
1.67105384595181));
#19831=CARTESIAN_POINT('Ctrl Pts',(-1.65481713073797,0.249117593166617,
1.82682748557708));
#19832=CARTESIAN_POINT('Ctrl Pts',(-1.08361696356336,-0.173143664137204,
1.26355539141207));
#19833=CARTESIAN_POINT('Ctrl Pts',(-1.31631931390947,-0.160806376565823,
1.51400180025811));
#19834=CARTESIAN_POINT('Ctrl Pts',(-1.48896648444242,-0.0212938283898121,
1.71948206324578));
#19835=CARTESIAN_POINT('Ctrl Pts',(-1.6016350942056,0.245739828560955,1.87979168962263));
#19836=CARTESIAN_POINT('Ctrl Pts',(-1.06394999292458,-0.172008888578299,
1.28318566992362));
#19837=CARTESIAN_POINT('Ctrl Pts',(-1.29249985168945,-0.160360824547434,
1.5375404757467));
#19838=CARTESIAN_POINT('Ctrl Pts',(-1.46236429518571,-0.0235398295887255,
1.74612008846831));
#19839=CARTESIAN_POINT('Ctrl Pts',(-1.57354332341336,0.238454096297827,
1.90892450808844));
#19840=CARTESIAN_POINT('',(-1.06762054184321,-0.171810769270086,1.28727233489076));
#19841=CARTESIAN_POINT('Ctrl Pts',(-1.23077165948193,-0.27609248605185,
1.10727038327973));
#19842=CARTESIAN_POINT('Ctrl Pts',(-1.21397173814619,-0.256045785977561,
1.1280508392544));
#19843=CARTESIAN_POINT('Ctrl Pts',(-1.19436482287745,-0.235667011409717,
1.15131250789248));
#19844=CARTESIAN_POINT('Ctrl Pts',(-1.15844075168685,-0.206554607000212,
1.19194777349561));
#19845=CARTESIAN_POINT('Ctrl Pts',(-1.14116749104443,-0.19410271785781,
1.21108489279989));
#19846=CARTESIAN_POINT('Ctrl Pts',(-1.10902103082118,-0.178981360555552,
1.24526606650677));
#19847=CARTESIAN_POINT('Ctrl Pts',(-1.09145681862839,-0.173166578774625,
1.26352342884084));
#19848=CARTESIAN_POINT('Ctrl Pts',(-1.06762054184321,-0.171810769270086,
1.28727233489076));
#19849=CARTESIAN_POINT('Ctrl Pts',(-1.06762054184321,-0.171810769270086,
1.28727233489076));
#19850=CARTESIAN_POINT('Ctrl Pts',(-1.16871252149279,-0.166049132983329,
1.39987124007464));
#19851=CARTESIAN_POINT('Ctrl Pts',(-1.25825944116939,-0.135662485730195,
1.50346488650363));
#19852=CARTESIAN_POINT('Ctrl Pts',(-1.43309732687145,-0.0123561690781437,
1.715480776583));
#19853=CARTESIAN_POINT('Ctrl Pts',(-1.51213990150266,0.0938909933754472,
1.81902921434248));
#19854=CARTESIAN_POINT('Ctrl Pts',(-1.57338902476662,0.238090659850088,
1.90869858745619));
#19855=CARTESIAN_POINT('Ctrl Pts',(-1.06762054184321,-0.171810769270086,
1.28727233489076));
#19856=CARTESIAN_POINT('Ctrl Pts',(-1.29491863831812,-0.158856141562724,
1.54044293163017));
#19857=CARTESIAN_POINT('Ctrl Pts',(-1.46385147967852,-0.0214114678431581,
1.74808806329354));
#19858=CARTESIAN_POINT('Ctrl Pts',(-1.5744190659244,0.240523251888612,1.91020772988088));
#19859=CARTESIAN_POINT('Ctrl Pts',(-1.07192527046357,-0.128593049303376,
1.28727233489076));
#19860=CARTESIAN_POINT('Ctrl Pts',(-1.2981540059198,-0.106557157682628,
1.54044293163017));
#19861=CARTESIAN_POINT('Ctrl Pts',(-1.46116778184124,0.0373276272898291,
1.74808806329354));
#19862=CARTESIAN_POINT('Ctrl Pts',(-1.56096659822788,0.303061305613997,
1.91020772988088));
#19863=CARTESIAN_POINT('Ctrl Pts',(-1.07622999908393,-0.0853753293366666,
1.28727233489076));
#19864=CARTESIAN_POINT('Ctrl Pts',(-1.30138937352148,-0.0542581738025321,
1.54044293163017));
#19865=CARTESIAN_POINT('Ctrl Pts',(-1.45848408400396,0.0960667224228176,
1.74808806329354));
#19866=CARTESIAN_POINT('Ctrl Pts',(-1.54751413053135,0.365599359339382,
1.91020772988088));
#19867=CARTESIAN_POINT('Ctrl Pts',(-1.08053472770428,-0.0421576093699569,
1.28727233489076));
#19868=CARTESIAN_POINT('Ctrl Pts',(-1.30462474112317,-0.00195918992243616,
1.54044293163017));
#19869=CARTESIAN_POINT('Ctrl Pts',(-1.45580038616668,0.154805817555805,
1.74808806329354));
#19870=CARTESIAN_POINT('Ctrl Pts',(-1.53406166283483,0.428137413064766,
1.91020772988088));
#19871=CARTESIAN_POINT('Ctrl Pts',(-1.06762054184321,-0.171810769270086,
1.28727233489076));
#19872=CARTESIAN_POINT('Ctrl Pts',(-1.0703931707,-0.150205945126616,1.28796759655004));
#19873=CARTESIAN_POINT('Ctrl Pts',(-1.07285457179227,-0.128560761691046,
1.2883190755065));
#19874=CARTESIAN_POINT('Ctrl Pts',(-1.07501055311346,-0.106874449528872,
1.288319084765));
#19875=CARTESIAN_POINT('Ctrl Pts',(-1.07715324084587,-0.0853218532357573,
1.28831909396641));
#19876=CARTESIAN_POINT('Ctrl Pts',(-1.07899214990169,-0.0637502700203498,
1.28797193184368));
#19877=CARTESIAN_POINT('Ctrl Pts',(-1.08053472770428,-0.0421576093699569,
1.28727233489076));
#19878=CARTESIAN_POINT('Origin',(0.,0.,1.37171309575435));
#19879=CARTESIAN_POINT('',(-1.25585067703094,0.117749801015232,1.10727038327973));
#19880=CARTESIAN_POINT('Ctrl Pts',(-1.71930883511106,0.719647344681869,
1.63615580822897));
#19881=CARTESIAN_POINT('Ctrl Pts',(-1.70798257074607,0.63437738084719,1.59808263051822));
#19882=CARTESIAN_POINT('Ctrl Pts',(-1.68649822169668,0.552378154622133,
1.55687869031203));
#19883=CARTESIAN_POINT('Ctrl Pts',(-1.61179111914083,0.383878819109613,
1.4528510278119));
#19884=CARTESIAN_POINT('Ctrl Pts',(-1.55475212125011,0.306551362590219,
1.3904370872311));
#19885=CARTESIAN_POINT('Ctrl Pts',(-1.41508721860523,0.186091644383524,
1.25222975809873));
#19886=CARTESIAN_POINT('Ctrl Pts',(-1.33721040532788,0.145146699351923,
1.18062438818012));
#19887=CARTESIAN_POINT('Ctrl Pts',(-1.25585067703094,0.117749801015232,
1.10727038327973));
#19888=CARTESIAN_POINT('Origin',(0.,0.,1.10727038327973));
#19889=CARTESIAN_POINT('Ctrl Pts',(-1.03743092372925,0.292083537906633,
1.28318517918604));
#19890=CARTESIAN_POINT('Ctrl Pts',(-1.23979244918951,0.39889124746765,1.537509268581));
#19891=CARTESIAN_POINT('Ctrl Pts',(-1.33623488367509,0.594491629104934,
1.74606924121327));
#19892=CARTESIAN_POINT('Ctrl Pts',(-1.32675822718598,0.878884682818485,
1.90886509708284));
#19893=CARTESIAN_POINT('Ctrl Pts',(-1.05199356151554,0.294610685989129,
1.26845681306972));
#19894=CARTESIAN_POINT('Ctrl Pts',(-1.25726427409018,0.402631406009325,
1.51984840181958));
#19895=CARTESIAN_POINT('Ctrl Pts',(-1.35531508433346,0.600652305106679,
1.72608377212012));
#19896=CARTESIAN_POINT('Ctrl Pts',(-1.34605472186502,0.88897141708892,1.88700775532559));
#19897=CARTESIAN_POINT('Ctrl Pts',(-1.07830248703538,0.302614092509142,
1.241120378339));
#19898=CARTESIAN_POINT('Ctrl Pts',(-1.28869195855349,0.413428941810946,
1.48709498232078));
#19899=CARTESIAN_POINT('Ctrl Pts',(-1.38909450341186,0.616606838701708,
1.68880599613843));
#19900=CARTESIAN_POINT('Ctrl Pts',(-1.3795008682383,0.912150767476994,1.84625490381856));
#19901=CARTESIAN_POINT('Ctrl Pts',(-1.13234954650475,0.339741650892322,
1.18057861631984));
#19902=CARTESIAN_POINT('Ctrl Pts',(-1.35241043892922,0.460769919763727,
1.41443334405943));
#19903=CARTESIAN_POINT('Ctrl Pts',(-1.4546018215964,0.67714071293772,1.6062429176887));
#19904=CARTESIAN_POINT('Ctrl Pts',(-1.4388862517722,0.989017806729704,1.7559174048444));
#19905=CARTESIAN_POINT('Ctrl Pts',(-1.17040376051197,0.384106544865058,
1.1340877844534));
#19906=CARTESIAN_POINT('Ctrl Pts',(-1.39633768248717,0.516073741815779,
1.35876508657128));
#19907=CARTESIAN_POINT('Ctrl Pts',(-1.49702742698245,0.744159155535353,
1.54303391436826));
#19908=CARTESIAN_POINT('Ctrl Pts',(-1.4722721909128,1.06856709212994,1.68683916414419));
#19909=CARTESIAN_POINT('Ctrl Pts',(-1.19569665581665,0.420763908606192,
1.101666983688));
#19910=CARTESIAN_POINT('Ctrl Pts',(-1.42522258493377,0.561378116697256,
1.31997051162989));
#19911=CARTESIAN_POINT('Ctrl Pts',(-1.52373714690789,0.798253662001989,
1.49898794576061));
#19912=CARTESIAN_POINT('Ctrl Pts',(-1.491240341739,1.13139054452039,1.63871928608014));
#19913=CARTESIAN_POINT('',(-1.04067701160391,0.293809324770207,1.28727233489076));
#19914=CARTESIAN_POINT('',(-1.19131159212569,0.414490807021284,1.10727038327973));
#19915=CARTESIAN_POINT('Ctrl Pts',(-1.04067701160391,0.293809324770207,
1.28727233489076));
#19916=CARTESIAN_POINT('Ctrl Pts',(-1.07291073821508,0.299434836228392,
1.25472274024218));
#19917=CARTESIAN_POINT('Ctrl Pts',(-1.0969856560603,0.312686039747429,1.22803799031299));
#19918=CARTESIAN_POINT('Ctrl Pts',(-1.14435511150582,0.354129853274474,
1.17079203987229));
#19919=CARTESIAN_POINT('Ctrl Pts',(-1.16800173688696,0.380297147864045,
1.14052203161246));
#19920=CARTESIAN_POINT('Ctrl Pts',(-1.19131159212569,0.414490807021284,
1.10727038327973));
#19921=CARTESIAN_POINT('Ctrl Pts',(-1.04067701160391,0.293809324770207,
1.28727233489076));
#19922=CARTESIAN_POINT('Ctrl Pts',(-1.12993947443311,0.341610972564374,
1.39987124007464));
#19923=CARTESIAN_POINT('Ctrl Pts',(-1.19835965101752,0.406884846288962,
1.50346488650363));
#19924=CARTESIAN_POINT('Ctrl Pts',(-1.30500348982786,0.592356746173702,
1.715480776583));
#19925=CARTESIAN_POINT('Ctrl Pts',(-1.33194693676576,0.722011051157661,
1.81902921434248));
#19926=CARTESIAN_POINT('Ctrl Pts',(-1.32676788217082,0.878593860895847,
1.90869858745619));
#19927=CARTESIAN_POINT('Ctrl Pts',(-1.19131159212569,0.414490807021284,
1.10727038327973));
#19928=CARTESIAN_POINT('Ctrl Pts',(-1.26101451903382,0.455811744539446,
1.17697999301248));
#19929=CARTESIAN_POINT('Ctrl Pts',(-1.32315639051141,0.510390409161015,
1.24430717677953));
#19930=CARTESIAN_POINT('Ctrl Pts',(-1.42696598762934,0.655828360684352,
1.37795460947454));
#19931=CARTESIAN_POINT('Ctrl Pts',(-1.46323512106126,0.744250824847066,
1.43952296396723));
#19932=CARTESIAN_POINT('Ctrl Pts',(-1.49770211069242,0.92602077179853,1.54471868724291));
#19933=CARTESIAN_POINT('Ctrl Pts',(-1.50135379887061,1.01770953159232,1.59041399531275));
#19934=CARTESIAN_POINT('Ctrl Pts',(-1.4914400228729,1.11782012388912,1.63615580822897));
#19935=CARTESIAN_POINT('Ctrl Pts',(-1.26214138440836,0.114046207919,1.10192461715937));
#19936=CARTESIAN_POINT('Ctrl Pts',(-1.51915795367952,0.193872070477571,
1.32030517702043));
#19937=CARTESIAN_POINT('Ctrl Pts',(-1.67285198321398,0.399215503609641,
1.49938098964775));
#19938=CARTESIAN_POINT('Ctrl Pts',(-1.72322347301172,0.730076507315209,
1.63915205504133));
#19939=CARTESIAN_POINT('Ctrl Pts',(-1.23350917110671,0.131128471412263,
1.12620814253777));
#19940=CARTESIAN_POINT('Ctrl Pts',(-1.48384440470434,0.213229856531406,
1.3493730700966));
#19941=CARTESIAN_POINT('Ctrl Pts',(-1.63116936194582,0.416549152036913,
1.53236753871639));
#19942=CARTESIAN_POINT('Ctrl Pts',(-1.67535851585319,0.741153963610053,
1.67519578767207));
#19943=CARTESIAN_POINT('Ctrl Pts',(-1.18566161414104,0.154321672329431,
1.16792358645355));
#19944=CARTESIAN_POINT('Ctrl Pts',(-1.42508536822678,0.239112514228605,
1.39930746388998));
#19945=CARTESIAN_POINT('Ctrl Pts',(-1.56242925297241,0.438352145622171,
1.58908978141842));
#19946=CARTESIAN_POINT('Ctrl Pts',(-1.59768412386215,0.752201465653604,
1.73717464481022));
#19947=CARTESIAN_POINT('Ctrl Pts',(-1.11989042845004,0.172598846101516,
1.2281493040678));
#19948=CARTESIAN_POINT('Ctrl Pts',(-1.34476711329973,0.258281860114562,
1.47154499595952));
#19949=CARTESIAN_POINT('Ctrl Pts',(-1.47038505632135,0.450170312236593,
1.67113613169255));
#19950=CARTESIAN_POINT('Ctrl Pts',(-1.49675459841166,0.748265815679372,
1.82691733765971));
#19951=CARTESIAN_POINT('Ctrl Pts',(-1.08406383481182,0.17018101435307,1.26357751389222));
#19952=CARTESIAN_POINT('Ctrl Pts',(-1.30156053800083,0.253820963688729,
1.51402822523202));
#19953=CARTESIAN_POINT('Ctrl Pts',(-1.42264323155934,0.439852505027486,
1.71951214242024));
#19954=CARTESIAN_POINT('Ctrl Pts',(-1.44728013834437,0.72862733638904,1.87982452105688));
#19955=CARTESIAN_POINT('Ctrl Pts',(-1.06503024353735,0.165188454635723,
1.28318566992362));
#19956=CARTESIAN_POINT('Ctrl Pts',(-1.27879462627691,0.246892212254839,
1.5375404757467));
#19957=CARTESIAN_POINT('Ctrl Pts',(-1.39806529952135,0.429507710856691,
1.74612008846831));
#19958=CARTESIAN_POINT('Ctrl Pts',(-1.42284226327066,0.713034950441279,
1.90892450808844));
#19959=CARTESIAN_POINT('',(-1.06845992077163,0.166511139289342,1.28727233489076));
#19960=CARTESIAN_POINT('Ctrl Pts',(-1.25585067703094,0.117749801015232,
1.10727038327973));
#19961=CARTESIAN_POINT('Ctrl Pts',(-1.23367823136702,0.13162388455433,1.12805083925461));
#19962=CARTESIAN_POINT('Ctrl Pts',(-1.20873355917026,0.144946380875815,
1.15131250789267));
#19963=CARTESIAN_POINT('Ctrl Pts',(-1.16557150946219,0.161532774289756,
1.1919477734965));
#19964=CARTESIAN_POINT('Ctrl Pts',(-1.1452958170136,0.168037493511785,1.21108489280069));
#19965=CARTESIAN_POINT('Ctrl Pts',(-1.11004996015928,0.172484956391182,
1.24526606650637));
#19966=CARTESIAN_POINT('Ctrl Pts',(-1.0915485353108,0.172587502434539,1.26352342884047));
#19967=CARTESIAN_POINT('Ctrl Pts',(-1.06845992077163,0.166511139289342,
1.28727233489076));
#19968=CARTESIAN_POINT('Ctrl Pts',(-1.06845992077163,0.166511139289342,
1.28727233489076));
#19969=CARTESIAN_POINT('Ctrl Pts',(-1.16282366323453,0.203229920731113,
1.39987124007464));
#19970=CARTESIAN_POINT('Ctrl Pts',(-1.23859785430383,0.259800859583567,
1.50346488650363));
#19971=CARTESIAN_POINT('Ctrl Pts',(-1.36677481743678,0.431100013478375,
1.715480776583));
#19972=CARTESIAN_POINT('Ctrl Pts',(-1.40911659430225,0.556572568507924,
1.81902921434248));
#19973=CARTESIAN_POINT('Ctrl Pts',(-1.42280782457595,0.712641620935351,
1.90869858745619));
#19974=CARTESIAN_POINT('Ctrl Pts',(-1.06845992077163,0.166511139289342,
1.28727233489076));
#19975=CARTESIAN_POINT('Ctrl Pts',(-1.28063005644821,0.24907069698643,1.54044293163017));
#19976=CARTESIAN_POINT('Ctrl Pts',(-1.3988219960746,0.431991468445894,1.74808806329354));
#19977=CARTESIAN_POINT('Ctrl Pts',(-1.42303573965083,0.715273453667736,
1.91020772988088));
#19978=CARTESIAN_POINT('Ctrl Pts',(-1.05919895104906,0.208943867782964,
1.28727233489076));
#19979=CARTESIAN_POINT('Ctrl Pts',(-1.26754579908091,0.29980976997318,1.54044293163017));
#19980=CARTESIAN_POINT('Ctrl Pts',(-1.37811826912839,0.487026359393917,
1.74808806329354));
#19981=CARTESIAN_POINT('Ctrl Pts',(-1.39091636119152,0.770593636045173,
1.91020772988088));
#19982=CARTESIAN_POINT('Ctrl Pts',(-1.04993798132648,0.251376596276585,
1.28727233489076));
#19983=CARTESIAN_POINT('Ctrl Pts',(-1.25446154171361,0.350548842959931,
1.54044293163017));
#19984=CARTESIAN_POINT('Ctrl Pts',(-1.35741454218218,0.542061250341939,
1.74808806329354));
#19985=CARTESIAN_POINT('Ctrl Pts',(-1.35879698273221,0.825913818422611,
1.91020772988088));
#19986=CARTESIAN_POINT('Ctrl Pts',(-1.04067701160391,0.293809324770207,
1.28727233489076));
#19987=CARTESIAN_POINT('Ctrl Pts',(-1.24137728434631,0.401287915946682,
1.54044293163017));
#19988=CARTESIAN_POINT('Ctrl Pts',(-1.33671081523597,0.597096141289962,
1.74808806329354));
#19989=CARTESIAN_POINT('Ctrl Pts',(-1.3266776042729,0.881234000800048,1.91020772988088));
#19990=CARTESIAN_POINT('Ctrl Pts',(-1.06845992077163,0.166511139289342,
1.28727233489076));
#19991=CARTESIAN_POINT('Ctrl Pts',(-1.06442058969234,0.187915337510244,
1.28796759655004));
#19992=CARTESIAN_POINT('Ctrl Pts',(-1.06007279171241,0.209261745030532,
1.2883190755065));
#19993=CARTESIAN_POINT('Ctrl Pts',(-1.05542181279351,0.230552888394581,
1.288319084765));
#19994=CARTESIAN_POINT('Ctrl Pts',(-1.05079951139632,0.251712752465176,
1.28831909396641));
#19995=CARTESIAN_POINT('Ctrl Pts',(-1.0458824320276,0.272796801398346,1.28797193184368));
#19996=CARTESIAN_POINT('Ctrl Pts',(-1.04067701160391,0.293809324770207,
1.28727233489076));
#19997=CARTESIAN_POINT('Origin',(0.,0.,1.37171309575435));
#19998=CARTESIAN_POINT('',(-1.15799828028598,0.500065917147839,1.10727038327973));
#19999=CARTESIAN_POINT('Ctrl Pts',(-1.4127766116927,1.21572094522251,1.63615580822897));
#20000=CARTESIAN_POINT('Ctrl Pts',(-1.42835456209775,1.13112438230172,1.59808263051822));
#20001=CARTESIAN_POINT('Ctrl Pts',(-1.4332608863651,1.04649945489987,1.55687869031203));
#20002=CARTESIAN_POINT('Ctrl Pts',(-1.41427936788009,0.863161299579019,
1.4528510278119));
#20003=CARTESIAN_POINT('Ctrl Pts',(-1.38392755544946,0.771992498477371,
1.3904370872311));
#20004=CARTESIAN_POINT('Ctrl Pts',(-1.2883224397548,0.614269670090823,1.25222975809873));
#20005=CARTESIAN_POINT('Ctrl Pts',(-1.22690987286759,0.551263454538706,
1.18062438818012));
#20006=CARTESIAN_POINT('Ctrl Pts',(-1.15799828028598,0.500065917147839,
1.10727038327973));
#20007=CARTESIAN_POINT('Origin',(0.,0.,1.10727038327973));
#20008=CARTESIAN_POINT('Ctrl Pts',(-0.896396663228496,0.598371737951084,
1.28318517918604));
#20009=CARTESIAN_POINT('Ctrl Pts',(-1.05584851328029,0.762485056494505,
1.53750926858099));
#20010=CARTESIAN_POINT('Ctrl Pts',(-1.08712687701302,0.978314425275392,
1.74606924121326));
#20011=CARTESIAN_POINT('Ctrl Pts',(-0.990231754426695,1.24585984429374,
1.90886509708283));
#20012=CARTESIAN_POINT('Ctrl Pts',(-0.909465623084801,0.605275301161475,
1.26845681306972));
#20013=CARTESIAN_POINT('Ctrl Pts',(-1.0713094336526,0.771441249464592,1.51984840181957));
#20014=CARTESIAN_POINT('Ctrl Pts',(-1.1033694726,0.990069682591155,1.72608377212011));
#20015=CARTESIAN_POINT('Ctrl Pts',(-1.00546683912554,1.26141584343747,1.88700775532558));
#20016=CARTESIAN_POINT('Ctrl Pts',(-0.932013737380385,0.621016981690704,
1.24112031232197));
#20017=CARTESIAN_POINT('Ctrl Pts',(-1.09786234356421,0.791422088358102,
1.48709491630373));
#20018=CARTESIAN_POINT('Ctrl Pts',(-1.13056538342229,1.01568188386468,1.68880590632087));
#20019=CARTESIAN_POINT('Ctrl Pts',(-1.03011319759962,1.29379626687142,1.84625481400099));
#20020=CARTESIAN_POINT('Ctrl Pts',(-0.971942506168049,0.673028944353635,
1.180578495595));
#20021=CARTESIAN_POINT('Ctrl Pts',(-1.14383306000902,0.856136223676182,
1.41443322333459));
#20022=CARTESIAN_POINT('Ctrl Pts',(-1.17416051125987,1.09349602729721,1.60624275382303));
#20023=CARTESIAN_POINT('Ctrl Pts',(-1.06283879403329,1.38525239147929,1.75591724097872));
#20024=CARTESIAN_POINT('Ctrl Pts',(-0.99442467311732,0.726981684724077,
1.1340877844534));
#20025=CARTESIAN_POINT('Ctrl Pts',(-1.16852049530615,0.92230736881738,1.35876508657127));
#20026=CARTESIAN_POINT('Ctrl Pts',(-1.19379986392409,1.17034433001556,1.54303391436824));
#20027=CARTESIAN_POINT('Ctrl Pts',(-1.0700086698298,1.47122482340641,1.68683916414417));
#20028=CARTESIAN_POINT('Ctrl Pts',(-1.00715189764781,0.769660843866381,
1.101666983688));
#20029=CARTESIAN_POINT('Ctrl Pts',(-1.18199184824263,0.974320315501956,
1.31997051162988));
#20030=CARTESIAN_POINT('Ctrl Pts',(-1.20248619530708,1.23004502025839,1.49898794576059));
#20031=CARTESIAN_POINT('Ctrl Pts',(-1.06863493884117,1.53683495813568,1.63871928608012));
#20032=CARTESIAN_POINT('',(-0.89895057878464,0.601016155111926,1.28727233489076));
#20033=CARTESIAN_POINT('',(-1.00491994924733,0.762339710524743,1.10727038327973));
#20034=CARTESIAN_POINT('Ctrl Pts',(-0.89895057878464,0.601016155111926,
1.28727233489076));
#20035=CARTESIAN_POINT('Ctrl Pts',(-0.927868295879635,0.616327103756397,
1.25472274024264));
#20036=CARTESIAN_POINT('Ctrl Pts',(-0.946670056292164,0.636369305963792,
1.22803799031384));
#20037=CARTESIAN_POINT('Ctrl Pts',(-0.978914242877163,0.690422681628326,
1.17079203987024));
#20038=CARTESIAN_POINT('Ctrl Pts',(-0.99331738130894,0.722616466765028,
1.14052203161));
#20039=CARTESIAN_POINT('Ctrl Pts',(-1.00491994924733,0.762339710524743,
1.10727038327973));
#20040=CARTESIAN_POINT('Ctrl Pts',(-0.89895057878464,0.601016155111926,
1.28727233489076));
#20041=CARTESIAN_POINT('Ctrl Pts',(-0.969072704191387,0.674061841710201,
1.39987124007464));
#20042=CARTESIAN_POINT('Ctrl Pts',(-1.01397342270847,0.757283981982513,
1.50346488650363));
#20043=CARTESIAN_POINT('Ctrl Pts',(-1.05808377148838,0.966632999495317,
1.715480776583));
#20044=CARTESIAN_POINT('Ctrl Pts',(-1.04364312863621,1.09826755410688,1.81902921434248));
#20045=CARTESIAN_POINT('Ctrl Pts',(-0.990330805779365,1.24558623976355,
1.90869858745619));
#20046=CARTESIAN_POINT('Ctrl Pts',(-1.00491994924733,0.762339710524743,
1.10727038327973));
#20047=CARTESIAN_POINT('Ctrl Pts',(-1.05844250017153,0.823177646383102,
1.17697999301248));
#20048=CARTESIAN_POINT('Ctrl Pts',(-1.10067719707672,0.894287935370973,
1.24430717677953));
#20049=CARTESIAN_POINT('Ctrl Pts',(-1.1544631922219,1.06468657657252,1.37795460947454));
#20050=CARTESIAN_POINT('Ctrl Pts',(-1.16163314380192,1.15998911590306,1.43952296396723));
#20051=CARTESIAN_POINT('Ctrl Pts',(-1.1382431962131,1.34351349395869,1.54471868724281));
#20052=CARTESIAN_POINT('Ctrl Pts',(-1.11338277308106,1.43184312013679,1.59041399531266));
#20053=CARTESIAN_POINT('Ctrl Pts',(-1.07301833748062,1.5239904260293,1.63615580822897));
#20054=CARTESIAN_POINT('Ctrl Pts',(-1.16512557173636,0.498487526286222,
1.10192461715937));
#20055=CARTESIAN_POINT('Ctrl Pts',(-1.38489530661629,0.653828920782168,
1.32030517702043));
#20056=CARTESIAN_POINT('Ctrl Pts',(-1.46761240439959,0.896616198000948,
1.49938098964775));
#20057=CARTESIAN_POINT('Ctrl Pts',(-1.41327686508626,1.22684935794256,1.63915205504132));
#20058=CARTESIAN_POINT('Ctrl Pts',(-1.13261600897808,0.505885883797787,
1.12620814253777));
#20059=CARTESIAN_POINT('Ctrl Pts',(-1.34532824088584,0.661326782584695,
1.3493730700966));
#20060=CARTESIAN_POINT('Ctrl Pts',(-1.4226134838877,0.900220838946926,1.53236753871639));
#20061=CARTESIAN_POINT('Ctrl Pts',(-1.3643314634289,1.22259355973874,1.67519578767207));
#20062=CARTESIAN_POINT('Ctrl Pts',(-1.07994282031224,0.513157335393552,
1.16792434557147));
#20063=CARTESIAN_POINT('Ctrl Pts',(-1.28144653067711,0.667784226973452,
1.39930822300789));
#20064=CARTESIAN_POINT('Ctrl Pts',(-1.35050022373305,0.899713500733371,
1.58909081893482));
#20065=CARTESIAN_POINT('Ctrl Pts',(-1.28704482486114,1.20909629592349,1.73717568232662));
#20066=CARTESIAN_POINT('Ctrl Pts',(-1.01174252544333,0.5102156806996,1.22815018770195));
#20067=CARTESIAN_POINT('Ctrl Pts',(-1.19913545447318,0.661195786769768,
1.47154587959366));
#20068=CARTESIAN_POINT('Ctrl Pts',(-1.25930861084253,0.882510125799203,
1.6711373385863));
#20069=CARTESIAN_POINT('Ctrl Pts',(-1.19227095916867,1.17416443346653,1.82691854455345));
#20070=CARTESIAN_POINT('Ctrl Pts',(-0.978417148622634,0.496845910594337,
1.26357751389222));
#20071=CARTESIAN_POINT('Ctrl Pts',(-1.15942263970987,0.643602406938538,
1.51402822523202));
#20072=CARTESIAN_POINT('Ctrl Pts',(-1.21709221666582,0.857945526599464,
1.71951214242024));
#20073=CARTESIAN_POINT('Ctrl Pts',(-1.15128697696661,1.14019993459331,1.87982452105687));
#20074=CARTESIAN_POINT('Ctrl Pts',(-0.961857913410637,0.486216000974361,
1.28318566992362));
#20075=CARTESIAN_POINT('Ctrl Pts',(-1.13991207295831,0.629977719122414,
1.5375404757467));
#20076=CARTESIAN_POINT('Ctrl Pts',(-1.19691393144611,0.840512044007264,
1.74612008846831));
#20077=CARTESIAN_POINT('Ctrl Pts',(-1.13286348887405,1.11781897562891,1.90892450808844));
#20078=CARTESIAN_POINT('',(-0.964710998256926,0.488533777383804,1.28727233489076));
#20079=CARTESIAN_POINT('Ctrl Pts',(-1.15799828028598,0.500065917147839,
1.10727038327973));
#20080=CARTESIAN_POINT('Ctrl Pts',(-1.13262370376054,0.50640929218822,1.12805083925429));
#20081=CARTESIAN_POINT('Ctrl Pts',(-1.10478303295006,0.511371411500259,
1.15131250789239));
#20082=CARTESIAN_POINT('Ctrl Pts',(-1.05860800687958,0.513808202166494,
1.19194777349505));
#20083=CARTESIAN_POINT('Ctrl Pts',(-1.03731460867033,0.513729024230272,
1.21108489279944));
#20084=CARTESIAN_POINT('Ctrl Pts',(-1.00241946522331,0.507067244033085,
1.24526606650681));
#20085=CARTESIAN_POINT('Ctrl Pts',(-0.984791876090385,0.501447516417348,
1.26352342884092));
#20086=CARTESIAN_POINT('Ctrl Pts',(-0.964710998256925,0.488533777383804,
1.28727233489076));
#20087=CARTESIAN_POINT('Ctrl Pts',(-0.964710998256925,0.488533777383804,
1.28727233489076));
#20088=CARTESIAN_POINT('Ctrl Pts',(-1.04310952295002,0.552615413818275,
1.39987124007464));
#20089=CARTESIAN_POINT('Ctrl Pts',(-1.09769367964031,0.629833086622262,
1.50346488650363));
#20090=CARTESIAN_POINT('Ctrl Pts',(-1.16666286599128,0.832357123065218,
1.715480776583));
#20091=CARTESIAN_POINT('Ctrl Pts',(-1.16815913695893,0.964772942765737,
1.81902921434248));
#20092=CARTESIAN_POINT('Ctrl Pts',(-1.13295228123076,1.11743425489732,1.90869858745619));
#20093=CARTESIAN_POINT('Ctrl Pts',(-0.964710998256926,0.488533777383804,
1.28727233489076));
#20094=CARTESIAN_POINT('Ctrl Pts',(-1.14098448197888,0.632616760336964,
1.54044293163017));
#20095=CARTESIAN_POINT('Ctrl Pts',(-1.19686606932897,0.843108069941918,
1.74808806329354));
#20096=CARTESIAN_POINT('Ctrl Pts',(-1.13235576030722,1.12000770619867,1.91020772988088));
#20097=CARTESIAN_POINT('Ctrl Pts',(-0.94279085843283,0.526027903293178,
1.28727233489076));
#20098=CARTESIAN_POINT('Ctrl Pts',(-1.11286137791709,0.676829228446517,
1.54044293163017));
#20099=CARTESIAN_POINT('Ctrl Pts',(-1.16016893831867,0.889051558128351,
1.74808806329354));
#20100=CARTESIAN_POINT('Ctrl Pts',(-1.08471353963759,1.16269489233868,1.91020772988088));
#20101=CARTESIAN_POINT('Ctrl Pts',(-0.920870718608735,0.563522029202552,
1.28727233489076));
#20102=CARTESIAN_POINT('Ctrl Pts',(-1.0847382738553,0.721041696556071,1.54044293163017));
#20103=CARTESIAN_POINT('Ctrl Pts',(-1.12347180730837,0.934995046314783,
1.74808806329354));
#20104=CARTESIAN_POINT('Ctrl Pts',(-1.03707131896797,1.20538207847869,1.91020772988088));
#20105=CARTESIAN_POINT('Ctrl Pts',(-0.89895057878464,0.601016155111926,
1.28727233489076));
#20106=CARTESIAN_POINT('Ctrl Pts',(-1.05661516979351,0.765254164665624,
1.54044293163017));
#20107=CARTESIAN_POINT('Ctrl Pts',(-1.08677467629807,0.980938534501216,
1.74808806329354));
#20108=CARTESIAN_POINT('Ctrl Pts',(-0.989429098298345,1.2480692646187,1.91020772988088));
#20109=CARTESIAN_POINT('Ctrl Pts',(-0.964710998256926,0.488533777383804,
1.28727233489076));
#20110=CARTESIAN_POINT('Ctrl Pts',(-0.954255105111255,0.507642157628472,
1.28796759655004));
#20111=CARTESIAN_POINT('Ctrl Pts',(-0.943523700818286,0.526600254136218,
1.2883190755065));
#20112=CARTESIAN_POINT('Ctrl Pts',(-0.932521031881151,0.545412103245543,
1.288319084765));
#20113=CARTESIAN_POINT('Ctrl Pts',(-0.921586204420601,0.564107960168957,
1.28831909396641));
#20114=CARTESIAN_POINT('Ctrl Pts',(-0.910394454615245,0.582640621209113,
1.28797193184368));
#20115=CARTESIAN_POINT('Ctrl Pts',(-0.89895057878464,0.601016155111926,
1.28727233489076));
#20116=CARTESIAN_POINT('Origin',(0.,0.,1.37171309575435));
#20117=CARTESIAN_POINT('',(-0.946792943618189,0.833432097145896,1.10727038327973));
#20118=CARTESIAN_POINT('Ctrl Pts',(-0.967951970128403,1.59279130921887,
1.63615580822897));
#20119=CARTESIAN_POINT('Ctrl Pts',(-1.00890925697988,1.51714904820957,1.59808263051822));
#20120=CARTESIAN_POINT('Ctrl Pts',(-1.03972598936032,1.43818209714157,1.55687869031203));
#20121=CARTESIAN_POINT('Ctrl Pts',(-1.07832809822747,1.25795153804723,1.4528510278119));
#20122=CARTESIAN_POINT('Ctrl Pts',(-1.07763451813115,1.16186562982554,1.3904370872311));
#20123=CARTESIAN_POINT('Ctrl Pts',(-1.03544768423092,0.982318700621183,
1.25222975809873));
#20124=CARTESIAN_POINT('Ctrl Pts',(-0.996510853667281,0.903418701916912,
1.18062438818013));
#20125=CARTESIAN_POINT('Ctrl Pts',(-0.946792943618189,0.833432097145896,
1.10727038327973));
#20126=CARTESIAN_POINT('Origin',(0.,0.,1.10727038327973));
#20127=CARTESIAN_POINT('Ctrl Pts',(-0.667616851768136,0.846087143183836,
1.28318517918604));
#20128=CARTESIAN_POINT('Ctrl Pts',(-0.768550768362021,1.05144151564591,
1.53750926858099));
#20129=CARTESIAN_POINT('Ctrl Pts',(-0.731603317170576,1.2663729891825,1.74606924121326));
#20130=CARTESIAN_POINT('Ctrl Pts',(-0.556774498193799,1.4908815637936,1.90886509708283));
#20131=CARTESIAN_POINT('Ctrl Pts',(-0.677912852846923,0.856691352655137,
1.26845681306972));
#20132=CARTESIAN_POINT('Ctrl Pts',(-0.780487361597375,1.06473704847503,
1.51984840181957));
#20133=CARTESIAN_POINT('Ctrl Pts',(-0.743418369261302,1.28257214132251,
1.72608377212011));
#20134=CARTESIAN_POINT('Ctrl Pts',(-0.566456856673053,1.5103840982294,1.88700775532558));
#20135=CARTESIAN_POINT('Ctrl Pts',(-0.694492950134685,0.878631748253103,
1.24111924840996));
#20136=CARTESIAN_POINT('Ctrl Pts',(-0.799566273875777,1.0919466731633,1.48709385239173));
#20137=CARTESIAN_POINT('Ctrl Pts',(-0.76136794175864,1.31533666464122,1.68880445881716));
#20138=CARTESIAN_POINT('Ctrl Pts',(-0.579890165126716,1.54879772833386,
1.84625336649728));
#20139=CARTESIAN_POINT('Ctrl Pts',(-0.716394511678363,0.940438249469778,
1.18057655035131));
#20140=CARTESIAN_POINT('Ctrl Pts',(-0.823288881893973,1.16770072295994,
1.41443127809089));
#20141=CARTESIAN_POINT('Ctrl Pts',(-0.778782224872494,1.4028158039603,1.60624011348192));
#20142=CARTESIAN_POINT('Ctrl Pts',(-0.582751305549681,1.64589229282024,
1.75591460063761));
#20143=CARTESIAN_POINT('Ctrl Pts',(-0.721104370153833,0.99869479210307,
1.13408778445339));
#20144=CARTESIAN_POINT('Ctrl Pts',(-0.826320380483541,1.23825912446584,
1.35876508657127));
#20145=CARTESIAN_POINT('Ctrl Pts',(-0.7737148524921,1.48196804720543,1.54303391436825));
#20146=CARTESIAN_POINT('Ctrl Pts',(-0.563005244955075,1.72986881834181,
1.68683916414417));
#20147=CARTESIAN_POINT('Ctrl Pts',(-0.720020094497306,1.0432180131865,1.101666983688));
#20148=CARTESIAN_POINT('Ctrl Pts',(-0.82305951402404,1.29188925333651,1.31997051162988));
#20149=CARTESIAN_POINT('Ctrl Pts',(-0.76352751669565,1.54143100170431,1.49898794576059));
#20150=CARTESIAN_POINT('Ctrl Pts',(-0.541424102512135,1.79184325828989,
1.63871928608012));
#20151=CARTESIAN_POINT('',(-0.669228599956957,0.849391336665505,1.28727233489076));
#20152=CARTESIAN_POINT('',(-0.720159740047643,1.03556549162895,1.10727038327973));
#20153=CARTESIAN_POINT('Ctrl Pts',(-0.669228599956957,0.849391336665505,
1.28727233489076));
#20154=CARTESIAN_POINT('Ctrl Pts',(-0.691999639905444,0.872888980165426,
1.25472274024256));
#20155=CARTESIAN_POINT('Ctrl Pts',(-0.7036877955768,0.897760310667323,1.22803799031376));
#20156=CARTESIAN_POINT('Ctrl Pts',(-0.717650427656563,0.959132127441791,
1.17079203987355));
#20157=CARTESIAN_POINT('Ctrl Pts',(-0.721400199597664,0.994201051127123,
1.14052203161356));
#20158=CARTESIAN_POINT('Ctrl Pts',(-0.720159740047643,1.03556549162895,
1.10727038327973));
#20159=CARTESIAN_POINT('Ctrl Pts',(-0.669228599956957,0.849391336665505,
1.28727233489076));
#20160=CARTESIAN_POINT('Ctrl Pts',(-0.713346345736856,0.940530841324424,
1.39987124007464));
#20161=CARTESIAN_POINT('Ctrl Pts',(-0.73033241101646,1.03355488521186,1.50346488650363));
#20162=CARTESIAN_POINT('Ctrl Pts',(-0.707591441492497,1.2462884798982,1.715480776583));
#20163=CARTESIAN_POINT('Ctrl Pts',(-0.653180259586497,1.36701797678012,
1.81902921434248));
#20164=CARTESIAN_POINT('Ctrl Pts',(-0.55695325007777,1.49065195897357,1.90869858745619));
#20165=CARTESIAN_POINT('Ctrl Pts',(-0.720159740047643,1.03556549162895,
1.10727038327973));
#20166=CARTESIAN_POINT('Ctrl Pts',(-0.752262754789917,1.10996518478287,
1.17697999301248));
#20167=CARTESIAN_POINT('Ctrl Pts',(-0.770456050723177,1.19064632759638,
1.24430717677952));
#20168=CARTESIAN_POINT('Ctrl Pts',(-0.768953495941758,1.36932585223818,
1.37795460947453));
#20169=CARTESIAN_POINT('Ctrl Pts',(-0.746322420853235,1.46217959017503,
1.43952296396722));
#20170=CARTESIAN_POINT('Ctrl Pts',(-0.667365107081823,1.62949375452132,
1.54471868724278));
#20171=CARTESIAN_POINT('Ctrl Pts',(-0.616426084068442,1.70581792784477,
1.59041399531263));
#20172=CARTESIAN_POINT('Ctrl Pts',(-0.549562141057365,1.78098192700405,
1.63615580822897));
#20173=CARTESIAN_POINT('Ctrl Pts',(-0.954059150195613,0.834133412413726,
1.10192461715937));
#20174=CARTESIAN_POINT('Ctrl Pts',(-1.11506945780848,1.04978444082665,1.32030517702044));
#20175=CARTESIAN_POINT('Ctrl Pts',(-1.11871269798568,1.30624985183955,1.49938098964776));
#20176=CARTESIAN_POINT('Ctrl Pts',(-0.96498887072721,1.60352964545243,1.63915205504134));
#20177=CARTESIAN_POINT('Ctrl Pts',(-0.920854500490905,0.831123661162971,
1.12620814253776));
#20178=CARTESIAN_POINT('Ctrl Pts',(-1.0751219753964,1.04468843542396,1.3493730700966));
#20179=CARTESIAN_POINT('Ctrl Pts',(-1.07480228609568,1.29577263793342,1.5323675387164));
#20180=CARTESIAN_POINT('Ctrl Pts',(-0.919754141507906,1.58435717993001,
1.67519578767208));
#20181=CARTESIAN_POINT('Ctrl Pts',(-0.868512346714968,0.821762669862001,
1.16792406090531));
#20182=CARTESIAN_POINT('Ctrl Pts',(-1.01237142622958,1.03108965362589,1.39930793834173));
#20183=CARTESIAN_POINT('Ctrl Pts',(-1.00637513236489,1.27300639515448,1.589090429871));
#20184=CARTESIAN_POINT('Ctrl Pts',(-0.850420920292679,1.5476381219134,1.73717529326279));
#20185=CARTESIAN_POINT('Ctrl Pts',(-0.80455912762015,0.797889917227132,
1.22814985715448));
#20186=CARTESIAN_POINT('Ctrl Pts',(-0.936124975293412,0.999388130632026,
1.4715455490462));
#20187=CARTESIAN_POINT('Ctrl Pts',(-0.924963031592627,1.22846526028813,
1.67113688711452));
#20188=CARTESIAN_POINT('Ctrl Pts',(-0.771080298579198,1.48512921647049,
1.82691809308168));
#20189=CARTESIAN_POINT('Ctrl Pts',(-0.776996174893135,0.774876067377614,
1.26357751389222));
#20190=CARTESIAN_POINT('Ctrl Pts',(-0.903792375271581,0.970383562355559,
1.51402822523203));
#20191=CARTESIAN_POINT('Ctrl Pts',(-0.892403735624943,1.19205686236992,
1.71951214242025));
#20192=CARTESIAN_POINT('Ctrl Pts',(-0.74259782479529,1.44016181895953,1.87982452105689));
#20193=CARTESIAN_POINT('Ctrl Pts',(-0.764532229061142,0.75964933747155,
1.28318566992362));
#20194=CARTESIAN_POINT('Ctrl Pts',(-0.889446983704125,0.951396617529428,
1.53754047574671));
#20195=CARTESIAN_POINT('Ctrl Pts',(-0.878600288371208,1.16924120209866,
1.74612008846832));
#20196=CARTESIAN_POINT('Ctrl Pts',(-0.73199214306239,1.41318309117925,1.90892450808845));
#20197=CARTESIAN_POINT('',(-0.766529441696069,0.762735325532963,1.28727233489076));
#20198=CARTESIAN_POINT('Ctrl Pts',(-0.946792943618189,0.833432097145897,
1.10727038327973));
#20199=CARTESIAN_POINT('Ctrl Pts',(-0.920700076575993,0.831623829941906,
1.12805083925451));
#20200=CARTESIAN_POINT('Ctrl Pts',(-0.892688645988233,0.827739845432993,
1.15131250789253));
#20201=CARTESIAN_POINT('Ctrl Pts',(-0.848020576826102,0.815788503303454,
1.19194777349529));
#20202=CARTESIAN_POINT('Ctrl Pts',(-0.827793819032997,0.809133178696536,
1.21108489279973));
#20203=CARTESIAN_POINT('Ctrl Pts',(-0.79666516876339,0.792014256883052,
1.24526606650818));
#20204=CARTESIAN_POINT('Ctrl Pts',(-0.781636926589457,0.78122235370212,
1.26352342884212));
#20205=CARTESIAN_POINT('Ctrl Pts',(-0.766529441696069,0.762735325532963,
1.28727233489076));
#20206=CARTESIAN_POINT('Ctrl Pts',(-0.766529441696069,0.762735325532963,
1.28727233489076));
#20207=CARTESIAN_POINT('Ctrl Pts',(-0.821288554787752,0.847907059902912,
1.39987124007464));
#20208=CARTESIAN_POINT('Ctrl Pts',(-0.849339599532016,0.938212862837218,
1.50346488650363));
#20209=CARTESIAN_POINT('Ctrl Pts',(-0.852349824604395,1.15213731807335,
1.715480776583));
#20210=CARTESIAN_POINT('Ctrl Pts',(-0.812854124246773,1.27853461941729,
1.81902921434248));
#20211=CARTESIAN_POINT('Ctrl Pts',(-0.732195474855993,1.41284463836769,
1.90869858745619));
#20212=CARTESIAN_POINT('Ctrl Pts',(-0.766529441696069,0.762735325532963,
1.28727233489076));
#20213=CARTESIAN_POINT('Ctrl Pts',(-0.889651396707116,0.954237887485567,
1.54044293163017));
#20214=CARTESIAN_POINT('Ctrl Pts',(-0.877752552661174,1.17169537927269,
1.74808806329354));
#20215=CARTESIAN_POINT('Ctrl Pts',(-0.730832909558243,1.41510780089433,
1.91020772988088));
#20216=CARTESIAN_POINT('Ctrl Pts',(-0.734095827783032,0.791620662577143,
1.28727233489076));
#20217=CARTESIAN_POINT('Ctrl Pts',(-0.849242331321591,0.987595926292982,
1.54044293163017));
#20218=CARTESIAN_POINT('Ctrl Pts',(-0.828654188454019,1.20405019596674,
1.74808806329354));
#20219=CARTESIAN_POINT('Ctrl Pts',(-0.672331399180314,1.44098347159841,
1.91020772988088));
#20220=CARTESIAN_POINT('Ctrl Pts',(-0.701662213869994,0.820505999621324,
1.28727233489076));
#20221=CARTESIAN_POINT('Ctrl Pts',(-0.808833265936067,1.0209539651004,1.54044293163017));
#20222=CARTESIAN_POINT('Ctrl Pts',(-0.779555824246864,1.23640501266079,
1.74808806329354));
#20223=CARTESIAN_POINT('Ctrl Pts',(-0.613829888802386,1.4668591423025,1.91020772988088));
#20224=CARTESIAN_POINT('Ctrl Pts',(-0.669228599956957,0.849391336665504,
1.28727233489076));
#20225=CARTESIAN_POINT('Ctrl Pts',(-0.768424200550542,1.05431200390781,
1.54044293163017));
#20226=CARTESIAN_POINT('Ctrl Pts',(-0.730457460039709,1.26875982935484,
1.74808806329354));
#20227=CARTESIAN_POINT('Ctrl Pts',(-0.555328378424457,1.49273481300659,
1.91020772988088));
#20228=CARTESIAN_POINT('Ctrl Pts',(-0.766529441696069,0.762735325532963,
1.28727233489076));
#20229=CARTESIAN_POINT('Ctrl Pts',(-0.750680482155644,0.777677426407089,
1.28796759655004));
#20230=CARTESIAN_POINT('Ctrl Pts',(-0.734615936171909,0.792391461327313,
1.2883190755065));
#20231=CARTESIAN_POINT('Ctrl Pts',(-0.718338595112193,0.806882581321256,
1.288319084765));
#20232=CARTESIAN_POINT('Ctrl Pts',(-0.702161618687529,0.82128435036013,
1.28831909396641));
#20233=CARTESIAN_POINT('Ctrl Pts',(-0.685790724893994,0.835451517520017,
1.28797193184368));
#20234=CARTESIAN_POINT('Ctrl Pts',(-0.669228599956957,0.849391336665505,
1.28727233489076));
#20235=CARTESIAN_POINT('Origin',(0.,0.,1.37171309575435));
#20236=CARTESIAN_POINT('',(-0.642908916934714,1.08521613661244,1.10727038327973));
#20237=CARTESIAN_POINT('Ctrl Pts',(-0.428377445609996,1.81394816223928,
1.63615580822897));
#20238=CARTESIAN_POINT('Ctrl Pts',(-0.490704884304683,1.75466459467969,
1.59808263051822));
#20239=CARTESIAN_POINT('Ctrl Pts',(-0.544415468320009,1.68908545531116,
1.55687869031203));
#20240=CARTESIAN_POINT('Ctrl Pts',(-0.636822561166696,1.52960471530763,
1.4528510278119));
#20241=CARTESIAN_POINT('Ctrl Pts',(-0.665855105856971,1.43800725813254,
1.3904370872311));
#20242=CARTESIAN_POINT('Ctrl Pts',(-0.681216094986278,1.2542115325179,1.25222975809873));
#20243=CARTESIAN_POINT('Ctrl Pts',(-0.66856640901063,1.16714103226325,1.18062438818012));
#20244=CARTESIAN_POINT('Ctrl Pts',(-0.642908916934714,1.08521613661244,
1.10727038327973));
#20245=CARTESIAN_POINT('Origin',(0.,0.,1.10727038327973));
#20246=CARTESIAN_POINT('Ctrl Pts',(-0.373486051296586,1.01098164380599,
1.28318517918604));
#20247=CARTESIAN_POINT('Ctrl Pts',(-0.40602191942841,1.23747555342209,1.537509268581));
#20248=CARTESIAN_POINT('Ctrl Pts',(-0.304465327263429,1.43047014156898,
1.74606924121326));
#20249=CARTESIAN_POINT('Ctrl Pts',(-0.0688162748016438,1.58996540824669,
1.90886509708284));
#20250=CARTESIAN_POINT('Ctrl Pts',(-0.382166213971436,1.02865698469238,
1.26356265747109));
#20251=CARTESIAN_POINT('Ctrl Pts',(-0.415747810278512,1.25921979945503,
1.51398032870897));
#20252=CARTESIAN_POINT('Ctrl Pts',(-0.312707553760736,1.45578649927555,
1.71944252353204));
#20253=CARTESIAN_POINT('Ctrl Pts',(-0.0730554435692729,1.61866306691267,
1.87974468006744));
#20254=CARTESIAN_POINT('Ctrl Pts',(-0.391657241669877,1.0633167753106,1.22810806352261));
#20255=CARTESIAN_POINT('Ctrl Pts',(-0.425647906592845,1.30153367691802,
1.4714667110343));
#20256=CARTESIAN_POINT('Ctrl Pts',(-0.318676377131988,1.50438827167773,
1.67103178775816));
#20257=CARTESIAN_POINT('Ctrl Pts',(-0.0707311879560992,1.67188067012364,
1.82679988540378));
#20258=CARTESIAN_POINT('Ctrl Pts',(-0.386793101125269,1.13146507111567,
1.16783895333641));
#20259=CARTESIAN_POINT('Ctrl Pts',(-0.416728995650738,1.38370624635607,
1.39917869757247));
#20260=CARTESIAN_POINT('Ctrl Pts',(-0.298796521842128,1.59505828371836,
1.58892894777221));
#20261=CARTESIAN_POINT('Ctrl Pts',(-0.0329933807603502,1.76565888855501,
1.73699566095833));
#20262=CARTESIAN_POINT('Ctrl Pts',(-0.373540819382843,1.18300585575676,
1.1260986586408));
#20263=CARTESIAN_POINT('Ctrl Pts',(-0.398429005793491,1.4453045731053,1.34921513358857));
#20264=CARTESIAN_POINT('Ctrl Pts',(-0.270901963247257,1.66164003747218,
1.53217466057836));
#20265=CARTESIAN_POINT('Ctrl Pts',(0.00890514499184177,1.83206393610154,
1.674981645914));
#20266=CARTESIAN_POINT('Ctrl Pts',(-0.362468171451202,1.21448591285885,
1.10179959977345));
#20267=CARTESIAN_POINT('Ctrl Pts',(-0.383640993960513,1.48279448162749,
1.32012924726704));
#20268=CARTESIAN_POINT('Ctrl Pts',(-0.249943984819036,1.7017123916886,1.49916808705051));
#20269=CARTESIAN_POINT('Ctrl Pts',(0.0386228559732295,1.87123964304219,
1.63891611912388));
#20270=CARTESIAN_POINT('',(-0.373997862975653,1.01462217612883,1.28727233489076));
#20271=CARTESIAN_POINT('',(-0.364905277844141,1.20742290720348,1.10727038327973));
#20272=CARTESIAN_POINT('Ctrl Pts',(-0.373997862975653,1.01462217612883,
1.28727233489076));
#20273=CARTESIAN_POINT('Ctrl Pts',(-0.388393237732322,1.04400640142086,
1.25472274024237));
#20274=CARTESIAN_POINT('Ctrl Pts',(-0.391823670549201,1.07127228109886,
1.22803799031368));
#20275=CARTESIAN_POINT('Ctrl Pts',(-0.386137988413871,1.13395503796173,
1.17079203987004));
#20276=CARTESIAN_POINT('Ctrl Pts',(-0.378867340058857,1.16846630960703,
1.1405220316102));
#20277=CARTESIAN_POINT('Ctrl Pts',(-0.364905277844141,1.20742290720348,
1.10727038327973));
#20278=CARTESIAN_POINT('Ctrl Pts',(-0.373997862975653,1.01462217612883,
1.28727233489076));
#20279=CARTESIAN_POINT('Ctrl Pts',(-0.387792676785359,1.11493412912611,
1.39987124007464));
#20280=CARTESIAN_POINT('Ctrl Pts',(-0.375201374409042,1.20865423507634,
1.50346488650363));
#20281=CARTESIAN_POINT('Ctrl Pts',(-0.287835131123856,1.40394856048621,
1.715480776583));
#20282=CARTESIAN_POINT('Ctrl Pts',(-0.198779555753984,1.50195515531182,
1.81902921434248));
#20283=CARTESIAN_POINT('Ctrl Pts',(-0.0690572297370878,1.58980227845634,
1.90869858745619));
#20284=CARTESIAN_POINT('Ctrl Pts',(-0.364905277844141,1.20742290720348,
1.10727038327973));
#20285=CARTESIAN_POINT('Ctrl Pts',(-0.372446289646659,1.2881015973139,1.17697999301248));
#20286=CARTESIAN_POINT('Ctrl Pts',(-0.364817298041905,1.3704559615559,1.24430717677952));
#20287=CARTESIAN_POINT('Ctrl Pts',(-0.308173273864789,1.53992597283257,
1.37795460947454));
#20288=CARTESIAN_POINT('Ctrl Pts',(-0.257956459417352,1.62124173855646,
1.43952296396723));
#20289=CARTESIAN_POINT('Ctrl Pts',(-0.127450637982162,1.75990988600072,
1.54779670475201));
#20290=CARTESIAN_POINT('Ctrl Pts',(-0.0535283678677282,1.81609416413934,
1.5933649555937));
#20291=CARTESIAN_POINT('Ctrl Pts',(0.0276890267571703,1.86363850813291,
1.63615580822897));
#20292=CARTESIAN_POINT('Ctrl Pts',(-0.649602771712747,1.08812850838495,
1.10192461715937));
#20293=CARTESIAN_POINT('Ctrl Pts',(-0.736092841324624,1.34297974552473,
1.32030517702043));
#20294=CARTESIAN_POINT('Ctrl Pts',(-0.660305598163237,1.58801866900221,
1.49938098964775));
#20295=CARTESIAN_POINT('Ctrl Pts',(-0.422241042228588,1.82324527881738,
1.63915205504133));
#20296=CARTESIAN_POINT('Ctrl Pts',(-0.618953337525111,1.07500526379448,
1.12620814253776));
#20297=CARTESIAN_POINT('Ctrl Pts',(-0.699675280139882,1.3257887054316,1.3493730700966));
#20298=CARTESIAN_POINT('Ctrl Pts',(-0.621781951952739,1.56448518294015,
1.5323675387164));
#20299=CARTESIAN_POINT('Ctrl Pts',(-0.385144875912219,1.79103288048413,
1.67519578767208));
#20300=CARTESIAN_POINT('Ctrl Pts',(-0.572065282586332,1.04992951600932,
1.16792267552995));
#20301=CARTESIAN_POINT('Ctrl Pts',(-0.644197802222636,1.29346620831953,
1.39930655296637));
#20302=CARTESIAN_POINT('Ctrl Pts',(-0.563737612015956,1.52169008642819,
1.58908853641612));
#20303=CARTESIAN_POINT('Ctrl Pts',(-0.330550471617962,1.73468787786897,
1.73717339980791));
#20304=CARTESIAN_POINT('Ctrl Pts',(-0.518619720423095,1.00746259753275,
1.22814823442989));
#20305=CARTESIAN_POINT('Ctrl Pts',(-0.581479904896343,1.23975486922368,
1.47154392632161));
#20306=CARTESIAN_POINT('Ctrl Pts',(-0.500074721257068,1.45417148278634,
1.67113467075223));
#20307=CARTESIAN_POINT('Ctrl Pts',(-0.274410020975489,1.65072103116966,
1.82691587671938));
#20308=CARTESIAN_POINT('Ctrl Pts',(-0.499517401914415,0.97705595580695,
1.26357751389222));
#20309=CARTESIAN_POINT('Ctrl Pts',(-0.559692616049941,1.20217681362938,
1.51402822523203));
#20310=CARTESIAN_POINT('Ctrl Pts',(-0.480360559198658,1.40948136690306,
1.71951214242025));
#20311=CARTESIAN_POINT('Ctrl Pts',(-0.261218023549743,1.59915063028856,
1.87982452105688));
#20312=CARTESIAN_POINT('Ctrl Pts',(-0.49236880332188,0.958722904028868,
1.28318566992362));
#20313=CARTESIAN_POINT('Ctrl Pts',(-0.551916626543442,1.17968618624264,
1.53754047574671));
#20314=CARTESIAN_POINT('Ctrl Pts',(-0.474283127502362,1.38351688474614,
1.74612008846831));
#20315=CARTESIAN_POINT('Ctrl Pts',(-0.25946830619864,1.57021499953936,1.90892450808845));
#20316=CARTESIAN_POINT('',(-0.493314642657339,0.962275025729455,1.28727233489076));
#20317=CARTESIAN_POINT('Ctrl Pts',(-0.642908916934714,1.08521613661244,
1.10727038327973));
#20318=CARTESIAN_POINT('Ctrl Pts',(-0.618651911001846,1.07543323295689,
1.12805083925448));
#20319=CARTESIAN_POINT('Ctrl Pts',(-0.59321167462972,1.06308333609212,1.15131250789253));
#20320=CARTESIAN_POINT('Ctrl Pts',(-0.554422984205854,1.037913741804,1.19194777349583));
#20321=CARTESIAN_POINT('Ctrl Pts',(-0.53724280281008,1.02533374006942,1.21108489280008));
#20322=CARTESIAN_POINT('Ctrl Pts',(-0.512927734894226,0.999433395982331,
1.24526606650743));
#20323=CARTESIAN_POINT('Ctrl Pts',(-0.501969908730524,0.984525703911643,
1.26352342884142));
#20324=CARTESIAN_POINT('Ctrl Pts',(-0.493314642657339,0.962275025729455,
1.28727233489076));
#20325=CARTESIAN_POINT('Ctrl Pts',(-0.493314642657339,0.962275025729455,
1.28727233489076));
#20326=CARTESIAN_POINT('Ctrl Pts',(-0.519074140629024,1.06019965524839,
1.39987124007464));
#20327=CARTESIAN_POINT('Ctrl Pts',(-0.517846241724568,1.15475382712427,
1.50346488650363));
#20328=CARTESIAN_POINT('Ctrl Pts',(-0.454602843714802,1.35913828497575,
1.715480776583));
#20329=CARTESIAN_POINT('Ctrl Pts',(-0.377981286365636,1.46714441944577,
1.81902921434248));
#20330=CARTESIAN_POINT('Ctrl Pts',(-0.259766273896473,1.5699559447672,1.90869858745619));
#20331=CARTESIAN_POINT('Ctrl Pts',(-0.493314642657339,0.962275025729455,
1.28727233489076));
#20332=CARTESIAN_POINT('Ctrl Pts',(-0.551233034159898,1.18245156164078,
1.54044293163017));
#20333=CARTESIAN_POINT('Ctrl Pts',(-0.472718500477254,1.38558898119851,
1.74808806329354));
#20334=CARTESIAN_POINT('Ctrl Pts',(-0.257771041609407,1.57168728440264,
1.91020772988088));
#20335=CARTESIAN_POINT('Ctrl Pts',(-0.453542382763444,0.979724075862581,
1.28727233489076));
#20336=CARTESIAN_POINT('Ctrl Pts',(-0.502493528317088,1.20168985388846,
1.54044293163017));
#20337=CARTESIAN_POINT('Ctrl Pts',(-0.416024993050259,1.4011880115129,1.74808806329354));
#20338=CARTESIAN_POINT('Ctrl Pts',(-0.194136776962956,1.57821854873589,
1.91020772988088));
#20339=CARTESIAN_POINT('Ctrl Pts',(-0.413770122869549,0.997173125995706,
1.28727233489076));
#20340=CARTESIAN_POINT('Ctrl Pts',(-0.453754022474278,1.22092814613614,
1.54044293163017));
#20341=CARTESIAN_POINT('Ctrl Pts',(-0.359331485623263,1.41678704182728,
1.74808806329354));
#20342=CARTESIAN_POINT('Ctrl Pts',(-0.130502512316506,1.58474981306913,
1.91020772988088));
#20343=CARTESIAN_POINT('Ctrl Pts',(-0.373997862975653,1.01462217612883,
1.28727233489076));
#20344=CARTESIAN_POINT('Ctrl Pts',(-0.405014516631467,1.24016643838382,
1.54044293163017));
#20345=CARTESIAN_POINT('Ctrl Pts',(-0.302637978196268,1.43238607214167,
1.74808806329354));
#20346=CARTESIAN_POINT('Ctrl Pts',(-0.066868247670056,1.59128107740238,
1.91020772988088));
#20347=CARTESIAN_POINT('Ctrl Pts',(-0.493314642657339,0.962275025729455,
1.28727233489076));
#20348=CARTESIAN_POINT('Ctrl Pts',(-0.473624023308118,0.971588210291795,
1.28796759655004));
#20349=CARTESIAN_POINT('Ctrl Pts',(-0.453798845322803,0.980617871367769,
1.2883190755065));
#20350=CARTESIAN_POINT('Ctrl Pts',(-0.433840171694363,0.989369770455727,
1.288319084765));
#20351=CARTESIAN_POINT('Ctrl Pts',(-0.414004561469676,0.998067706113494,
1.28831909396641));
#20352=CARTESIAN_POINT('Ctrl Pts',(-0.394057020835222,1.00648259836303,
1.28797193184368));
#20353=CARTESIAN_POINT('Ctrl Pts',(-0.373997862975653,1.01462217612883,
1.28727233489076));
#20354=CARTESIAN_POINT('Origin',(0.,0.,1.37171309575435));
#20355=CARTESIAN_POINT('',(-0.27609248605185,1.23077165948193,1.10727038327973));
#20356=CARTESIAN_POINT('Ctrl Pts',(0.153129647965883,1.85754313061971,1.63615580822897));
#20357=CARTESIAN_POINT('Ctrl Pts',(0.0607713534907839,1.81335940151627,
1.59083969670469));
#20358=CARTESIAN_POINT('Ctrl Pts',(-0.0223614442500398,1.75708539039456,
1.54129005514746));
#20359=CARTESIAN_POINT('Ctrl Pts',(-0.159600739735625,1.61733286423933,
1.42521036359322));
#20360=CARTESIAN_POINT('Ctrl Pts',(-0.208550308549109,1.53789592166466,
1.36183966503053));
#20361=CARTESIAN_POINT('Ctrl Pts',(-0.264206681902338,1.37907079095174,
1.23219371736399));
#20362=CARTESIAN_POINT('Ctrl Pts',(-0.275306576910198,1.30454791379682,
1.17031259812848));
#20363=CARTESIAN_POINT('Ctrl Pts',(-0.27609248605185,1.23077165948193,1.10727038327973));
#20364=CARTESIAN_POINT('Origin',(0.,0.,1.10727038327973));
#20365=CARTESIAN_POINT('Ctrl Pts',(-0.042795833893793,1.07691421720911,
1.28318517918604));
#20366=CARTESIAN_POINT('Ctrl Pts',(-0.00374881610008838,1.30237686203014,
1.53750926858099));
#20367=CARTESIAN_POINT('Ctrl Pts',(0.152475850210928,1.45454290982716,1.74606924121326));
#20368=CARTESIAN_POINT('Ctrl Pts',(0.425878165039256,1.53341236060018,1.90886509708283));
#20369=CARTESIAN_POINT('Ctrl Pts',(-0.0448924758011831,1.091545040475,1.26845681306972));
#20370=CARTESIAN_POINT('Ctrl Pts',(-0.00559080476410172,1.32014932750452,
1.51984840181958));
#20371=CARTESIAN_POINT('Ctrl Pts',(0.152438895007651,1.4745930125769,1.72608377212011));
#20372=CARTESIAN_POINT('Ctrl Pts',(0.429508274607602,1.55488138991364,1.88700775532559));
#20373=CARTESIAN_POINT('Ctrl Pts',(-0.0454099470705956,1.11904054473513,
1.24111941924413));
#20374=CARTESIAN_POINT('Ctrl Pts',(-0.00503268467650735,1.35337649424566,
1.4870940232259));
#20375=CARTESIAN_POINT('Ctrl Pts',(0.157175625948464,1.51165038249934,1.68880469124906));
#20376=CARTESIAN_POINT('Ctrl Pts',(0.441219201568124,1.59385438982847,1.84625359892919));
#20377=CARTESIAN_POINT('Ctrl Pts',(-0.026799925001142,1.18191630764682,
1.1805768626608));
#20378=CARTESIAN_POINT('Ctrl Pts',(0.0203022432084504,1.42860644524987,
1.41443159040039));
#20379=CARTESIAN_POINT('Ctrl Pts',(0.19450578395595,1.5926582292379,1.60624053738542));
#20380=CARTESIAN_POINT('Ctrl Pts',(0.49597490444196,1.6740871562873,1.75591502454111));
#20381=CARTESIAN_POINT('Ctrl Pts',(0.00363238016698291,1.2318155731452,
1.13408778445341));
#20382=CARTESIAN_POINT('Ctrl Pts',(0.0593232212680486,1.48747160844963,
1.35876508657129));
#20383=CARTESIAN_POINT('Ctrl Pts',(0.245130498049602,1.65371551508434,1.54303391436826));
#20384=CARTESIAN_POINT('Ctrl Pts',(0.561310568731024,1.73041945202573,1.68683916414419));
#20385=CARTESIAN_POINT('Ctrl Pts',(0.0306796703370947,1.26719829440569,
1.10166698368801));
#20386=CARTESIAN_POINT('Ctrl Pts',(0.093484316478892,1.52894260490193,1.3199705116299));
#20387=CARTESIAN_POINT('Ctrl Pts',(0.288323673548512,1.69583409006837,1.4989879457606));
#20388=CARTESIAN_POINT('Ctrl Pts',(0.615197741545956,1.76787274990501,1.63871928608014));
#20389=CARTESIAN_POINT('',(-0.0421576093699569,1.08053472770428,1.28727233489076));
#20390=CARTESIAN_POINT('',(0.0260686553993152,1.26108935601086,1.10727038327973));
#20391=CARTESIAN_POINT('Ctrl Pts',(-0.0421576093699569,1.08053472770428,
1.28727233489076));
#20392=CARTESIAN_POINT('Ctrl Pts',(-0.0467681993550378,1.11292920208489,
1.25472274024224));
#20393=CARTESIAN_POINT('Ctrl Pts',(-0.0416051146519907,1.13992065666392,
1.22803799031329));
#20394=CARTESIAN_POINT('Ctrl Pts',(-0.0168276724833753,1.19777852863159,
1.1707920398713));
#20395=CARTESIAN_POINT('Ctrl Pts',(0.000751694447766439,1.22835394451364,
1.14052203161151));
#20396=CARTESIAN_POINT('Ctrl Pts',(0.0260686553993151,1.26108935601086,
1.10727038327973));
#20397=CARTESIAN_POINT('Ctrl Pts',(-0.0421576093699569,1.08053472770428,
1.28727233489076));
#20398=CARTESIAN_POINT('Ctrl Pts',(-0.0242791587196549,1.18019989616608,
1.39987124007464));
#20399=CARTESIAN_POINT('Ctrl Pts',(0.0166569869072257,1.26544208722232,
1.50346488650363));
#20400=CARTESIAN_POINT('Ctrl Pts',(0.16009648734447,1.42418037408903,1.715480776583));
#20401=CARTESIAN_POINT('Ctrl Pts',(0.275079075974333,1.48987049850469,1.81902921434248));
#20402=CARTESIAN_POINT('Ctrl Pts',(0.425598593400272,1.53333167412,1.90869858745619));
#20403=CARTESIAN_POINT('Ctrl Pts',(0.0260686553993151,1.26108935601086,
1.10727038327973));
#20404=CARTESIAN_POINT('Ctrl Pts',(0.0438278133131022,1.34014965076829,
1.17697999301248));
#20405=CARTESIAN_POINT('Ctrl Pts',(0.0765323136032915,1.41611581747019,
1.24430717677953));
#20406=CARTESIAN_POINT('Ctrl Pts',(0.182773095427524,1.55978740991096,1.37795460947454));
#20407=CARTESIAN_POINT('Ctrl Pts',(0.255660077554632,1.62160544971256,1.43952296396723));
#20408=CARTESIAN_POINT('Ctrl Pts',(0.417882684528636,1.71055550747307,1.54471868724301));
#20409=CARTESIAN_POINT('Ctrl Pts',(0.503955443296384,1.74236185427982,1.59041399531286));
#20410=CARTESIAN_POINT('Ctrl Pts',(0.602229799711921,1.76386916735271,1.63615580822897));
#20411=CARTESIAN_POINT('Ctrl Pts',(-0.281756991007075,1.23578335387376,
1.1017328493151));
#20412=CARTESIAN_POINT('Ctrl Pts',(-0.285293785520307,1.50493278576873,
1.32007563441911));
#20413=CARTESIAN_POINT('Ctrl Pts',(-0.13749526484018,1.71461214828354,1.49912049044759));
#20414=CARTESIAN_POINT('Ctrl Pts',(0.161638571033305,1.8648214414182,1.63886741740056));
#20415=CARTESIAN_POINT('Ctrl Pts',(-0.248240087990173,1.20648752589178,
1.13414277848451));
#20416=CARTESIAN_POINT('Ctrl Pts',(-0.246204407588735,1.4681167114295,1.35885799576156));
#20417=CARTESIAN_POINT('Ctrl Pts',(-0.0982540365453086,1.66875380764494,
1.54315303441876));
#20418=CARTESIAN_POINT('Ctrl Pts',(0.195476545731356,1.80862652874333,1.68697274180731));
#20419=CARTESIAN_POINT('Ctrl Pts',(-0.208527189600699,1.16364558145094,
1.1806131496188));
#20420=CARTESIAN_POINT('Ctrl Pts',(-0.200108802601649,1.41464853624076,
1.41450373020722));
#20421=CARTESIAN_POINT('Ctrl Pts',(-0.0532621882672281,1.60356331755514,
1.60633610108347));
#20422=CARTESIAN_POINT('Ctrl Pts',(0.232035965773787,1.73053166984717,1.75602333097544));
#20423=CARTESIAN_POINT('Ctrl Pts',(-0.177813888094451,1.10574232216634,
1.24113368360637));
#20424=CARTESIAN_POINT('Ctrl Pts',(-0.165512243823413,1.34323970181786,
1.48714102989094));
#20425=CARTESIAN_POINT('Ctrl Pts',(-0.0231812731495988,1.5196432848029,
1.68887271819554));
#20426=CARTESIAN_POINT('Ctrl Pts',(0.249170413362428,1.63495516880573,1.84633185797669));
#20427=CARTESIAN_POINT('Ctrl Pts',(-0.172859970247478,1.07870022090367,
1.26846296103996));
#20428=CARTESIAN_POINT('Ctrl Pts',(-0.160752258036383,1.31037084404559,
1.51988605935312));
#20429=CARTESIAN_POINT('Ctrl Pts',(-0.0218314126094571,1.48224938444033,
1.72614171343829));
#20430=CARTESIAN_POINT('Ctrl Pts',(0.243918395495177,1.59461215150754,1.88707489423909));
#20431=CARTESIAN_POINT('Ctrl Pts',(-0.172008888578299,1.06394999292458,
1.28318566992362));
#20432=CARTESIAN_POINT('Ctrl Pts',(-0.160360824547434,1.29249985168946,
1.53754047574671));
#20433=CARTESIAN_POINT('Ctrl Pts',(-0.0235398295887241,1.46236429518571,
1.74612008846831));
#20434=CARTESIAN_POINT('Ctrl Pts',(0.238454096297831,1.57354332341336,1.90892450808845));
#20435=CARTESIAN_POINT('',(-0.171810769270086,1.06762054184321,1.28727233489076));
#20436=CARTESIAN_POINT('Ctrl Pts',(-0.27609248605185,1.23077165948193,1.10727038327973));
#20437=CARTESIAN_POINT('Ctrl Pts',(-0.256045785977569,1.21397173814619,
1.12805083925439));
#20438=CARTESIAN_POINT('Ctrl Pts',(-0.235667011409721,1.19436482287746,
1.15131250789247));
#20439=CARTESIAN_POINT('Ctrl Pts',(-0.206554607000384,1.15844075168706,
1.19194777349537));
#20440=CARTESIAN_POINT('Ctrl Pts',(-0.194102717857879,1.14116749104457,
1.21108489279973));
#20441=CARTESIAN_POINT('Ctrl Pts',(-0.178981360555473,1.10902103082101,
1.24526606650695));
#20442=CARTESIAN_POINT('Ctrl Pts',(-0.173166578774615,1.09145681862821,
1.26352342884102));
#20443=CARTESIAN_POINT('Ctrl Pts',(-0.171810769270086,1.06762054184321,
1.28727233489076));
#20444=CARTESIAN_POINT('Ctrl Pts',(-0.171810769270086,1.06762054184321,
1.28727233489076));
#20445=CARTESIAN_POINT('Ctrl Pts',(-0.166049132983329,1.16871252149279,
1.39987124007464));
#20446=CARTESIAN_POINT('Ctrl Pts',(-0.135662485730195,1.25825944116939,
1.50346488650363));
#20447=CARTESIAN_POINT('Ctrl Pts',(-0.0123561690781438,1.43309732687145,
1.715480776583));
#20448=CARTESIAN_POINT('Ctrl Pts',(0.0938909933754471,1.51213990150266,
1.81902921434248));
#20449=CARTESIAN_POINT('Ctrl Pts',(0.238090659850088,1.57338902476662,1.90869858745619));
#20450=CARTESIAN_POINT('Ctrl Pts',(-0.171810769270086,1.06762054184321,
1.28727233489076));
#20451=CARTESIAN_POINT('Ctrl Pts',(-0.158856141562724,1.29491863831812,
1.54044293163017));
#20452=CARTESIAN_POINT('Ctrl Pts',(-0.0214114678431582,1.46385147967851,
1.74808806329354));
#20453=CARTESIAN_POINT('Ctrl Pts',(0.240523251888612,1.5744190659244,1.91020772988088));
#20454=CARTESIAN_POINT('Ctrl Pts',(-0.128593049303376,1.07192527046357,
1.28727233489076));
#20455=CARTESIAN_POINT('Ctrl Pts',(-0.106557157682628,1.2981540059198,1.54044293163017));
#20456=CARTESIAN_POINT('Ctrl Pts',(0.0373276272898298,1.46116778184124,
1.74808806329354));
#20457=CARTESIAN_POINT('Ctrl Pts',(0.303061305613997,1.56096659822788,1.91020772988088));
#20458=CARTESIAN_POINT('Ctrl Pts',(-0.0853753293366666,1.07622999908393,
1.28727233489076));
#20459=CARTESIAN_POINT('Ctrl Pts',(-0.0542581738025321,1.30138937352148,
1.54044293163017));
#20460=CARTESIAN_POINT('Ctrl Pts',(0.0960667224228169,1.45848408400396,
1.74808806329354));
#20461=CARTESIAN_POINT('Ctrl Pts',(0.365599359339382,1.54751413053135,1.91020772988088));
#20462=CARTESIAN_POINT('Ctrl Pts',(-0.042157609369957,1.08053472770428,
1.28727233489076));
#20463=CARTESIAN_POINT('Ctrl Pts',(-0.00195918992243626,1.30462474112317,
1.54044293163017));
#20464=CARTESIAN_POINT('Ctrl Pts',(0.154805817555805,1.45580038616668,1.74808806329354));
#20465=CARTESIAN_POINT('Ctrl Pts',(0.428137413064766,1.53406166283483,1.91020772988088));
#20466=CARTESIAN_POINT('Ctrl Pts',(-0.171810769270086,1.06762054184321,
1.28727233489076));
#20467=CARTESIAN_POINT('Ctrl Pts',(-0.150205945126615,1.0703931707,1.28796759655004));
#20468=CARTESIAN_POINT('Ctrl Pts',(-0.128560761691045,1.07285457179227,
1.2883190755065));
#20469=CARTESIAN_POINT('Ctrl Pts',(-0.106874449528872,1.07501055311346,
1.288319084765));
#20470=CARTESIAN_POINT('Ctrl Pts',(-0.0853218532357455,1.07715324084587,
1.28831909396641));
#20471=CARTESIAN_POINT('Ctrl Pts',(-0.0637502700203263,1.07899214990169,
1.28797193184368));
#20472=CARTESIAN_POINT('Ctrl Pts',(-0.042157609369957,1.08053472770428,
1.28727233489076));
#20473=CARTESIAN_POINT('Origin',(0.,0.,1.37171309575435));
#20474=CARTESIAN_POINT('',(0.117749801015232,1.25585067703094,1.10727038327973));
#20475=CARTESIAN_POINT('Ctrl Pts',(0.719647344681868,1.71930883511106,1.63615580822897));
#20476=CARTESIAN_POINT('Ctrl Pts',(0.634377380847188,1.70798257074607,1.59808263051822));
#20477=CARTESIAN_POINT('Ctrl Pts',(0.552378154622132,1.68649822169668,1.55687869031203));
#20478=CARTESIAN_POINT('Ctrl Pts',(0.383878819109615,1.61179111914083,1.4528510278119));
#20479=CARTESIAN_POINT('Ctrl Pts',(0.306551362590222,1.55475212125012,1.3904370872311));
#20480=CARTESIAN_POINT('Ctrl Pts',(0.186091644383526,1.41508721860523,1.25222975809873));
#20481=CARTESIAN_POINT('Ctrl Pts',(0.145146699351924,1.33721040532788,1.18062438818012));
#20482=CARTESIAN_POINT('Ctrl Pts',(0.117749801015232,1.25585067703094,1.10727038327973));
#20483=CARTESIAN_POINT('Origin',(0.,0.,1.10727038327973));
#20484=CARTESIAN_POINT('Ctrl Pts',(0.292083537906633,1.03743092372925,1.28318517918604));
#20485=CARTESIAN_POINT('Ctrl Pts',(0.398891247467645,1.23979244918951,1.53750926858099));
#20486=CARTESIAN_POINT('Ctrl Pts',(0.594491629104918,1.33623488367508,1.74606924121325));
#20487=CARTESIAN_POINT('Ctrl Pts',(0.87888468281845,1.32675822718598,1.90886509708282));
#20488=CARTESIAN_POINT('Ctrl Pts',(0.294610685989129,1.05199356151554,1.26845681306972));
#20489=CARTESIAN_POINT('Ctrl Pts',(0.40263140600932,1.25726427409018,1.51984840181957));
#20490=CARTESIAN_POINT('Ctrl Pts',(0.600652305106663,1.35531508433345,1.7260837721201));
#20491=CARTESIAN_POINT('Ctrl Pts',(0.888971417088885,1.34605472186503,1.88700775532557));
#20492=CARTESIAN_POINT('Ctrl Pts',(0.302614092509143,1.07830248703539,1.241120378339));
#20493=CARTESIAN_POINT('Ctrl Pts',(0.413428941810942,1.28869195855348,1.48709498232076));
#20494=CARTESIAN_POINT('Ctrl Pts',(0.616606838701691,1.38909450341185,1.6888059961384));
#20495=CARTESIAN_POINT('Ctrl Pts',(0.912150767476957,1.3795008682383,1.84625490381853));
#20496=CARTESIAN_POINT('Ctrl Pts',(0.339741650892327,1.13234954650476,1.18057861631984));
#20497=CARTESIAN_POINT('Ctrl Pts',(0.460769919763728,1.35241043892922,1.41443334405942));
#20498=CARTESIAN_POINT('Ctrl Pts',(0.677140712937703,1.45460182159639,1.60624291768869));
#20499=CARTESIAN_POINT('Ctrl Pts',(0.989017806729666,1.43888625177221,1.75591740484438));
#20500=CARTESIAN_POINT('Ctrl Pts',(0.384106544865064,1.17040376051198,1.13408778445339));
#20501=CARTESIAN_POINT('Ctrl Pts',(0.516073741815779,1.39633768248717,1.35876508657127));
#20502=CARTESIAN_POINT('Ctrl Pts',(0.744159155535338,1.49702742698244,1.54303391436824));
#20503=CARTESIAN_POINT('Ctrl Pts',(1.06856709212991,1.47227219091281,1.68683916414416));
#20504=CARTESIAN_POINT('Ctrl Pts',(0.420763908606199,1.19569665581666,1.101666983688));
#20505=CARTESIAN_POINT('Ctrl Pts',(0.56137811669726,1.42522258493377,1.31997051162988));
#20506=CARTESIAN_POINT('Ctrl Pts',(0.798253662001981,1.52373714690789,1.49898794576058));
#20507=CARTESIAN_POINT('Ctrl Pts',(1.13139054452036,1.49124034173901,1.63871928608011));
#20508=CARTESIAN_POINT('',(0.293809324770207,1.04067701160391,1.28727233489076));
#20509=CARTESIAN_POINT('',(0.414490807021284,1.19131159212569,1.10727038327973));
#20510=CARTESIAN_POINT('Ctrl Pts',(0.293809324770207,1.04067701160391,1.28727233489076));
#20511=CARTESIAN_POINT('Ctrl Pts',(0.299434836228389,1.07291073821506,1.2547227402422));
#20512=CARTESIAN_POINT('Ctrl Pts',(0.312686039747463,1.09698565606033,1.22803799031295));
#20513=CARTESIAN_POINT('Ctrl Pts',(0.354129853274083,1.14435511150538,1.17079203987282));
#20514=CARTESIAN_POINT('Ctrl Pts',(0.380297147863541,1.1680017368866,1.14052203161296));
#20515=CARTESIAN_POINT('Ctrl Pts',(0.414490807021284,1.19131159212569,1.10727038327973));
#20516=CARTESIAN_POINT('Ctrl Pts',(0.293809324770207,1.04067701160391,1.28727233489076));
#20517=CARTESIAN_POINT('Ctrl Pts',(0.341610972564374,1.12993947443311,1.39987124007464));
#20518=CARTESIAN_POINT('Ctrl Pts',(0.406884846288962,1.19835965101752,1.50346488650363));
#20519=CARTESIAN_POINT('Ctrl Pts',(0.592356746173702,1.30500348982786,1.715480776583));
#20520=CARTESIAN_POINT('Ctrl Pts',(0.722011051157661,1.33194693676576,1.81902921434248));
#20521=CARTESIAN_POINT('Ctrl Pts',(0.878593860895847,1.32676788217082,1.90869858745619));
#20522=CARTESIAN_POINT('Ctrl Pts',(0.414490807021284,1.19131159212569,1.10727038327973));
#20523=CARTESIAN_POINT('Ctrl Pts',(0.455811744539446,1.26101451903382,1.17697999301248));
#20524=CARTESIAN_POINT('Ctrl Pts',(0.510390409161015,1.32315639051141,1.24430717677953));
#20525=CARTESIAN_POINT('Ctrl Pts',(0.655828360684359,1.42696598762934,1.37795460947455));
#20526=CARTESIAN_POINT('Ctrl Pts',(0.744250824847078,1.46323512106126,1.43952296396724));
#20527=CARTESIAN_POINT('Ctrl Pts',(0.926020771798293,1.49770211069237,1.54471868724277));
#20528=CARTESIAN_POINT('Ctrl Pts',(1.01770953159202,1.50135379887064,1.59041399531261));
#20529=CARTESIAN_POINT('Ctrl Pts',(1.11782012388912,1.4914400228729,1.63615580822897));
#20530=CARTESIAN_POINT('Ctrl Pts',(0.114046207919,1.26214138440836,1.10192461715937));
#20531=CARTESIAN_POINT('Ctrl Pts',(0.193872070477572,1.51915795367953,1.32030517702043));
#20532=CARTESIAN_POINT('Ctrl Pts',(0.399215503609646,1.67285198321398,1.49938098964776));
#20533=CARTESIAN_POINT('Ctrl Pts',(0.730076507315222,1.72322347301172,1.63915205504133));
#20534=CARTESIAN_POINT('Ctrl Pts',(0.131128471412264,1.23350917110672,1.12620814253776));
#20535=CARTESIAN_POINT('Ctrl Pts',(0.213229856531408,1.48384440470435,1.3493730700966));
#20536=CARTESIAN_POINT('Ctrl Pts',(0.416549152036918,1.63116936194582,1.53236753871639));
#20537=CARTESIAN_POINT('Ctrl Pts',(0.741153963610066,1.67535851585319,1.67519578767207));
#20538=CARTESIAN_POINT('Ctrl Pts',(0.15432167232943,1.18566161414104,1.16792358645355));
#20539=CARTESIAN_POINT('Ctrl Pts',(0.239112514228604,1.42508536822678,1.39930746388997));
#20540=CARTESIAN_POINT('Ctrl Pts',(0.438352145622179,1.56242925297243,1.58908978141844));
#20541=CARTESIAN_POINT('Ctrl Pts',(0.752201465653619,1.59768412386216,1.73717464481024));
#20542=CARTESIAN_POINT('Ctrl Pts',(0.172598846101516,1.11989042845005,1.22814930406781));
#20543=CARTESIAN_POINT('Ctrl Pts',(0.258281860114563,1.34476711329974,1.47154499595953));
#20544=CARTESIAN_POINT('Ctrl Pts',(0.450170312236601,1.47038505632136,1.67113613169257));
#20545=CARTESIAN_POINT('Ctrl Pts',(0.748265815679387,1.49675459841166,1.82691733765972));
#20546=CARTESIAN_POINT('Ctrl Pts',(0.17018101435307,1.08406383481183,1.26357751389222));
#20547=CARTESIAN_POINT('Ctrl Pts',(0.25382096368873,1.30156053800084,1.51402822523203));
#20548=CARTESIAN_POINT('Ctrl Pts',(0.439852505027491,1.42264323155934,1.71951214242025));
#20549=CARTESIAN_POINT('Ctrl Pts',(0.728627336389052,1.44728013834437,1.87982452105688));
#20550=CARTESIAN_POINT('Ctrl Pts',(0.165188454635723,1.06503024353735,1.28318566992362));
#20551=CARTESIAN_POINT('Ctrl Pts',(0.24689221225484,1.27879462627691,1.53754047574671));
#20552=CARTESIAN_POINT('Ctrl Pts',(0.429507710856696,1.39806529952135,1.74612008846832));
#20553=CARTESIAN_POINT('Ctrl Pts',(0.71303495044129,1.42284226327066,1.90892450808845));
#20554=CARTESIAN_POINT('',(0.166511139289342,1.06845992077163,1.28727233489076));
#20555=CARTESIAN_POINT('Ctrl Pts',(0.117749801015232,1.25585067703094,1.10727038327973));
#20556=CARTESIAN_POINT('Ctrl Pts',(0.13162388455422,1.23367823136719,1.12805083925445));
#20557=CARTESIAN_POINT('Ctrl Pts',(0.144946380875765,1.2087335591704,1.15131250789254));
#20558=CARTESIAN_POINT('Ctrl Pts',(0.161532774289144,1.16557150946378,1.19194777349501));
#20559=CARTESIAN_POINT('Ctrl Pts',(0.168037493511643,1.1452958170147,1.21108489279962));
#20560=CARTESIAN_POINT('Ctrl Pts',(0.172484956391369,1.11004996015782,1.24526606650779));
#20561=CARTESIAN_POINT('Ctrl Pts',(0.172587502434193,1.09154853530949,1.26352342884182));
#20562=CARTESIAN_POINT('Ctrl Pts',(0.166511139289342,1.06845992077163,1.28727233489076));
#20563=CARTESIAN_POINT('Ctrl Pts',(0.166511139289342,1.06845992077163,1.28727233489076));
#20564=CARTESIAN_POINT('Ctrl Pts',(0.203229920731113,1.16282366323453,1.39987124007464));
#20565=CARTESIAN_POINT('Ctrl Pts',(0.259800859583567,1.23859785430383,1.50346488650363));
#20566=CARTESIAN_POINT('Ctrl Pts',(0.431100013478375,1.36677481743678,1.715480776583));
#20567=CARTESIAN_POINT('Ctrl Pts',(0.556572568507924,1.40911659430225,1.81902921434248));
#20568=CARTESIAN_POINT('Ctrl Pts',(0.712641620935351,1.42280782457595,1.90869858745619));
#20569=CARTESIAN_POINT('Ctrl Pts',(0.166511139289342,1.06845992077163,1.28727233489076));
#20570=CARTESIAN_POINT('Ctrl Pts',(0.24907069698643,1.28063005644821,1.54044293163017));
#20571=CARTESIAN_POINT('Ctrl Pts',(0.431991468445894,1.3988219960746,1.74808806329354));
#20572=CARTESIAN_POINT('Ctrl Pts',(0.715273453667735,1.42303573965083,1.91020772988088));
#20573=CARTESIAN_POINT('Ctrl Pts',(0.208943867782964,1.05919895104906,1.28727233489076));
#20574=CARTESIAN_POINT('Ctrl Pts',(0.29980976997318,1.26754579908091,1.54044293163017));
#20575=CARTESIAN_POINT('Ctrl Pts',(0.487026359393917,1.37811826912839,1.74808806329354));
#20576=CARTESIAN_POINT('Ctrl Pts',(0.770593636045173,1.39091636119152,1.91020772988088));
#20577=CARTESIAN_POINT('Ctrl Pts',(0.251376596276585,1.04993798132648,1.28727233489076));
#20578=CARTESIAN_POINT('Ctrl Pts',(0.350548842959931,1.25446154171361,1.54044293163017));
#20579=CARTESIAN_POINT('Ctrl Pts',(0.542061250341939,1.35741454218218,1.74808806329354));
#20580=CARTESIAN_POINT('Ctrl Pts',(0.82591381842261,1.35879698273221,1.91020772988088));
#20581=CARTESIAN_POINT('Ctrl Pts',(0.293809324770207,1.04067701160391,1.28727233489076));
#20582=CARTESIAN_POINT('Ctrl Pts',(0.401287915946682,1.24137728434631,1.54044293163017));
#20583=CARTESIAN_POINT('Ctrl Pts',(0.597096141289962,1.33671081523597,1.74808806329354));
#20584=CARTESIAN_POINT('Ctrl Pts',(0.881234000800047,1.3266776042729,1.91020772988088));
#20585=CARTESIAN_POINT('Ctrl Pts',(0.166511139289342,1.06845992077163,1.28727233489076));
#20586=CARTESIAN_POINT('Ctrl Pts',(0.187915337510245,1.06442058969234,1.28796759655004));
#20587=CARTESIAN_POINT('Ctrl Pts',(0.209261745030533,1.06007279171241,1.2883190755065));
#20588=CARTESIAN_POINT('Ctrl Pts',(0.230552888394581,1.05542181279351,1.288319084765));
#20589=CARTESIAN_POINT('Ctrl Pts',(0.251712752465187,1.05079951139632,1.28831909396641));
#20590=CARTESIAN_POINT('Ctrl Pts',(0.272796801398367,1.04588243202759,1.28797193184368));
#20591=CARTESIAN_POINT('Ctrl Pts',(0.293809324770207,1.04067701160391,1.28727233489076));
#20592=CARTESIAN_POINT('Origin',(0.,0.,1.37171309575435));
#20593=CARTESIAN_POINT('',(0.500065917147839,1.15799828028598,1.10727038327973));
#20594=CARTESIAN_POINT('Ctrl Pts',(1.21572094522251,1.4127766116927,1.63615580822897));
#20595=CARTESIAN_POINT('Ctrl Pts',(1.13112438230172,1.42835456209775,1.59808263051822));
#20596=CARTESIAN_POINT('Ctrl Pts',(1.04649945489987,1.4332608863651,1.55687869031203));
#20597=CARTESIAN_POINT('Ctrl Pts',(0.863161299579016,1.41427936788009,1.4528510278119));
#20598=CARTESIAN_POINT('Ctrl Pts',(0.771992498477368,1.38392755544946,1.3904370872311));
#20599=CARTESIAN_POINT('Ctrl Pts',(0.614269670090823,1.2883224397548,1.25222975809873));
#20600=CARTESIAN_POINT('Ctrl Pts',(0.551263454538705,1.22690987286759,1.18062438818012));
#20601=CARTESIAN_POINT('Ctrl Pts',(0.500065917147839,1.15799828028598,1.10727038327973));
#20602=CARTESIAN_POINT('Origin',(0.,0.,1.10727038327973));
#20603=CARTESIAN_POINT('Ctrl Pts',(0.598371737951084,0.896396663228496,
1.28318517918604));
#20604=CARTESIAN_POINT('Ctrl Pts',(0.762485056494508,1.05584851328029,1.537509268581));
#20605=CARTESIAN_POINT('Ctrl Pts',(0.9783144252754,1.08712687701302,1.74606924121326));
#20606=CARTESIAN_POINT('Ctrl Pts',(1.24585984429376,0.99023175442669,1.90886509708284));
#20607=CARTESIAN_POINT('Ctrl Pts',(0.605275301161475,0.909465623084801,
1.26845681306972));
#20608=CARTESIAN_POINT('Ctrl Pts',(0.771441249464595,1.07130943365261,1.51984840181958));
#20609=CARTESIAN_POINT('Ctrl Pts',(0.990069682591161,1.10336947260001,1.72608377212012));
#20610=CARTESIAN_POINT('Ctrl Pts',(1.26141584343748,1.00546683912554,1.88700775532559));
#20611=CARTESIAN_POINT('Ctrl Pts',(0.621016981690702,0.932013737380381,
1.24112031232197));
#20612=CARTESIAN_POINT('Ctrl Pts',(0.791422088358104,1.09786234356421,1.48709491630374));
#20613=CARTESIAN_POINT('Ctrl Pts',(1.01568188386469,1.13056538342229,1.68880590632087));
#20614=CARTESIAN_POINT('Ctrl Pts',(1.29379626687143,1.03011319759961,1.846254814001));
#20615=CARTESIAN_POINT('Ctrl Pts',(0.673028944353636,0.971942506168049,
1.180578495595));
#20616=CARTESIAN_POINT('Ctrl Pts',(0.856136223676185,1.14383306000902,1.41443322333459));
#20617=CARTESIAN_POINT('Ctrl Pts',(1.09349602729721,1.17416051125987,1.60624275382306));
#20618=CARTESIAN_POINT('Ctrl Pts',(1.38525239147931,1.06283879403329,1.75591724097875));
#20619=CARTESIAN_POINT('Ctrl Pts',(0.726981684724074,0.994424673117319,
1.1340877844534));
#20620=CARTESIAN_POINT('Ctrl Pts',(0.922307368817381,1.16852049530615,1.35876508657128));
#20621=CARTESIAN_POINT('Ctrl Pts',(1.17034433001557,1.1937998639241,1.54303391436826));
#20622=CARTESIAN_POINT('Ctrl Pts',(1.47122482340644,1.0700086698298,1.68683916414419));
#20623=CARTESIAN_POINT('Ctrl Pts',(0.769660843866374,1.00715189764781,1.101666983688));
#20624=CARTESIAN_POINT('Ctrl Pts',(0.974320315501952,1.18199184824263,1.31997051162989));
#20625=CARTESIAN_POINT('Ctrl Pts',(1.23004502025839,1.20248619530708,1.4989879457606));
#20626=CARTESIAN_POINT('Ctrl Pts',(1.53683495813569,1.06863493884117,1.63871928608014));
#20627=CARTESIAN_POINT('',(0.601016155111926,0.89895057878464,1.28727233489076));
#20628=CARTESIAN_POINT('',(0.762339710524743,1.00491994924733,1.10727038327973));
#20629=CARTESIAN_POINT('Ctrl Pts',(0.601016155111926,0.89895057878464,1.28727233489076));
#20630=CARTESIAN_POINT('Ctrl Pts',(0.616327103756364,0.927868295879574,
1.25472274024271));
#20631=CARTESIAN_POINT('Ctrl Pts',(0.636369305963446,0.946670056291957,
1.2280379903142));
#20632=CARTESIAN_POINT('Ctrl Pts',(0.690422681622986,0.978914242873978,
1.1707920398759));
#20633=CARTESIAN_POINT('Ctrl Pts',(0.722616466757832,0.993317381306835,
1.14052203161603));
#20634=CARTESIAN_POINT('Ctrl Pts',(0.762339710524743,1.00491994924733,1.10727038327973));
#20635=CARTESIAN_POINT('Ctrl Pts',(0.601016155111926,0.89895057878464,1.28727233489076));
#20636=CARTESIAN_POINT('Ctrl Pts',(0.674061841710201,0.969072704191387,
1.39987124007464));
#20637=CARTESIAN_POINT('Ctrl Pts',(0.757283981982513,1.01397342270847,1.50346488650363));
#20638=CARTESIAN_POINT('Ctrl Pts',(0.966632999495317,1.05808377148838,1.715480776583));
#20639=CARTESIAN_POINT('Ctrl Pts',(1.09826755410688,1.04364312863621,1.81902921434248));
#20640=CARTESIAN_POINT('Ctrl Pts',(1.24558623976355,0.990330805779365,1.90869858745619));
#20641=CARTESIAN_POINT('Ctrl Pts',(0.762339710524743,1.00491994924733,1.10727038327973));
#20642=CARTESIAN_POINT('Ctrl Pts',(0.823177646383101,1.05844250017153,1.17697999301248));
#20643=CARTESIAN_POINT('Ctrl Pts',(0.894287935370968,1.10067719707671,1.24430717677952));
#20644=CARTESIAN_POINT('Ctrl Pts',(1.06468657657251,1.15446319222191,1.37795460947454));
#20645=CARTESIAN_POINT('Ctrl Pts',(1.15998911590306,1.16163314380192,1.43952296396723));
#20646=CARTESIAN_POINT('Ctrl Pts',(1.34351349395885,1.13824319621308,1.54471868724291));
#20647=CARTESIAN_POINT('Ctrl Pts',(1.43184312013697,1.11338277308098,1.59041399531275));
#20648=CARTESIAN_POINT('Ctrl Pts',(1.5239904260293,1.07301833748062,1.63615580822897));
#20649=CARTESIAN_POINT('Ctrl Pts',(0.498487526286222,1.16512557173636,1.10192461715937));
#20650=CARTESIAN_POINT('Ctrl Pts',(0.653828920782169,1.38489530661629,1.32030517702043));
#20651=CARTESIAN_POINT('Ctrl Pts',(0.896616198000952,1.46761240439959,1.49938098964775));
#20652=CARTESIAN_POINT('Ctrl Pts',(1.22684935794257,1.41327686508625,1.63915205504133));
#20653=CARTESIAN_POINT('Ctrl Pts',(0.508352002968308,1.12177948805866,1.13430265099724));
#20654=CARTESIAN_POINT('Ctrl Pts',(0.663777262634273,1.33220260121988,1.35904945381843));
#20655=CARTESIAN_POINT('Ctrl Pts',(0.901376560628895,1.40752683379662,1.54337045304295));
#20656=CARTESIAN_POINT('Ctrl Pts',(1.22117496033747,1.34801632954311,1.68721036521565));
#20657=CARTESIAN_POINT('Ctrl Pts',(0.515271529296697,1.06384346101581,1.18072933479299));
#20658=CARTESIAN_POINT('Ctrl Pts',(0.669611793063643,1.26193419272815,1.41464220917676));
#20659=CARTESIAN_POINT('Ctrl Pts',(0.899433473713048,1.32843484168648,1.60649429051817));
#20660=CARTESIAN_POINT('Ctrl Pts',(1.20484145605229,1.26345277789772,1.75619579796004));
#20661=CARTESIAN_POINT('Ctrl Pts',(0.506068760645491,0.999035931036402,
1.24118020602736));
#20662=CARTESIAN_POINT('Ctrl Pts',(0.655613152504221,1.18393656063858,1.48719644285888));
#20663=CARTESIAN_POINT('Ctrl Pts',(0.874439260092139,1.2429854225176,1.68893627188731));
#20664=CARTESIAN_POINT('Ctrl Pts',(1.1625431884408,1.17619191287087,1.84640112540367));
#20665=CARTESIAN_POINT('Ctrl Pts',(0.494188433189343,0.974277339819634,
1.26847955290007));
#20666=CARTESIAN_POINT('Ctrl Pts',(0.640153731237153,1.15458357076034,1.51990601315847));
#20667=CARTESIAN_POINT('Ctrl Pts',(0.853567659762739,1.21197995173255,1.72616419407531));
#20668=CARTESIAN_POINT('Ctrl Pts',(1.13460469485221,1.14668110494347,1.88709951781477));
#20669=CARTESIAN_POINT('Ctrl Pts',(0.486216000974361,0.961857913410637,
1.28318566992362));
#20670=CARTESIAN_POINT('Ctrl Pts',(0.629977719122416,1.13991207295831,1.5375404757467));
#20671=CARTESIAN_POINT('Ctrl Pts',(0.840512044007267,1.19691393144611,1.74612008846831));
#20672=CARTESIAN_POINT('Ctrl Pts',(1.11781897562892,1.13286348887405,1.90892450808844));
#20673=CARTESIAN_POINT('',(0.488533777383804,0.964710998256926,1.28727233489076));
#20674=CARTESIAN_POINT('Ctrl Pts',(0.500065917147839,1.15799828028598,1.10727038327973));
#20675=CARTESIAN_POINT('Ctrl Pts',(0.506409292188269,1.13262370376034,1.12805083925446));
#20676=CARTESIAN_POINT('Ctrl Pts',(0.511371411500265,1.10478303294993,1.1513125078925));
#20677=CARTESIAN_POINT('Ctrl Pts',(0.513808202166489,1.05860800687968,1.19194777349496));
#20678=CARTESIAN_POINT('Ctrl Pts',(0.513729024230259,1.03731460867027,1.2110848927995));
#20679=CARTESIAN_POINT('Ctrl Pts',(0.507067244033061,1.00241946522318,1.24526606650694));
#20680=CARTESIAN_POINT('Ctrl Pts',(0.501447516417269,0.984791876090262,
1.26352342884106));
#20681=CARTESIAN_POINT('Ctrl Pts',(0.488533777383804,0.964710998256926,
1.28727233489076));
#20682=CARTESIAN_POINT('Ctrl Pts',(0.488533777383804,0.964710998256926,
1.28727233489076));
#20683=CARTESIAN_POINT('Ctrl Pts',(0.552615413818275,1.04310952295002,1.39987124007464));
#20684=CARTESIAN_POINT('Ctrl Pts',(0.629833086622262,1.09769367964031,1.50346488650363));
#20685=CARTESIAN_POINT('Ctrl Pts',(0.832357123065218,1.16666286599128,1.715480776583));
#20686=CARTESIAN_POINT('Ctrl Pts',(0.964772942765737,1.16815913695893,1.81902921434248));
#20687=CARTESIAN_POINT('Ctrl Pts',(1.11743425489732,1.13295228123076,1.90869858745619));
#20688=CARTESIAN_POINT('Ctrl Pts',(0.488533777383804,0.964710998256926,
1.28727233489076));
#20689=CARTESIAN_POINT('Ctrl Pts',(0.632616760336964,1.14098448197888,1.54044293163017));
#20690=CARTESIAN_POINT('Ctrl Pts',(0.843108069941918,1.19686606932897,1.74808806329354));
#20691=CARTESIAN_POINT('Ctrl Pts',(1.12000770619867,1.13235576030722,1.91020772988088));
#20692=CARTESIAN_POINT('Ctrl Pts',(0.526027903293178,0.94279085843283,1.28727233489076));
#20693=CARTESIAN_POINT('Ctrl Pts',(0.676829228446517,1.11286137791709,1.54044293163017));
#20694=CARTESIAN_POINT('Ctrl Pts',(0.889051558128351,1.16016893831867,1.74808806329354));
#20695=CARTESIAN_POINT('Ctrl Pts',(1.16269489233868,1.08471353963759,1.91020772988088));
#20696=CARTESIAN_POINT('Ctrl Pts',(0.563522029202552,0.920870718608735,
1.28727233489076));
#20697=CARTESIAN_POINT('Ctrl Pts',(0.72104169655607,1.0847382738553,1.54044293163017));
#20698=CARTESIAN_POINT('Ctrl Pts',(0.934995046314783,1.12347180730837,1.74808806329354));
#20699=CARTESIAN_POINT('Ctrl Pts',(1.20538207847869,1.03707131896797,1.91020772988088));
#20700=CARTESIAN_POINT('Ctrl Pts',(0.601016155111926,0.89895057878464,1.28727233489076));
#20701=CARTESIAN_POINT('Ctrl Pts',(0.765254164665624,1.05661516979351,1.54044293163017));
#20702=CARTESIAN_POINT('Ctrl Pts',(0.980938534501216,1.08677467629807,1.74808806329354));
#20703=CARTESIAN_POINT('Ctrl Pts',(1.2480692646187,0.989429098298345,1.91020772988088));
#20704=CARTESIAN_POINT('Ctrl Pts',(0.488533777383804,0.964710998256926,
1.28727233489076));
#20705=CARTESIAN_POINT('Ctrl Pts',(0.507642157628461,0.95425510511126,1.28796759655004));
#20706=CARTESIAN_POINT('Ctrl Pts',(0.526600254136213,0.943523700818289,
1.2883190755065));
#20707=CARTESIAN_POINT('Ctrl Pts',(0.545412103245543,0.932521031881151,
1.288319084765));
#20708=CARTESIAN_POINT('Ctrl Pts',(0.564107960168948,0.921586204420606,
1.28831909396641));
#20709=CARTESIAN_POINT('Ctrl Pts',(0.582640621209095,0.910394454615255,
1.28797193184368));
#20710=CARTESIAN_POINT('Ctrl Pts',(0.601016155111926,0.89895057878464,1.28727233489076));
#20711=CARTESIAN_POINT('Origin',(0.,0.,1.37171309575435));
#20712=CARTESIAN_POINT('',(0.833432097145896,0.946792943618189,1.10727038327973));
#20713=CARTESIAN_POINT('Ctrl Pts',(1.59279130921887,0.967951970128403,1.63615580822897));
#20714=CARTESIAN_POINT('Ctrl Pts',(1.51714904820957,1.00890925697988,1.59808263051822));
#20715=CARTESIAN_POINT('Ctrl Pts',(1.43818209714157,1.03972598936032,1.55687869031203));
#20716=CARTESIAN_POINT('Ctrl Pts',(1.25795153804723,1.07832809822746,1.45285102781191));
#20717=CARTESIAN_POINT('Ctrl Pts',(1.16186562982555,1.07763451813115,1.39043708723111));
#20718=CARTESIAN_POINT('Ctrl Pts',(0.982318700621182,1.03544768423092,1.25222975809873));
#20719=CARTESIAN_POINT('Ctrl Pts',(0.903418701916906,0.996510853667278,
1.18062438818012));
#20720=CARTESIAN_POINT('Ctrl Pts',(0.833432097145897,0.946792943618189,
1.10727038327973));
#20721=CARTESIAN_POINT('Origin',(0.,0.,1.10727038327973));
#20722=CARTESIAN_POINT('Ctrl Pts',(0.846087143183836,0.667616851768136,
1.28318517918604));
#20723=CARTESIAN_POINT('Ctrl Pts',(1.05144151564591,0.768550768362022,1.53750926858099));
#20724=CARTESIAN_POINT('Ctrl Pts',(1.2663729891825,0.731603317170575,1.74606924121326));
#20725=CARTESIAN_POINT('Ctrl Pts',(1.4908815637936,0.556774498193796,1.90886509708283));
#20726=CARTESIAN_POINT('Ctrl Pts',(0.856691352655137,0.677912852846922,
1.26845681306972));
#20727=CARTESIAN_POINT('Ctrl Pts',(1.06473704847503,0.780487361597376,1.51984840181957));
#20728=CARTESIAN_POINT('Ctrl Pts',(1.28257214132252,0.743418369261302,1.72608377212011));
#20729=CARTESIAN_POINT('Ctrl Pts',(1.51038409822941,0.56645685667305,1.88700775532558));
#20730=CARTESIAN_POINT('Ctrl Pts',(0.878631748253099,0.694492950134685,
1.24111924840996));
#20731=CARTESIAN_POINT('Ctrl Pts',(1.0919466731633,0.799566273875776,1.48709385239173));
#20732=CARTESIAN_POINT('Ctrl Pts',(1.31533666464122,0.761367941758637,1.68880445881716));
#20733=CARTESIAN_POINT('Ctrl Pts',(1.54879772833386,0.579890165126711,1.84625336649728));
#20734=CARTESIAN_POINT('Ctrl Pts',(0.940438249469778,0.716394511678359,
1.18057655035131));
#20735=CARTESIAN_POINT('Ctrl Pts',(1.16770072295995,0.823288881893969,1.4144312780909));
#20736=CARTESIAN_POINT('Ctrl Pts',(1.40281580396031,0.778782224872496,1.60624011348192));
#20737=CARTESIAN_POINT('Ctrl Pts',(1.64589229282025,0.582751305549679,1.75591460063761));
#20738=CARTESIAN_POINT('Ctrl Pts',(0.998694792103065,0.72110437015383,1.1340877844534));
#20739=CARTESIAN_POINT('Ctrl Pts',(1.23825912446584,0.82632038048354,1.35876508657128));
#20740=CARTESIAN_POINT('Ctrl Pts',(1.48196804720543,0.773714852492098,1.54303391436825));
#20741=CARTESIAN_POINT('Ctrl Pts',(1.7298688183418,0.563005244955071,1.68683916414418));
#20742=CARTESIAN_POINT('Ctrl Pts',(1.0432180131865,0.720020094497306,1.101666983688));
#20743=CARTESIAN_POINT('Ctrl Pts',(1.29188925333651,0.823059514024041,1.31997051162989));
#20744=CARTESIAN_POINT('Ctrl Pts',(1.54143100170431,0.76352751669565,1.4989879457606));
#20745=CARTESIAN_POINT('Ctrl Pts',(1.79184325828988,0.541424102512133,1.63871928608013));
#20746=CARTESIAN_POINT('',(0.849391336665505,0.669228599956957,1.28727233489076));
#20747=CARTESIAN_POINT('',(1.03556549162895,0.720159740047643,1.10727038327973));
#20748=CARTESIAN_POINT('Ctrl Pts',(0.849391336665505,0.669228599956957,
1.28727233489076));
#20749=CARTESIAN_POINT('Ctrl Pts',(0.872888980165507,0.691999639905522,
1.25472274024245));
#20750=CARTESIAN_POINT('Ctrl Pts',(0.897760310667753,0.703687795576912,
1.22803799031335));
#20751=CARTESIAN_POINT('Ctrl Pts',(0.959132127441248,0.717650427656427,
1.17079203987406));
#20752=CARTESIAN_POINT('Ctrl Pts',(0.994201051126515,0.721400199597683,
1.14052203161404));
#20753=CARTESIAN_POINT('Ctrl Pts',(1.03556549162895,0.720159740047643,1.10727038327973));
#20754=CARTESIAN_POINT('Ctrl Pts',(0.849391336665505,0.669228599956957,
1.28727233489076));
#20755=CARTESIAN_POINT('Ctrl Pts',(0.940530841324424,0.713346345736856,
1.39987124007464));
#20756=CARTESIAN_POINT('Ctrl Pts',(1.03355488521186,0.73033241101646,1.50346488650363));
#20757=CARTESIAN_POINT('Ctrl Pts',(1.2462884798982,0.707591441492496,1.715480776583));
#20758=CARTESIAN_POINT('Ctrl Pts',(1.36701797678012,0.653180259586497,1.81902921434248));
#20759=CARTESIAN_POINT('Ctrl Pts',(1.49065195897357,0.556953250077769,1.90869858745619));
#20760=CARTESIAN_POINT('Ctrl Pts',(1.03556549162895,0.720159740047643,1.10727038327973));
#20761=CARTESIAN_POINT('Ctrl Pts',(1.10996518478287,0.752262754789917,1.17697999301248));
#20762=CARTESIAN_POINT('Ctrl Pts',(1.19064632759639,0.77045605072318,1.24430717677953));
#20763=CARTESIAN_POINT('Ctrl Pts',(1.3693258522382,0.768953495941755,1.37795460947454));
#20764=CARTESIAN_POINT('Ctrl Pts',(1.46217959017505,0.746322420853228,1.43952296396723));
#20765=CARTESIAN_POINT('Ctrl Pts',(1.62949375452144,0.667365107081762,1.54471868724285));
#20766=CARTESIAN_POINT('Ctrl Pts',(1.70581792784489,0.616426084068337,1.5904139953127));
#20767=CARTESIAN_POINT('Ctrl Pts',(1.78098192700405,0.549562141057365,1.63615580822897));
#20768=CARTESIAN_POINT('Ctrl Pts',(0.834133412413726,0.954059150195613,
1.10192461715937));
#20769=CARTESIAN_POINT('Ctrl Pts',(1.04978444082665,1.11506945780848,1.32030517702044));
#20770=CARTESIAN_POINT('Ctrl Pts',(1.30624985183956,1.11871269798568,1.49938098964776));
#20771=CARTESIAN_POINT('Ctrl Pts',(1.60352964545243,0.964988870727209,1.63915205504134));
#20772=CARTESIAN_POINT('Ctrl Pts',(0.831123661162973,0.920854500490908,
1.12620814253777));
#20773=CARTESIAN_POINT('Ctrl Pts',(1.04468843542397,1.0751219753964,1.34937307009661));
#20774=CARTESIAN_POINT('Ctrl Pts',(1.29577263793342,1.07480228609568,1.5323675387164));
#20775=CARTESIAN_POINT('Ctrl Pts',(1.58435717993001,0.919754141507906,1.67519578767208));
#20776=CARTESIAN_POINT('Ctrl Pts',(0.821762669862007,0.868512346714967,
1.16792406090532));
#20777=CARTESIAN_POINT('Ctrl Pts',(1.0310896536259,1.01237142622958,1.39930793834175));
#20778=CARTESIAN_POINT('Ctrl Pts',(1.27300639515449,1.00637513236489,1.589090429871));
#20779=CARTESIAN_POINT('Ctrl Pts',(1.54763812191341,0.850420920292676,1.7371752932628));
#20780=CARTESIAN_POINT('Ctrl Pts',(0.79788991722713,0.804559127620147,1.22814985715448));
#20781=CARTESIAN_POINT('Ctrl Pts',(0.999388130632025,0.93612497529341,1.4715455490462));
#20782=CARTESIAN_POINT('Ctrl Pts',(1.22846526028813,0.924963031592628,1.67113688711451));
#20783=CARTESIAN_POINT('Ctrl Pts',(1.48512921647049,0.771080298579199,1.82691809308167));
#20784=CARTESIAN_POINT('Ctrl Pts',(0.774876067377614,0.776996174893135,
1.26357751389222));
#20785=CARTESIAN_POINT('Ctrl Pts',(0.97038356235556,0.903792375271581,1.51402822523203));
#20786=CARTESIAN_POINT('Ctrl Pts',(1.19205686236993,0.892403735624943,1.71951214242026));
#20787=CARTESIAN_POINT('Ctrl Pts',(1.44016181895954,0.742597824795289,1.87982452105689));
#20788=CARTESIAN_POINT('Ctrl Pts',(0.75964933747155,0.764532229061143,1.28318566992362));
#20789=CARTESIAN_POINT('Ctrl Pts',(0.951396617529429,0.889446983704126,
1.53754047574671));
#20790=CARTESIAN_POINT('Ctrl Pts',(1.16924120209866,0.878600288371208,1.74612008846832));
#20791=CARTESIAN_POINT('Ctrl Pts',(1.41318309117925,0.731992143062389,1.90892450808845));
#20792=CARTESIAN_POINT('',(0.762735325532963,0.766529441696069,1.28727233489076));
#20793=CARTESIAN_POINT('Ctrl Pts',(0.833432097145897,0.946792943618189,
1.10727038327973));
#20794=CARTESIAN_POINT('Ctrl Pts',(0.831623829941911,0.920700076576089,
1.12805083925443));
#20795=CARTESIAN_POINT('Ctrl Pts',(0.827739845433,0.892688645988255,1.15131250789251));
#20796=CARTESIAN_POINT('Ctrl Pts',(0.815788503303407,0.848020576825928,
1.19194777349545));
#20797=CARTESIAN_POINT('Ctrl Pts',(0.809133178696474,0.827793819032885,
1.21108489279985));
#20798=CARTESIAN_POINT('Ctrl Pts',(0.792014256883229,0.796665168763711,
1.24526606650783));
#20799=CARTESIAN_POINT('Ctrl Pts',(0.781222353702368,0.78163692658966,1.2635234288418));
#20800=CARTESIAN_POINT('Ctrl Pts',(0.762735325532963,0.766529441696069,
1.28727233489076));
#20801=CARTESIAN_POINT('Ctrl Pts',(0.762735325532963,0.766529441696069,
1.28727233489076));
#20802=CARTESIAN_POINT('Ctrl Pts',(0.847907059902912,0.821288554787752,
1.39987124007464));
#20803=CARTESIAN_POINT('Ctrl Pts',(0.938212862837218,0.849339599532016,
1.50346488650363));
#20804=CARTESIAN_POINT('Ctrl Pts',(1.15213731807335,0.852349824604395,1.715480776583));
#20805=CARTESIAN_POINT('Ctrl Pts',(1.27853461941729,0.812854124246773,1.81902921434248));
#20806=CARTESIAN_POINT('Ctrl Pts',(1.41284463836769,0.732195474855992,1.90869858745619));
#20807=CARTESIAN_POINT('Ctrl Pts',(0.762735325532963,0.766529441696069,
1.28727233489076));
#20808=CARTESIAN_POINT('Ctrl Pts',(0.954237887485568,0.889651396707116,
1.54044293163017));
#20809=CARTESIAN_POINT('Ctrl Pts',(1.17169537927269,0.877752552661174,1.74808806329354));
#20810=CARTESIAN_POINT('Ctrl Pts',(1.41510780089433,0.730832909558243,1.91020772988088));
#20811=CARTESIAN_POINT('Ctrl Pts',(0.791620662577143,0.734095827783032,
1.28727233489076));
#20812=CARTESIAN_POINT('Ctrl Pts',(0.987595926292982,0.849242331321592,
1.54044293163017));
#20813=CARTESIAN_POINT('Ctrl Pts',(1.20405019596674,0.828654188454019,1.74808806329354));
#20814=CARTESIAN_POINT('Ctrl Pts',(1.44098347159841,0.672331399180314,1.91020772988088));
#20815=CARTESIAN_POINT('Ctrl Pts',(0.820505999621324,0.701662213869994,
1.28727233489076));
#20816=CARTESIAN_POINT('Ctrl Pts',(1.0209539651004,0.808833265936067,1.54044293163017));
#20817=CARTESIAN_POINT('Ctrl Pts',(1.23640501266079,0.779555824246864,1.74808806329354));
#20818=CARTESIAN_POINT('Ctrl Pts',(1.4668591423025,0.613829888802385,1.91020772988088));
#20819=CARTESIAN_POINT('Ctrl Pts',(0.849391336665505,0.669228599956957,
1.28727233489076));
#20820=CARTESIAN_POINT('Ctrl Pts',(1.05431200390781,0.768424200550542,1.54044293163017));
#20821=CARTESIAN_POINT('Ctrl Pts',(1.26875982935484,0.730457460039708,1.74808806329354));
#20822=CARTESIAN_POINT('Ctrl Pts',(1.49273481300659,0.555328378424457,1.91020772988088));
#20823=CARTESIAN_POINT('Ctrl Pts',(0.762735325532963,0.766529441696069,
1.28727233489076));
#20824=CARTESIAN_POINT('Ctrl Pts',(0.777677426407088,0.750680482155644,
1.28796759655004));
#20825=CARTESIAN_POINT('Ctrl Pts',(0.792391461327313,0.734615936171909,
1.2883190755065));
#20826=CARTESIAN_POINT('Ctrl Pts',(0.806882581321256,0.718338595112193,
1.288319084765));
#20827=CARTESIAN_POINT('Ctrl Pts',(0.82128435036013,0.702161618687529,1.28831909396641));
#20828=CARTESIAN_POINT('Ctrl Pts',(0.835451517520018,0.685790724893994,
1.28797193184368));
#20829=CARTESIAN_POINT('Ctrl Pts',(0.849391336665505,0.669228599956957,
1.28727233489076));
#20830=CARTESIAN_POINT('Origin',(0.,0.,1.37171309575435));
#20831=CARTESIAN_POINT('',(1.08521613661244,0.642908916934715,1.10727038327973));
#20832=CARTESIAN_POINT('Ctrl Pts',(1.81394816223928,0.428377445609997,1.63615580822897));
#20833=CARTESIAN_POINT('Ctrl Pts',(1.75466459467969,0.490704884304684,1.59808263051822));
#20834=CARTESIAN_POINT('Ctrl Pts',(1.68908545531116,0.544415468320014,1.55687869031203));
#20835=CARTESIAN_POINT('Ctrl Pts',(1.52960471530762,0.636822561166699,1.4528510278119));
#20836=CARTESIAN_POINT('Ctrl Pts',(1.43800725813253,0.665855105856973,1.39043708723109));
#20837=CARTESIAN_POINT('Ctrl Pts',(1.25421153251789,0.681216094986277,1.25222975809873));
#20838=CARTESIAN_POINT('Ctrl Pts',(1.16714103226326,0.668566409010631,1.18062438818012));
#20839=CARTESIAN_POINT('Ctrl Pts',(1.08521613661244,0.642908916934714,1.10727038327973));
#20840=CARTESIAN_POINT('Origin',(0.,0.,1.10727038327973));
#20841=CARTESIAN_POINT('Ctrl Pts',(1.08812850838495,0.649602771712747,1.10192461715937));
#20842=CARTESIAN_POINT('Ctrl Pts',(1.34297974552472,0.736092841324622,1.32030517702043));
#20843=CARTESIAN_POINT('Ctrl Pts',(1.58801866900219,0.660305598163242,1.49938098964775));
#20844=CARTESIAN_POINT('Ctrl Pts',(1.82324527881736,0.422241042228606,1.63915205504132));
#20845=CARTESIAN_POINT('Ctrl Pts',(1.07063084893098,0.608736859462564,1.13430265099723));
#20846=CARTESIAN_POINT('Ctrl Pts',(1.32005612801352,0.687616058553887,1.35904945381841));
#20847=CARTESIAN_POINT('Ctrl Pts',(1.55655247099158,0.608897279480441,1.54337045304294));
#20848=CARTESIAN_POINT('Ctrl Pts',(1.78029541437302,0.37277948714011,1.68721036521563));
#20849=CARTESIAN_POINT('Ctrl Pts',(1.04217626136028,0.557802714124105,1.18072639205178));
#20850=CARTESIAN_POINT('Ctrl Pts',(1.28347496838039,0.62734255163042,1.41463926643554));
#20851=CARTESIAN_POINT('Ctrl Pts',(1.50849481334977,0.546058002751389,1.6064902962218));
#20852=CARTESIAN_POINT('Ctrl Pts',(1.71737956252142,0.313972100865329,1.75619180366366));
#20853=CARTESIAN_POINT('Ctrl Pts',(0.996637718803135,0.510779237881579,
1.24117859886916));
#20854=CARTESIAN_POINT('Ctrl Pts',(1.22630353645006,0.572467001402756,1.48719483570068));
#20855=CARTESIAN_POINT('Ctrl Pts',(1.43804667102142,0.491616133252199,1.68893408523068));
#20856=CARTESIAN_POINT('Ctrl Pts',(1.63186740528246,0.268235808623187,1.84639893874703));
#20857=CARTESIAN_POINT('Ctrl Pts',(0.972472692862429,0.497730252266281,
1.26847955290007));
#20858=CARTESIAN_POINT('Ctrl Pts',(1.1965424430155,0.557804807750029,1.51990601315847));
#20859=CARTESIAN_POINT('Ctrl Pts',(1.40293468429944,0.478797895551027,1.7261641940753));
#20860=CARTESIAN_POINT('Ctrl Pts',(1.59191672260124,0.260780594211983,1.88709951781476));
#20861=CARTESIAN_POINT('Ctrl Pts',(0.958722904028867,0.49236880332188,1.28318566992362));
#20862=CARTESIAN_POINT('Ctrl Pts',(1.17968618624263,0.55191662654344,1.5375404757467));
#20863=CARTESIAN_POINT('Ctrl Pts',(1.38351688474613,0.474283127502366,1.7461200884683));
#20864=CARTESIAN_POINT('Ctrl Pts',(1.57021499953935,0.259468306198656,1.90892450808844));
#20865=CARTESIAN_POINT('',(0.962275025729455,0.493314642657339,1.28727233489076));
#20866=CARTESIAN_POINT('Ctrl Pts',(0.962275025729455,0.493314642657339,
1.28727233489076));
#20867=CARTESIAN_POINT('Ctrl Pts',(1.06019965524839,0.519074140629024,1.39987124007464));
#20868=CARTESIAN_POINT('Ctrl Pts',(1.15475382712427,0.517846241724568,1.50346488650363));
#20869=CARTESIAN_POINT('Ctrl Pts',(1.35913828497575,0.454602843714802,1.715480776583));
#20870=CARTESIAN_POINT('Ctrl Pts',(1.46714441944577,0.377981286365636,1.81902921434248));
#20871=CARTESIAN_POINT('Ctrl Pts',(1.5699559447672,0.259766273896473,1.90869858745619));
#20872=CARTESIAN_POINT('Ctrl Pts',(1.08521613661244,0.642908916934714,1.10727038327973));
#20873=CARTESIAN_POINT('Ctrl Pts',(1.0754332329569,0.618651911001869,1.12805083925446));
#20874=CARTESIAN_POINT('Ctrl Pts',(1.06308333609211,0.593211674629706,1.15131250789255));
#20875=CARTESIAN_POINT('Ctrl Pts',(1.03791374180399,0.554422984205844,1.19194777349584));
#20876=CARTESIAN_POINT('Ctrl Pts',(1.02533374006937,0.537242802810037,1.21108489280014));
#20877=CARTESIAN_POINT('Ctrl Pts',(0.999433395982306,0.512927734894202,
1.24526606650747));
#20878=CARTESIAN_POINT('Ctrl Pts',(0.984525703911604,0.501969908730509,
1.26352342884146));
#20879=CARTESIAN_POINT('Ctrl Pts',(0.962275025729455,0.493314642657339,
1.28727233489076));
#20880=CARTESIAN_POINT('Ctrl Pts',(0.962275025729455,0.493314642657339,
1.28727233489076));
#20881=CARTESIAN_POINT('Ctrl Pts',(1.18245156164078,0.551233034159898,1.54044293163017));
#20882=CARTESIAN_POINT('Ctrl Pts',(1.38558898119851,0.472718500477254,1.74808806329354));
#20883=CARTESIAN_POINT('Ctrl Pts',(1.57168728440264,0.257771041609407,1.91020772988088));
#20884=CARTESIAN_POINT('Ctrl Pts',(0.979724075862581,0.453542382763444,
1.28727233489076));
#20885=CARTESIAN_POINT('Ctrl Pts',(1.20168985388846,0.502493528317088,1.54044293163017));
#20886=CARTESIAN_POINT('Ctrl Pts',(1.40118801151289,0.416024993050259,1.74808806329354));
#20887=CARTESIAN_POINT('Ctrl Pts',(1.57821854873589,0.194136776962957,1.91020772988088));
#20888=CARTESIAN_POINT('Ctrl Pts',(0.997173125995706,0.413770122869549,
1.28727233489076));
#20889=CARTESIAN_POINT('Ctrl Pts',(1.22092814613614,0.453754022474278,1.54044293163017));
#20890=CARTESIAN_POINT('Ctrl Pts',(1.41678704182728,0.359331485623264,1.74808806329354));
#20891=CARTESIAN_POINT('Ctrl Pts',(1.58474981306913,0.130502512316507,1.91020772988088));
#20892=CARTESIAN_POINT('Ctrl Pts',(1.01462217612883,0.373997862975653,1.28727233489076));
#20893=CARTESIAN_POINT('Ctrl Pts',(1.24016643838382,0.405014516631468,1.54044293163017));
#20894=CARTESIAN_POINT('Ctrl Pts',(1.43238607214167,0.302637978196269,1.74808806329354));
#20895=CARTESIAN_POINT('Ctrl Pts',(1.59128107740238,0.0668682476700567,
1.91020772988088));
#20896=CARTESIAN_POINT('',(1.01462217612883,0.373997862975654,1.28727233489076));
#20897=CARTESIAN_POINT('Ctrl Pts',(1.01462217612883,0.373997862975653,1.28727233489076));
#20898=CARTESIAN_POINT('Ctrl Pts',(1.11493412912611,0.387792676785359,1.39987124007464));
#20899=CARTESIAN_POINT('Ctrl Pts',(1.20865423507634,0.375201374409042,1.50346488650363));
#20900=CARTESIAN_POINT('Ctrl Pts',(1.40394856048621,0.287835131123856,1.715480776583));
#20901=CARTESIAN_POINT('Ctrl Pts',(1.50195515531182,0.198779555753984,1.81902921434248));
#20902=CARTESIAN_POINT('Ctrl Pts',(1.58980227845634,0.0690572297370882,
1.90869858745619));
#20903=CARTESIAN_POINT('Ctrl Pts',(0.962275025729455,0.493314642657339,
1.28727233489076));
#20904=CARTESIAN_POINT('Ctrl Pts',(0.971588210291788,0.473624023308133,
1.28796759655004));
#20905=CARTESIAN_POINT('Ctrl Pts',(0.980617871367766,0.453798845322811,
1.2883190755065));
#20906=CARTESIAN_POINT('Ctrl Pts',(0.989369770455727,0.433840171694363,
1.288319084765));
#20907=CARTESIAN_POINT('Ctrl Pts',(0.9980677061135,0.414004561469663,1.28831909396641));
#20908=CARTESIAN_POINT('Ctrl Pts',(1.00648259836304,0.394057020835195,1.28797193184368));
#20909=CARTESIAN_POINT('Ctrl Pts',(1.01462217612883,0.373997862975653,1.28727233489076));
#20910=CARTESIAN_POINT('Ctrl Pts',(1.01098164380599,0.373486051296587,1.28318517918604));
#20911=CARTESIAN_POINT('Ctrl Pts',(1.23747555342208,0.40602191942841,1.53750926858099));
#20912=CARTESIAN_POINT('Ctrl Pts',(1.43047014156898,0.304465327263434,1.74606924121325));
#20913=CARTESIAN_POINT('Ctrl Pts',(1.58996540824668,0.0688162748016592,
1.90886509708283));
#20914=CARTESIAN_POINT('Ctrl Pts',(1.02865698469238,0.382166213971436,1.26356265747109));
#20915=CARTESIAN_POINT('Ctrl Pts',(1.25921979945503,0.415747810278511,1.51398032870897));
#20916=CARTESIAN_POINT('Ctrl Pts',(1.45578649927554,0.312707553760741,1.71944252353203));
#20917=CARTESIAN_POINT('Ctrl Pts',(1.61866306691266,0.0730554435692883,
1.87974468006743));
#20918=CARTESIAN_POINT('Ctrl Pts',(1.06331677531061,0.391657241669877,1.2281080635226));
#20919=CARTESIAN_POINT('Ctrl Pts',(1.30153367691801,0.425647906592844,1.47146671103428));
#20920=CARTESIAN_POINT('Ctrl Pts',(1.50438827167772,0.318676377131993,1.67103178775815));
#20921=CARTESIAN_POINT('Ctrl Pts',(1.67188067012362,0.0707311879561156,
1.82679988540377));
#20922=CARTESIAN_POINT('Ctrl Pts',(1.13146507111568,0.386793101125271,1.16783895333641));
#20923=CARTESIAN_POINT('Ctrl Pts',(1.38370624635607,0.41672899565074,1.39917869757247));
#20924=CARTESIAN_POINT('Ctrl Pts',(1.59505828371836,0.298796521842133,1.5889289477722));
#20925=CARTESIAN_POINT('Ctrl Pts',(1.76565888855501,0.032993380760367,1.73699566095832));
#20926=CARTESIAN_POINT('Ctrl Pts',(1.18300585575676,0.373540819382844,1.12609865864079));
#20927=CARTESIAN_POINT('Ctrl Pts',(1.44530457310529,0.398429005793492,1.34921513358856));
#20928=CARTESIAN_POINT('Ctrl Pts',(1.66164003747217,0.270901963247261,1.53217466057835));
#20929=CARTESIAN_POINT('Ctrl Pts',(1.83206393610153,-0.00890514499182499,
1.67498164591399));
#20930=CARTESIAN_POINT('Ctrl Pts',(1.21448591285885,0.362468171451202,1.10179959977345));
#20931=CARTESIAN_POINT('Ctrl Pts',(1.48279448162748,0.383640993960512,1.32012924726704));
#20932=CARTESIAN_POINT('Ctrl Pts',(1.70171239168859,0.249943984819042,1.49916808705051));
#20933=CARTESIAN_POINT('Ctrl Pts',(1.87123964304218,-0.0386228559732111,
1.63891611912387));
#20934=CARTESIAN_POINT('',(1.20742290720348,0.364905277844141,1.10727038327973));
#20935=CARTESIAN_POINT('Ctrl Pts',(1.20742290720348,0.364905277844141,1.10727038327973));
#20936=CARTESIAN_POINT('Ctrl Pts',(1.2881015973139,0.372446289646659,1.17697999301248));
#20937=CARTESIAN_POINT('Ctrl Pts',(1.3704559615559,0.364817298041905,1.24430717677952));
#20938=CARTESIAN_POINT('Ctrl Pts',(1.53992597283256,0.308173273864794,1.37795460947453));
#20939=CARTESIAN_POINT('Ctrl Pts',(1.62124173855644,0.257956459417363,1.43952296396722));
#20940=CARTESIAN_POINT('Ctrl Pts',(1.75990988600071,0.127450637982172,1.547796704752));
#20941=CARTESIAN_POINT('Ctrl Pts',(1.81609416413933,0.0535283678677367,
1.5933649555937));
#20942=CARTESIAN_POINT('Ctrl Pts',(1.86363850813291,-0.0276890267571701,
1.63615580822897));
#20943=CARTESIAN_POINT('Ctrl Pts',(1.01462217612883,0.373997862975653,1.28727233489076));
#20944=CARTESIAN_POINT('Ctrl Pts',(1.0440064014209,0.388393237732341,1.25472274024233));
#20945=CARTESIAN_POINT('Ctrl Pts',(1.07127228109912,0.391823670549181,1.22803799031345));
#20946=CARTESIAN_POINT('Ctrl Pts',(1.13395503796013,0.386137988414013,1.1707920398715));
#20947=CARTESIAN_POINT('Ctrl Pts',(1.16846630960532,0.378867340059468,1.14052203161166));
#20948=CARTESIAN_POINT('Ctrl Pts',(1.20742290720348,0.364905277844141,1.10727038327973));
#20949=CARTESIAN_POINT('Ctrl Pts',(1.23578335387376,0.281756991007075,1.1017328493151));
#20950=CARTESIAN_POINT('Ctrl Pts',(1.50493278576872,0.285293785520307,1.3200756344191));
#20951=CARTESIAN_POINT('Ctrl Pts',(1.71461214828353,0.137495264840185,1.49912049044759));
#20952=CARTESIAN_POINT('Ctrl Pts',(1.86482144141819,-0.16163857103329,1.63886741740055));
#20953=CARTESIAN_POINT('Ctrl Pts',(1.20648752589176,0.248240087990173,1.13414277848452));
#20954=CARTESIAN_POINT('Ctrl Pts',(1.46811671142948,0.246204407588735,1.35885799576156));
#20955=CARTESIAN_POINT('Ctrl Pts',(1.66875380764494,0.0982540365453173,
1.54315303441877));
#20956=CARTESIAN_POINT('Ctrl Pts',(1.80862652874333,-0.195476545731338,
1.68697274180732));
#20957=CARTESIAN_POINT('Ctrl Pts',(1.16364558145094,0.2085271896007,1.1806131496188));
#20958=CARTESIAN_POINT('Ctrl Pts',(1.41464853624076,0.20010880260165,1.41450373020722));
#20959=CARTESIAN_POINT('Ctrl Pts',(1.60356331755514,0.053262188267234,1.60633610108347));
#20960=CARTESIAN_POINT('Ctrl Pts',(1.73053166984717,-0.232035965773771,
1.75602333097544));
#20961=CARTESIAN_POINT('Ctrl Pts',(1.10574232216633,0.177813888094452,1.24113368360636));
#20962=CARTESIAN_POINT('Ctrl Pts',(1.34323970181785,0.165512243823414,1.48714102989093));
#20963=CARTESIAN_POINT('Ctrl Pts',(1.51964328480289,0.0231812731496048,
1.68887271819552));
#20964=CARTESIAN_POINT('Ctrl Pts',(1.63495516880573,-0.249170413362414,
1.84633185797667));
#20965=CARTESIAN_POINT('Ctrl Pts',(1.07870022090367,0.172859970247478,1.26846296103996));
#20966=CARTESIAN_POINT('Ctrl Pts',(1.31037084404559,0.160752258036383,1.51988605935311));
#20967=CARTESIAN_POINT('Ctrl Pts',(1.48224938444032,0.0218314126094617,
1.72614171343828));
#20968=CARTESIAN_POINT('Ctrl Pts',(1.59461215150753,-0.243918395495164,
1.88707489423908));
#20969=CARTESIAN_POINT('Ctrl Pts',(1.06394999292458,0.172008888578299,1.28318566992362));
#20970=CARTESIAN_POINT('Ctrl Pts',(1.29249985168945,0.160360824547434,1.5375404757467));
#20971=CARTESIAN_POINT('Ctrl Pts',(1.46236429518571,0.0235398295887289,
1.74612008846831));
#20972=CARTESIAN_POINT('Ctrl Pts',(1.57354332341336,-0.238454096297817,
1.90892450808844));
#20973=CARTESIAN_POINT('',(1.06762054184321,0.171810769270086,1.28727233489076));
#20974=CARTESIAN_POINT('Ctrl Pts',(1.06762054184321,0.171810769270086,1.28727233489076));
#20975=CARTESIAN_POINT('Ctrl Pts',(1.16871252149279,0.166049132983329,1.39987124007464));
#20976=CARTESIAN_POINT('Ctrl Pts',(1.25825944116939,0.135662485730195,1.50346488650363));
#20977=CARTESIAN_POINT('Ctrl Pts',(1.43309732687145,0.0123561690781439,
1.715480776583));
#20978=CARTESIAN_POINT('Ctrl Pts',(1.51213990150266,-0.093890993375447,
1.81902921434248));
#20979=CARTESIAN_POINT('Ctrl Pts',(1.57338902476662,-0.238090659850088,
1.90869858745619));
#20980=CARTESIAN_POINT('',(1.23077165948193,0.27609248605185,1.10727038327973));
#20981=CARTESIAN_POINT('Ctrl Pts',(1.23077165948193,0.27609248605185,1.10727038327973));
#20982=CARTESIAN_POINT('Ctrl Pts',(1.21397173814614,0.25604578597751,1.12805083925445));
#20983=CARTESIAN_POINT('Ctrl Pts',(1.19436482287741,0.235667011409686,1.15131250789252));
#20984=CARTESIAN_POINT('Ctrl Pts',(1.15844075168677,0.206554607000144,1.1919477734957));
#20985=CARTESIAN_POINT('Ctrl Pts',(1.14116749104432,0.19410271785776,1.2110848928));
#20986=CARTESIAN_POINT('Ctrl Pts',(1.10902103082114,0.178981360555533,1.24526606650682));
#20987=CARTESIAN_POINT('Ctrl Pts',(1.09145681862835,0.173166578774623,1.26352342884088));
#20988=CARTESIAN_POINT('Ctrl Pts',(1.06762054184321,0.171810769270086,1.28727233489076));
#20989=CARTESIAN_POINT('Ctrl Pts',(1.85754313061971,-0.153129647965883,
1.63615580822897));
#20990=CARTESIAN_POINT('Ctrl Pts',(1.81335940151627,-0.0607713534907822,
1.59083969670469));
#20991=CARTESIAN_POINT('Ctrl Pts',(1.75708539039456,0.0223614442500402,
1.54129005514746));
#20992=CARTESIAN_POINT('Ctrl Pts',(1.61733286423933,0.159600739735627,1.42521036359322));
#20993=CARTESIAN_POINT('Ctrl Pts',(1.53789592166465,0.208550308549111,1.36183966503053));
#20994=CARTESIAN_POINT('Ctrl Pts',(1.37907079095174,0.264206681902339,1.23219371736399));
#20995=CARTESIAN_POINT('Ctrl Pts',(1.30454791379682,0.275306576910198,1.17031259812848));
#20996=CARTESIAN_POINT('Ctrl Pts',(1.23077165948193,0.27609248605185,1.10727038327973));
#20997=CARTESIAN_POINT('Ctrl Pts',(1.06762054184321,0.171810769270086,1.28727233489076));
#20998=CARTESIAN_POINT('Ctrl Pts',(1.29491863831812,0.158856141562724,1.54044293163017));
#20999=CARTESIAN_POINT('Ctrl Pts',(1.46385147967852,0.0214114678431584,
1.74808806329354));
#21000=CARTESIAN_POINT('Ctrl Pts',(1.5744190659244,-0.240523251888611,1.91020772988088));
#21001=CARTESIAN_POINT('Ctrl Pts',(1.07192527046357,0.128593049303376,1.28727233489076));
#21002=CARTESIAN_POINT('Ctrl Pts',(1.2981540059198,0.106557157682628,1.54044293163017));
#21003=CARTESIAN_POINT('Ctrl Pts',(1.46116778184124,-0.0373276272898292,
1.74808806329354));
#21004=CARTESIAN_POINT('Ctrl Pts',(1.56096659822788,-0.303061305613996,
1.91020772988088));
#21005=CARTESIAN_POINT('Ctrl Pts',(1.07622999908393,0.0853753293366667,
1.28727233489076));
#21006=CARTESIAN_POINT('Ctrl Pts',(1.30138937352148,0.0542581738025322,
1.54044293163017));
#21007=CARTESIAN_POINT('Ctrl Pts',(1.45848408400396,-0.0960667224228172,
1.74808806329354));
#21008=CARTESIAN_POINT('Ctrl Pts',(1.54751413053135,-0.365599359339381,
1.91020772988088));
#21009=CARTESIAN_POINT('Ctrl Pts',(1.08053472770428,0.042157609369957,1.28727233489076));
#21010=CARTESIAN_POINT('Ctrl Pts',(1.30462474112317,0.00195918992243627,
1.54044293163017));
#21011=CARTESIAN_POINT('Ctrl Pts',(1.45580038616668,-0.154805817555805,
1.74808806329354));
#21012=CARTESIAN_POINT('Ctrl Pts',(1.53406166283483,-0.428137413064766,
1.91020772988088));
#21013=CARTESIAN_POINT('',(1.08053472770428,0.042157609369957,1.28727233489076));
#21014=CARTESIAN_POINT('Ctrl Pts',(1.08053472770428,0.042157609369957,1.28727233489076));
#21015=CARTESIAN_POINT('Ctrl Pts',(1.18019989616608,0.024279158719655,1.39987124007464));
#21016=CARTESIAN_POINT('Ctrl Pts',(1.26544208722232,-0.0166569869072256,
1.50346488650363));
#21017=CARTESIAN_POINT('Ctrl Pts',(1.42418037408903,-0.16009648734447,1.715480776583));
#21018=CARTESIAN_POINT('Ctrl Pts',(1.48987049850469,-0.275079075974333,
1.81902921434248));
#21019=CARTESIAN_POINT('Ctrl Pts',(1.53333167412,-0.425598593400271,1.90869858745619));
#21020=CARTESIAN_POINT('Ctrl Pts',(1.06762054184321,0.171810769270086,1.28727233489076));
#21021=CARTESIAN_POINT('Ctrl Pts',(1.0703931707,0.150205945126616,1.28796759655004));
#21022=CARTESIAN_POINT('Ctrl Pts',(1.07285457179227,0.128560761691046,1.2883190755065));
#21023=CARTESIAN_POINT('Ctrl Pts',(1.07501055311346,0.106874449528872,1.288319084765));
#21024=CARTESIAN_POINT('Ctrl Pts',(1.07715324084587,0.0853218532357679,
1.28831909396641));
#21025=CARTESIAN_POINT('Ctrl Pts',(1.07899214990168,0.0637502700203708,
1.28797193184368));
#21026=CARTESIAN_POINT('Ctrl Pts',(1.08053472770428,0.0421576093699569,
1.28727233489076));
#21027=CARTESIAN_POINT('Ctrl Pts',(1.07691421720911,0.0427958338937931,
1.28318517918604));
#21028=CARTESIAN_POINT('Ctrl Pts',(1.30237686203014,0.00374881610008822,
1.53750926858099));
#21029=CARTESIAN_POINT('Ctrl Pts',(1.45454290982716,-0.15247585021093,1.74606924121326));
#21030=CARTESIAN_POINT('Ctrl Pts',(1.53341236060018,-0.425878165039262,
1.90886509708284));
#21031=CARTESIAN_POINT('Ctrl Pts',(1.091545040475,0.0448924758011831,1.26845681306972));
#21032=CARTESIAN_POINT('Ctrl Pts',(1.32014932750452,0.0055908047641015,
1.51984840181958));
#21033=CARTESIAN_POINT('Ctrl Pts',(1.4745930125769,-0.152438895007652,1.72608377212012));
#21034=CARTESIAN_POINT('Ctrl Pts',(1.55488138991364,-0.429508274607607,
1.88700775532559));
#21035=CARTESIAN_POINT('Ctrl Pts',(1.11904054473513,0.0454099470705955,
1.24111941924412));
#21036=CARTESIAN_POINT('Ctrl Pts',(1.35337649424567,0.00503268467650712,
1.48709402322589));
#21037=CARTESIAN_POINT('Ctrl Pts',(1.51165038249934,-0.157175625948469,
1.68880469124906));
#21038=CARTESIAN_POINT('Ctrl Pts',(1.59385438982847,-0.441219201568131,
1.84625359892919));
#21039=CARTESIAN_POINT('Ctrl Pts',(1.18191630764681,0.026799925001142,1.18057686266081));
#21040=CARTESIAN_POINT('Ctrl Pts',(1.42860644524987,-0.0203022432084509,
1.41443159040039));
#21041=CARTESIAN_POINT('Ctrl Pts',(1.59265822923791,-0.19450578395595,1.60624053738541));
#21042=CARTESIAN_POINT('Ctrl Pts',(1.6740871562873,-0.495974904441967,1.75591502454111));
#21043=CARTESIAN_POINT('Ctrl Pts',(1.23181557314521,-0.00363238016698347,
1.1340877844534));
#21044=CARTESIAN_POINT('Ctrl Pts',(1.48747160844964,-0.0593232212680496,
1.35876508657128));
#21045=CARTESIAN_POINT('Ctrl Pts',(1.65371551508434,-0.245130498049609,
1.54303391436826));
#21046=CARTESIAN_POINT('Ctrl Pts',(1.73041945202572,-0.561310568731033,
1.68683916414419));
#21047=CARTESIAN_POINT('Ctrl Pts',(1.26719829440569,-0.0306796703370956,
1.10166698368801));
#21048=CARTESIAN_POINT('Ctrl Pts',(1.52894260490193,-0.0934843164788936,
1.3199705116299));
#21049=CARTESIAN_POINT('Ctrl Pts',(1.69583409006837,-0.288323673548516,
1.49898794576061));
#21050=CARTESIAN_POINT('Ctrl Pts',(1.76787274990501,-0.615197741545964,
1.63871928608014));
#21051=CARTESIAN_POINT('Ctrl Pts',(1.08053472770428,0.042157609369957,1.28727233489076));
#21052=CARTESIAN_POINT('Ctrl Pts',(1.1129292020849,0.0467681993550386,1.25472274024223));
#21053=CARTESIAN_POINT('Ctrl Pts',(1.13992065666396,0.0416051146519737,
1.22803799031325));
#21054=CARTESIAN_POINT('Ctrl Pts',(1.19777852863138,0.016827672483465,1.1707920398715));
#21055=CARTESIAN_POINT('Ctrl Pts',(1.22835394451345,-0.000751694447614519,
1.14052203161171));
#21056=CARTESIAN_POINT('Ctrl Pts',(1.26108935601086,-0.026068655399315,
1.10727038327973));
#21057=CARTESIAN_POINT('Origin',(0.,0.,1.38794976669063));
#21058=CARTESIAN_POINT('',(-0.7,-8.57252759403147E-17,1.66862915010152));
#21059=CARTESIAN_POINT('Origin',(0.,0.,1.66862915010152));
#21060=CARTESIAN_POINT('',(-0.980679383410898,-1.20098586788396E-16,1.38794976669063));
#21061=CARTESIAN_POINT('Origin',(0.,0.,1.10727038327973));
#21062=CARTESIAN_POINT('Origin',(0.,0.,1.37171309575435));
#21063=CARTESIAN_POINT('Origin',(0.541,0.,2.6));
#21064=CARTESIAN_POINT('',(-0.541,-6.62533918338718E-17,2.6));
#21065=CARTESIAN_POINT('Origin',(0.,0.,2.6));
#21066=CARTESIAN_POINT('Origin',(0.,0.,2.58));
#21067=CARTESIAN_POINT('',(-0.501,-6.13548046372824E-17,2.56));
#21068=CARTESIAN_POINT('',(-0.521,-6.38040982355771E-17,2.58));
#21069=CARTESIAN_POINT('Origin',(0.,0.,2.56));
#21070=CARTESIAN_POINT('Origin',(0.,0.,2.13431457505076));
#21071=CARTESIAN_POINT('',(-0.501,-6.13548046372824E-17,1.70862915010152));
#21072=CARTESIAN_POINT('',(-0.501,-6.13548046372824E-17,2.13431457505076));
#21073=CARTESIAN_POINT('Origin',(0.,0.,1.70862915010152));
#21074=CARTESIAN_POINT('Origin',(0.,0.,1.68862915010152));
#21075=CARTESIAN_POINT('',(-0.541,-6.62533918338718E-17,1.66862915010152));
#21076=CARTESIAN_POINT('',(-0.521,-6.38040982355771E-17,1.68862915010152));
#21077=CARTESIAN_POINT('Origin',(0.,0.,1.66862915010152));
#21078=CARTESIAN_POINT('Origin',(0.7,0.,1.66862915010152));
#31615=UNCERTAINTY_MEASURE_WITH_UNIT(LENGTH_MEASURE(0.001),#31639,
'DISTANCE_ACCURACY_VALUE',
'Maximum model space distance between geometric entities at asserted c
onnectivities');
#31625=UNCERTAINTY_MEASURE_WITH_UNIT(LENGTH_MEASURE(0.001),#31639,
'DISTANCE_ACCURACY_VALUE',
'Maximum model space distance between geometric entities at asserted c
onnectivities');
#31628=(
GEOMETRIC_REPRESENTATION_CONTEXT(3)
GLOBAL_UNCERTAINTY_ASSIGNED_CONTEXT((#31615))
GLOBAL_UNIT_ASSIGNED_CONTEXT((#31639,#31641,#31642))
REPRESENTATION_CONTEXT('','3D')
);
#31638=(
GEOMETRIC_REPRESENTATION_CONTEXT(3)
GLOBAL_UNCERTAINTY_ASSIGNED_CONTEXT((#31625))
GLOBAL_UNIT_ASSIGNED_CONTEXT((#31639,#31641,#31642))
REPRESENTATION_CONTEXT('','3D')
);
#31639=(
LENGTH_UNIT()
NAMED_UNIT(*)
SI_UNIT(.CENTI.,.METRE.)
);
#31641=(
NAMED_UNIT(*)
PLANE_ANGLE_UNIT()
SI_UNIT($,.RADIAN.)
);
#31642=(
NAMED_UNIT(*)
SI_UNIT($,.STERADIAN.)
SOLID_ANGLE_UNIT()
);
#31645=SHAPE_DEFINITION_REPRESENTATION(#31657,#31706);
#31657=PRODUCT_DEFINITION_SHAPE('',$,#31719);
#31706=SHAPE_REPRESENTATION('',(#12776),#31628);
#31716=PRODUCT_DEFINITION_CONTEXT('part definition',#31754,'design');
#31719=PRODUCT_DEFINITION('2026-10-22-02-42-12-427',
'03_Spiral_Bevel_Pinion_m1.75_z20_LH_Input',#31731,#31716);
#31731=PRODUCT_DEFINITION_FORMATION('',$,#31758);
#31754=APPLICATION_CONTEXT(
'Core Data for Automotive Mechanical Design Process');
#31755=PRODUCT_CONTEXT('part definition',#31754,'mechanical');
#31758=PRODUCT('2026-10-22-02-42-12-427',
'03_Spiral_Bevel_Pinion_m1.75_z20_LH_Input',$,(#31755));
#31817=COLOUR_RGB('Sky Blue',0.24,0.69,0.87);
#31818=FILL_AREA_STYLE_COLOUR('',#31817);
#31819=FILL_AREA_STYLE('',(#31818));
#31820=SURFACE_STYLE_FILL_AREA(#31819);
#31821=SURFACE_SIDE_STYLE('',(#31820));
#31822=SURFACE_STYLE_USAGE(.BOTH.,#31821);
#31823=PRESENTATION_STYLE_ASSIGNMENT((#31822));
ENDSEC;
END-ISO-10303-21;
